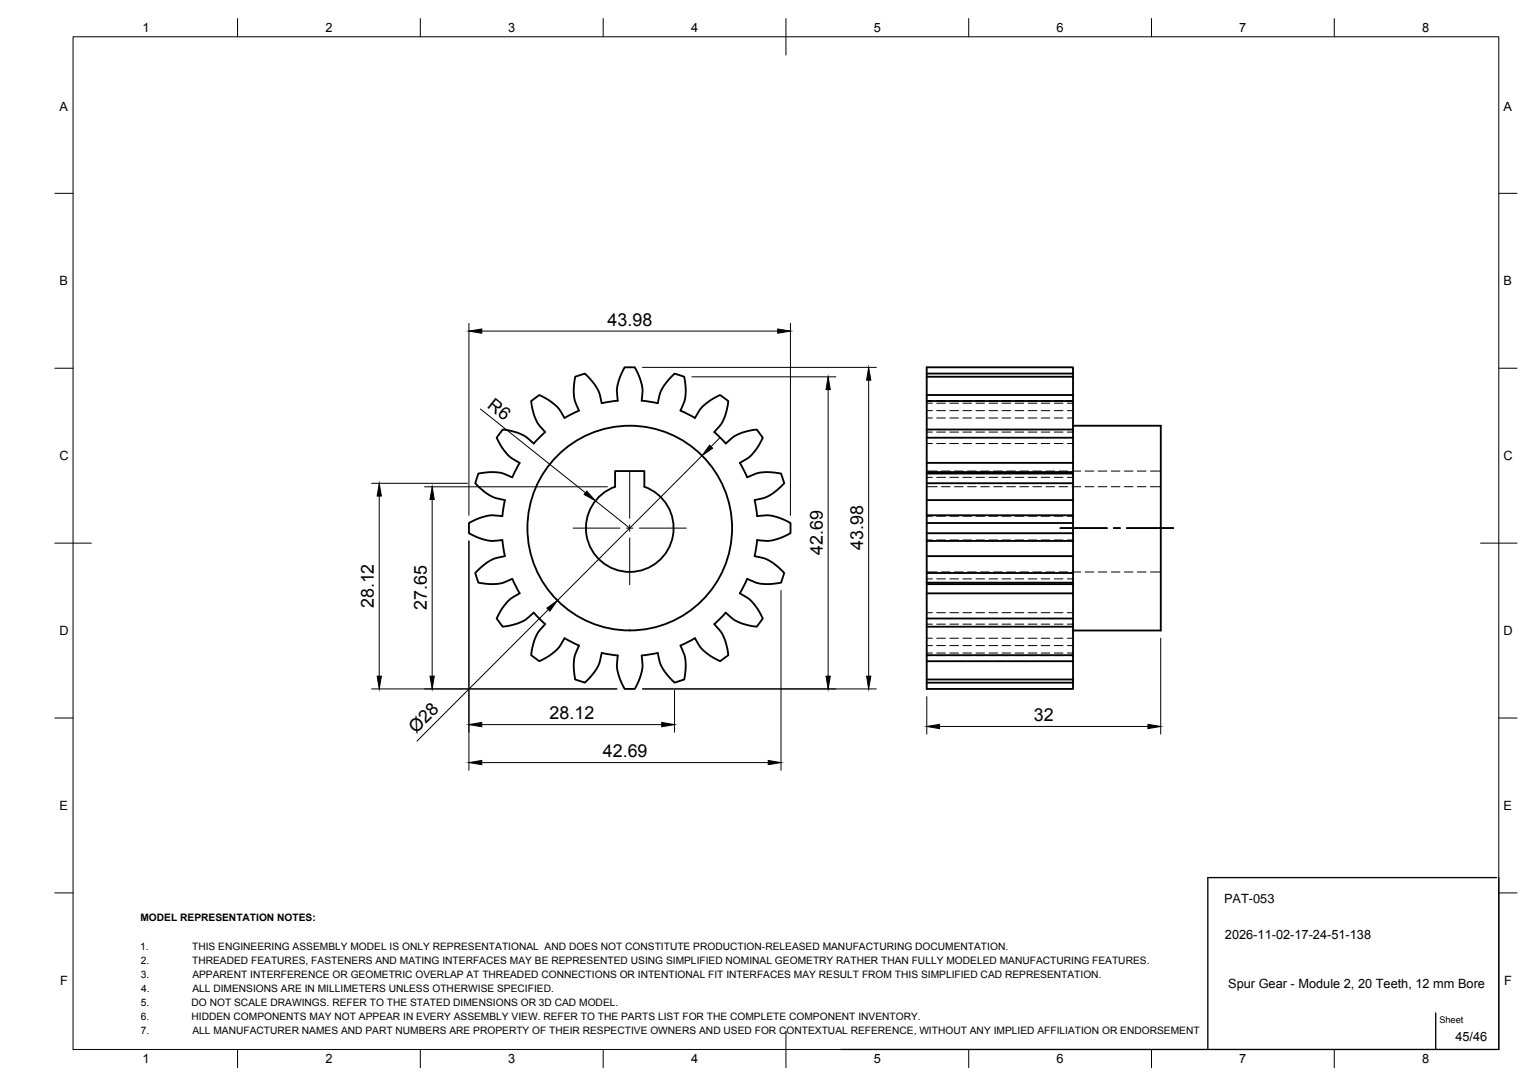
ISO-10303-21;
HEADER;
/* Generated by software containing ST-Developer
 * from STEP Tools, Inc. (www.steptools.com) 
 */

FILE_DESCRIPTION(
/* description */ ('Hand-operated arbor press'),
/* implementation_level */ '2;1');

FILE_NAME(
/* name */ 'Spur Gear - Module 2, 20 Teeth, 12 mm Bore.step',
/* time_stamp */ '2026-10-28T03:25:25-07:00',
/* author */ (''),
/* organization */ (''),
/* preprocessor_version */ 'ST-DEVELOPER v20.2',
/* originating_system */ 'Autodesk Translation Framework v15.17.0.0',
/* authorisation */ '');

FILE_SCHEMA (('AUTOMOTIVE_DESIGN { 1 0 10303 214 3 1 1 }'));
ENDSEC;

DATA;
#10=MECHANICAL_DESIGN_GEOMETRIC_PRESENTATION_REPRESENTATION('',(#630),#32751);
#11=(
BOUNDED_SURFACE()
B_SPLINE_SURFACE(5,1,((#23774,#23775),(#23776,#23777),(#23778,#23779),(#23780,
#23781),(#23782,#23783),(#23784,#23785),(#23786,#23787),(#23788,#23789),
(#23790,#23791),(#23792,#23793),(#23794,#23795),(#23796,#23797),(#23798,
#23799),(#23800,#23801),(#23802,#23803),(#23804,#23805),(#23806,#23807),
(#23808,#23809),(#23810,#23811),(#23812,#23813),(#23814,#23815),(#23816,
#23817),(#23818,#23819),(#23820,#23821),(#23822,#23823),(#23824,#23825),
(#23826,#23827),(#23828,#23829),(#23830,#23831),(#23832,#23833),(#23834,
#23835),(#23836,#23837),(#23838,#23839),(#23840,#23841),(#23842,#23843),
(#23844,#23845),(#23846,#23847),(#23848,#23849),(#23850,#23851),(#23852,
#23853),(#23854,#23855),(#23856,#23857),(#23858,#23859),(#23860,#23861),
(#23862,#23863),(#23864,#23865),(#23866,#23867),(#23868,#23869),(#23870,
#23871),(#23872,#23873),(#23874,#23875),(#23876,#23877),(#23878,#23879),
(#23880,#23881),(#23882,#23883),(#23884,#23885),(#23886,#23887),(#23888,
#23889),(#23890,#23891),(#23892,#23893),(#23894,#23895),(#23896,#23897),
(#23898,#23899),(#23900,#23901),(#23902,#23903),(#23904,#23905),(#23906,
#23907),(#23908,#23909),(#23910,#23911),(#23912,#23913)),.UNSPECIFIED.,
 .F.,.F.,.F.)
B_SPLINE_SURFACE_WITH_KNOTS((6,1,1,1,1,1,1,1,1,1,1,1,1,1,1,1,1,1,1,1,1,
1,1,1,1,1,1,1,1,1,1,1,1,1,1,1,1,1,1,1,1,1,1,1,1,1,1,1,1,1,1,1,1,1,1,1,1,
1,1,1,1,1,1,1,1,6),(2,2),(-1.,-0.984615384615383,-0.969230769230768,-0.953846153846152,
-0.938461538461537,-0.923076923076922,-0.907692307692306,-0.892307692307691,
-0.876923076923076,-0.86153846153846,-0.846153846153845,-0.83076923076923,
-0.815384615384614,-0.799999999999999,-0.784615384615384,-0.769230769230768,
-0.753846153846153,-0.738461538461538,-0.723076923076922,-0.707692307692307,
-0.692307692307692,-0.676923076923076,-0.661538461538461,-0.646153846153846,
-0.63076923076923,-0.615384615384615,-0.6,-0.584615384615384,-0.569230769230769,
-0.553846153846154,-0.538461538461538,-0.523076923076923,-0.507692307692308,
-0.492307692307692,-0.476923076923077,-0.461538461538462,-0.446153846153846,
-0.430769230769231,-0.415384615384615,-0.4,-0.384615384615385,-0.369230769230769,
-0.353846153846154,-0.338461538461538,-0.323076923076923,-0.307692307692308,
-0.292307692307692,-0.276923076923077,-0.261538461538462,-0.246153846153846,
-0.230769230769231,-0.215384615384615,-0.2,-0.184615384615385,-0.169230769230769,
-0.153846153846154,-0.138461538461538,-0.123076923076923,-0.107692307692308,
-0.0923076923076923,-0.0769230769230769,-0.0615384615384615,-0.0461538461538462,
-0.0307692307692308,-0.0153846153846154,0.),(-1.,1.),.UNSPECIFIED.)
GEOMETRIC_REPRESENTATION_ITEM()
RATIONAL_B_SPLINE_SURFACE(((1.,1.),(1.,1.),(1.,1.),(1.,1.),(1.,1.),(1.,
1.),(1.,1.),(1.,1.),(1.,1.),(1.,1.),(1.,1.),(1.,1.),(1.,1.),(1.,1.),(1.,
1.),(1.,1.),(1.,1.),(1.,1.),(1.,1.),(1.,1.),(1.,1.),(1.,1.),(1.,1.),(1.,
1.),(1.,1.),(1.,1.),(1.,1.),(1.,1.),(1.,1.),(1.,1.),(1.,1.),(1.,1.),(1.,
1.),(1.,1.),(1.,1.),(1.,1.),(1.,1.),(1.,1.),(1.,1.),(1.,1.),(1.,1.),(1.,
1.),(1.,1.),(1.,1.),(1.,1.),(1.,1.),(1.,1.),(1.,1.),(1.,1.),(1.,1.),(1.,
1.),(1.,1.),(1.,1.),(1.,1.),(1.,1.),(1.,1.),(1.,1.),(1.,1.),(1.,1.),(1.,
1.),(1.,1.),(1.,1.),(1.,1.),(1.,1.),(1.,1.),(1.,1.),(1.,1.),(1.,1.),(1.,
1.),(1.,1.)))
REPRESENTATION_ITEM('')
SURFACE()
);
#12=(
BOUNDED_SURFACE()
B_SPLINE_SURFACE(5,1,((#23992,#23993),(#23994,#23995),(#23996,#23997),(#23998,
#23999),(#24000,#24001),(#24002,#24003),(#24004,#24005),(#24006,#24007),
(#24008,#24009),(#24010,#24011),(#24012,#24013),(#24014,#24015),(#24016,
#24017),(#24018,#24019),(#24020,#24021),(#24022,#24023),(#24024,#24025),
(#24026,#24027),(#24028,#24029),(#24030,#24031),(#24032,#24033),(#24034,
#24035),(#24036,#24037),(#24038,#24039),(#24040,#24041),(#24042,#24043),
(#24044,#24045),(#24046,#24047),(#24048,#24049),(#24050,#24051),(#24052,
#24053),(#24054,#24055),(#24056,#24057),(#24058,#24059),(#24060,#24061),
(#24062,#24063),(#24064,#24065),(#24066,#24067),(#24068,#24069),(#24070,
#24071),(#24072,#24073),(#24074,#24075),(#24076,#24077),(#24078,#24079),
(#24080,#24081),(#24082,#24083),(#24084,#24085),(#24086,#24087),(#24088,
#24089),(#24090,#24091),(#24092,#24093),(#24094,#24095),(#24096,#24097),
(#24098,#24099),(#24100,#24101),(#24102,#24103),(#24104,#24105),(#24106,
#24107),(#24108,#24109),(#24110,#24111),(#24112,#24113),(#24114,#24115),
(#24116,#24117),(#24118,#24119),(#24120,#24121),(#24122,#24123),(#24124,
#24125),(#24126,#24127),(#24128,#24129),(#24130,#24131)),.UNSPECIFIED.,
 .F.,.F.,.F.)
B_SPLINE_SURFACE_WITH_KNOTS((6,1,1,1,1,1,1,1,1,1,1,1,1,1,1,1,1,1,1,1,1,
1,1,1,1,1,1,1,1,1,1,1,1,1,1,1,1,1,1,1,1,1,1,1,1,1,1,1,1,1,1,1,1,1,1,1,1,
1,1,1,1,1,1,1,1,6),(2,2),(-1.,-0.984615384615383,-0.969230769230768,-0.953846153846152,
-0.938461538461537,-0.923076923076922,-0.907692307692306,-0.892307692307691,
-0.876923076923076,-0.86153846153846,-0.846153846153845,-0.83076923076923,
-0.815384615384614,-0.799999999999999,-0.784615384615384,-0.769230769230768,
-0.753846153846153,-0.738461538461538,-0.723076923076922,-0.707692307692307,
-0.692307692307692,-0.676923076923076,-0.661538461538461,-0.646153846153846,
-0.63076923076923,-0.615384615384615,-0.6,-0.584615384615384,-0.569230769230769,
-0.553846153846154,-0.538461538461538,-0.523076923076923,-0.507692307692308,
-0.492307692307692,-0.476923076923077,-0.461538461538462,-0.446153846153846,
-0.430769230769231,-0.415384615384615,-0.4,-0.384615384615385,-0.369230769230769,
-0.353846153846154,-0.338461538461538,-0.323076923076923,-0.307692307692308,
-0.292307692307692,-0.276923076923077,-0.261538461538462,-0.246153846153846,
-0.230769230769231,-0.215384615384615,-0.2,-0.184615384615385,-0.169230769230769,
-0.153846153846154,-0.138461538461538,-0.123076923076923,-0.107692307692308,
-0.0923076923076923,-0.0769230769230769,-0.0615384615384615,-0.0461538461538462,
-0.0307692307692308,-0.0153846153846154,0.),(-1.,1.),.UNSPECIFIED.)
GEOMETRIC_REPRESENTATION_ITEM()
RATIONAL_B_SPLINE_SURFACE(((1.,1.),(1.,1.),(1.,1.),(1.,1.),(1.,1.),(1.,
1.),(1.,1.),(1.,1.),(1.,1.),(1.,1.),(1.,1.),(1.,1.),(1.,1.),(1.,1.),(1.,
1.),(1.,1.),(1.,1.),(1.,1.),(1.,1.),(1.,1.),(1.,1.),(1.,1.),(1.,1.),(1.,
1.),(1.,1.),(1.,1.),(1.,1.),(1.,1.),(1.,1.),(1.,1.),(1.,1.),(1.,1.),(1.,
1.),(1.,1.),(1.,1.),(1.,1.),(1.,1.),(1.,1.),(1.,1.),(1.,1.),(1.,1.),(1.,
1.),(1.,1.),(1.,1.),(1.,1.),(1.,1.),(1.,1.),(1.,1.),(1.,1.),(1.,1.),(1.,
1.),(1.,1.),(1.,1.),(1.,1.),(1.,1.),(1.,1.),(1.,1.),(1.,1.),(1.,1.),(1.,
1.),(1.,1.),(1.,1.),(1.,1.),(1.,1.),(1.,1.),(1.,1.),(1.,1.),(1.,1.),(1.,
1.),(1.,1.)))
REPRESENTATION_ITEM('')
SURFACE()
);
#13=(
BOUNDED_SURFACE()
B_SPLINE_SURFACE(5,1,((#24208,#24209),(#24210,#24211),(#24212,#24213),(#24214,
#24215),(#24216,#24217),(#24218,#24219),(#24220,#24221),(#24222,#24223),
(#24224,#24225),(#24226,#24227),(#24228,#24229),(#24230,#24231),(#24232,
#24233),(#24234,#24235),(#24236,#24237),(#24238,#24239),(#24240,#24241),
(#24242,#24243),(#24244,#24245),(#24246,#24247),(#24248,#24249),(#24250,
#24251),(#24252,#24253),(#24254,#24255),(#24256,#24257),(#24258,#24259),
(#24260,#24261),(#24262,#24263),(#24264,#24265),(#24266,#24267),(#24268,
#24269),(#24270,#24271),(#24272,#24273),(#24274,#24275),(#24276,#24277),
(#24278,#24279),(#24280,#24281),(#24282,#24283),(#24284,#24285),(#24286,
#24287),(#24288,#24289),(#24290,#24291),(#24292,#24293),(#24294,#24295),
(#24296,#24297),(#24298,#24299),(#24300,#24301),(#24302,#24303),(#24304,
#24305),(#24306,#24307),(#24308,#24309),(#24310,#24311),(#24312,#24313),
(#24314,#24315),(#24316,#24317),(#24318,#24319),(#24320,#24321),(#24322,
#24323),(#24324,#24325),(#24326,#24327),(#24328,#24329),(#24330,#24331),
(#24332,#24333),(#24334,#24335),(#24336,#24337),(#24338,#24339),(#24340,
#24341),(#24342,#24343),(#24344,#24345),(#24346,#24347)),.UNSPECIFIED.,
 .F.,.F.,.F.)
B_SPLINE_SURFACE_WITH_KNOTS((6,1,1,1,1,1,1,1,1,1,1,1,1,1,1,1,1,1,1,1,1,
1,1,1,1,1,1,1,1,1,1,1,1,1,1,1,1,1,1,1,1,1,1,1,1,1,1,1,1,1,1,1,1,1,1,1,1,
1,1,1,1,1,1,1,1,6),(2,2),(-1.,-0.984615384615383,-0.969230769230768,-0.953846153846152,
-0.938461538461537,-0.923076923076922,-0.907692307692306,-0.892307692307691,
-0.876923076923076,-0.86153846153846,-0.846153846153845,-0.83076923076923,
-0.815384615384614,-0.799999999999999,-0.784615384615384,-0.769230769230768,
-0.753846153846153,-0.738461538461538,-0.723076923076922,-0.707692307692307,
-0.692307692307692,-0.676923076923076,-0.661538461538461,-0.646153846153846,
-0.63076923076923,-0.615384615384615,-0.6,-0.584615384615384,-0.569230769230769,
-0.553846153846154,-0.538461538461538,-0.523076923076923,-0.507692307692308,
-0.492307692307692,-0.476923076923077,-0.461538461538462,-0.446153846153846,
-0.430769230769231,-0.415384615384615,-0.4,-0.384615384615385,-0.369230769230769,
-0.353846153846154,-0.338461538461538,-0.323076923076923,-0.307692307692308,
-0.292307692307692,-0.276923076923077,-0.261538461538462,-0.246153846153846,
-0.230769230769231,-0.215384615384615,-0.2,-0.184615384615385,-0.169230769230769,
-0.153846153846154,-0.138461538461538,-0.123076923076923,-0.107692307692308,
-0.0923076923076923,-0.0769230769230769,-0.0615384615384615,-0.0461538461538462,
-0.0307692307692308,-0.0153846153846154,0.),(-1.,1.),.UNSPECIFIED.)
GEOMETRIC_REPRESENTATION_ITEM()
RATIONAL_B_SPLINE_SURFACE(((1.,1.),(1.,1.),(1.,1.),(1.,1.),(1.,1.),(1.,
1.),(1.,1.),(1.,1.),(1.,1.),(1.,1.),(1.,1.),(1.,1.),(1.,1.),(1.,1.),(1.,
1.),(1.,1.),(1.,1.),(1.,1.),(1.,1.),(1.,1.),(1.,1.),(1.,1.),(1.,1.),(1.,
1.),(1.,1.),(1.,1.),(1.,1.),(1.,1.),(1.,1.),(1.,1.),(1.,1.),(1.,1.),(1.,
1.),(1.,1.),(1.,1.),(1.,1.),(1.,1.),(1.,1.),(1.,1.),(1.,1.),(1.,1.),(1.,
1.),(1.,1.),(1.,1.),(1.,1.),(1.,1.),(1.,1.),(1.,1.),(1.,1.),(1.,1.),(1.,
1.),(1.,1.),(1.,1.),(1.,1.),(1.,1.),(1.,1.),(1.,1.),(1.,1.),(1.,1.),(1.,
1.),(1.,1.),(1.,1.),(1.,1.),(1.,1.),(1.,1.),(1.,1.),(1.,1.),(1.,1.),(1.,
1.),(1.,1.)))
REPRESENTATION_ITEM('')
SURFACE()
);
#14=(
BOUNDED_SURFACE()
B_SPLINE_SURFACE(5,1,((#24424,#24425),(#24426,#24427),(#24428,#24429),(#24430,
#24431),(#24432,#24433),(#24434,#24435),(#24436,#24437),(#24438,#24439),
(#24440,#24441),(#24442,#24443),(#24444,#24445),(#24446,#24447),(#24448,
#24449),(#24450,#24451),(#24452,#24453),(#24454,#24455),(#24456,#24457),
(#24458,#24459),(#24460,#24461),(#24462,#24463),(#24464,#24465),(#24466,
#24467),(#24468,#24469),(#24470,#24471),(#24472,#24473),(#24474,#24475),
(#24476,#24477),(#24478,#24479),(#24480,#24481),(#24482,#24483),(#24484,
#24485),(#24486,#24487),(#24488,#24489),(#24490,#24491),(#24492,#24493),
(#24494,#24495),(#24496,#24497),(#24498,#24499),(#24500,#24501),(#24502,
#24503),(#24504,#24505),(#24506,#24507),(#24508,#24509),(#24510,#24511),
(#24512,#24513),(#24514,#24515),(#24516,#24517),(#24518,#24519),(#24520,
#24521),(#24522,#24523),(#24524,#24525),(#24526,#24527),(#24528,#24529),
(#24530,#24531),(#24532,#24533),(#24534,#24535),(#24536,#24537),(#24538,
#24539),(#24540,#24541),(#24542,#24543),(#24544,#24545),(#24546,#24547),
(#24548,#24549),(#24550,#24551),(#24552,#24553),(#24554,#24555),(#24556,
#24557),(#24558,#24559),(#24560,#24561),(#24562,#24563)),.UNSPECIFIED.,
 .F.,.F.,.F.)
B_SPLINE_SURFACE_WITH_KNOTS((6,1,1,1,1,1,1,1,1,1,1,1,1,1,1,1,1,1,1,1,1,
1,1,1,1,1,1,1,1,1,1,1,1,1,1,1,1,1,1,1,1,1,1,1,1,1,1,1,1,1,1,1,1,1,1,1,1,
1,1,1,1,1,1,1,1,6),(2,2),(-1.,-0.984615384615383,-0.969230769230768,-0.953846153846152,
-0.938461538461537,-0.923076923076922,-0.907692307692306,-0.892307692307691,
-0.876923076923076,-0.86153846153846,-0.846153846153845,-0.83076923076923,
-0.815384615384614,-0.799999999999999,-0.784615384615384,-0.769230769230768,
-0.753846153846153,-0.738461538461538,-0.723076923076922,-0.707692307692307,
-0.692307692307692,-0.676923076923076,-0.661538461538461,-0.646153846153846,
-0.63076923076923,-0.615384615384615,-0.6,-0.584615384615384,-0.569230769230769,
-0.553846153846154,-0.538461538461538,-0.523076923076923,-0.507692307692308,
-0.492307692307692,-0.476923076923077,-0.461538461538462,-0.446153846153846,
-0.430769230769231,-0.415384615384615,-0.4,-0.384615384615385,-0.369230769230769,
-0.353846153846154,-0.338461538461538,-0.323076923076923,-0.307692307692308,
-0.292307692307692,-0.276923076923077,-0.261538461538462,-0.246153846153846,
-0.230769230769231,-0.215384615384615,-0.2,-0.184615384615385,-0.169230769230769,
-0.153846153846154,-0.138461538461538,-0.123076923076923,-0.107692307692308,
-0.0923076923076923,-0.0769230769230769,-0.0615384615384615,-0.0461538461538462,
-0.0307692307692308,-0.0153846153846154,0.),(-1.,1.),.UNSPECIFIED.)
GEOMETRIC_REPRESENTATION_ITEM()
RATIONAL_B_SPLINE_SURFACE(((1.,1.),(1.,1.),(1.,1.),(1.,1.),(1.,1.),(1.,
1.),(1.,1.),(1.,1.),(1.,1.),(1.,1.),(1.,1.),(1.,1.),(1.,1.),(1.,1.),(1.,
1.),(1.,1.),(1.,1.),(1.,1.),(1.,1.),(1.,1.),(1.,1.),(1.,1.),(1.,1.),(1.,
1.),(1.,1.),(1.,1.),(1.,1.),(1.,1.),(1.,1.),(1.,1.),(1.,1.),(1.,1.),(1.,
1.),(1.,1.),(1.,1.),(1.,1.),(1.,1.),(1.,1.),(1.,1.),(1.,1.),(1.,1.),(1.,
1.),(1.,1.),(1.,1.),(1.,1.),(1.,1.),(1.,1.),(1.,1.),(1.,1.),(1.,1.),(1.,
1.),(1.,1.),(1.,1.),(1.,1.),(1.,1.),(1.,1.),(1.,1.),(1.,1.),(1.,1.),(1.,
1.),(1.,1.),(1.,1.),(1.,1.),(1.,1.),(1.,1.),(1.,1.),(1.,1.),(1.,1.),(1.,
1.),(1.,1.)))
REPRESENTATION_ITEM('')
SURFACE()
);
#15=(
BOUNDED_SURFACE()
B_SPLINE_SURFACE(5,1,((#24640,#24641),(#24642,#24643),(#24644,#24645),(#24646,
#24647),(#24648,#24649),(#24650,#24651),(#24652,#24653),(#24654,#24655),
(#24656,#24657),(#24658,#24659),(#24660,#24661),(#24662,#24663),(#24664,
#24665),(#24666,#24667),(#24668,#24669),(#24670,#24671),(#24672,#24673),
(#24674,#24675),(#24676,#24677),(#24678,#24679),(#24680,#24681),(#24682,
#24683),(#24684,#24685),(#24686,#24687),(#24688,#24689),(#24690,#24691),
(#24692,#24693),(#24694,#24695),(#24696,#24697),(#24698,#24699),(#24700,
#24701),(#24702,#24703),(#24704,#24705),(#24706,#24707),(#24708,#24709),
(#24710,#24711),(#24712,#24713),(#24714,#24715),(#24716,#24717),(#24718,
#24719),(#24720,#24721),(#24722,#24723),(#24724,#24725),(#24726,#24727),
(#24728,#24729),(#24730,#24731),(#24732,#24733),(#24734,#24735),(#24736,
#24737),(#24738,#24739),(#24740,#24741),(#24742,#24743),(#24744,#24745),
(#24746,#24747),(#24748,#24749),(#24750,#24751),(#24752,#24753),(#24754,
#24755),(#24756,#24757),(#24758,#24759),(#24760,#24761),(#24762,#24763),
(#24764,#24765),(#24766,#24767),(#24768,#24769),(#24770,#24771),(#24772,
#24773),(#24774,#24775),(#24776,#24777),(#24778,#24779)),.UNSPECIFIED.,
 .F.,.F.,.F.)
B_SPLINE_SURFACE_WITH_KNOTS((6,1,1,1,1,1,1,1,1,1,1,1,1,1,1,1,1,1,1,1,1,
1,1,1,1,1,1,1,1,1,1,1,1,1,1,1,1,1,1,1,1,1,1,1,1,1,1,1,1,1,1,1,1,1,1,1,1,
1,1,1,1,1,1,1,1,6),(2,2),(-1.,-0.984615384615383,-0.969230769230768,-0.953846153846152,
-0.938461538461537,-0.923076923076922,-0.907692307692306,-0.892307692307691,
-0.876923076923076,-0.86153846153846,-0.846153846153845,-0.83076923076923,
-0.815384615384614,-0.799999999999999,-0.784615384615384,-0.769230769230768,
-0.753846153846153,-0.738461538461538,-0.723076923076922,-0.707692307692307,
-0.692307692307692,-0.676923076923076,-0.661538461538461,-0.646153846153846,
-0.63076923076923,-0.615384615384615,-0.6,-0.584615384615384,-0.569230769230769,
-0.553846153846154,-0.538461538461538,-0.523076923076923,-0.507692307692308,
-0.492307692307692,-0.476923076923077,-0.461538461538462,-0.446153846153846,
-0.430769230769231,-0.415384615384615,-0.4,-0.384615384615385,-0.369230769230769,
-0.353846153846154,-0.338461538461538,-0.323076923076923,-0.307692307692308,
-0.292307692307692,-0.276923076923077,-0.261538461538462,-0.246153846153846,
-0.230769230769231,-0.215384615384615,-0.2,-0.184615384615385,-0.169230769230769,
-0.153846153846154,-0.138461538461538,-0.123076923076923,-0.107692307692308,
-0.0923076923076923,-0.0769230769230769,-0.0615384615384615,-0.0461538461538462,
-0.0307692307692308,-0.0153846153846154,0.),(-1.,1.),.UNSPECIFIED.)
GEOMETRIC_REPRESENTATION_ITEM()
RATIONAL_B_SPLINE_SURFACE(((1.,1.),(1.,1.),(1.,1.),(1.,1.),(1.,1.),(1.,
1.),(1.,1.),(1.,1.),(1.,1.),(1.,1.),(1.,1.),(1.,1.),(1.,1.),(1.,1.),(1.,
1.),(1.,1.),(1.,1.),(1.,1.),(1.,1.),(1.,1.),(1.,1.),(1.,1.),(1.,1.),(1.,
1.),(1.,1.),(1.,1.),(1.,1.),(1.,1.),(1.,1.),(1.,1.),(1.,1.),(1.,1.),(1.,
1.),(1.,1.),(1.,1.),(1.,1.),(1.,1.),(1.,1.),(1.,1.),(1.,1.),(1.,1.),(1.,
1.),(1.,1.),(1.,1.),(1.,1.),(1.,1.),(1.,1.),(1.,1.),(1.,1.),(1.,1.),(1.,
1.),(1.,1.),(1.,1.),(1.,1.),(1.,1.),(1.,1.),(1.,1.),(1.,1.),(1.,1.),(1.,
1.),(1.,1.),(1.,1.),(1.,1.),(1.,1.),(1.,1.),(1.,1.),(1.,1.),(1.,1.),(1.,
1.),(1.,1.)))
REPRESENTATION_ITEM('')
SURFACE()
);
#16=(
BOUNDED_SURFACE()
B_SPLINE_SURFACE(5,1,((#24856,#24857),(#24858,#24859),(#24860,#24861),(#24862,
#24863),(#24864,#24865),(#24866,#24867),(#24868,#24869),(#24870,#24871),
(#24872,#24873),(#24874,#24875),(#24876,#24877),(#24878,#24879),(#24880,
#24881),(#24882,#24883),(#24884,#24885),(#24886,#24887),(#24888,#24889),
(#24890,#24891),(#24892,#24893),(#24894,#24895),(#24896,#24897),(#24898,
#24899),(#24900,#24901),(#24902,#24903),(#24904,#24905),(#24906,#24907),
(#24908,#24909),(#24910,#24911),(#24912,#24913),(#24914,#24915),(#24916,
#24917),(#24918,#24919),(#24920,#24921),(#24922,#24923),(#24924,#24925),
(#24926,#24927),(#24928,#24929),(#24930,#24931),(#24932,#24933),(#24934,
#24935),(#24936,#24937),(#24938,#24939),(#24940,#24941),(#24942,#24943),
(#24944,#24945),(#24946,#24947),(#24948,#24949),(#24950,#24951),(#24952,
#24953),(#24954,#24955),(#24956,#24957),(#24958,#24959),(#24960,#24961),
(#24962,#24963),(#24964,#24965),(#24966,#24967),(#24968,#24969),(#24970,
#24971),(#24972,#24973),(#24974,#24975),(#24976,#24977),(#24978,#24979),
(#24980,#24981),(#24982,#24983),(#24984,#24985),(#24986,#24987),(#24988,
#24989),(#24990,#24991),(#24992,#24993),(#24994,#24995)),.UNSPECIFIED.,
 .F.,.F.,.F.)
B_SPLINE_SURFACE_WITH_KNOTS((6,1,1,1,1,1,1,1,1,1,1,1,1,1,1,1,1,1,1,1,1,
1,1,1,1,1,1,1,1,1,1,1,1,1,1,1,1,1,1,1,1,1,1,1,1,1,1,1,1,1,1,1,1,1,1,1,1,
1,1,1,1,1,1,1,1,6),(2,2),(-1.,-0.984615384615383,-0.969230769230768,-0.953846153846152,
-0.938461538461537,-0.923076923076922,-0.907692307692306,-0.892307692307691,
-0.876923076923076,-0.86153846153846,-0.846153846153845,-0.83076923076923,
-0.815384615384614,-0.799999999999999,-0.784615384615384,-0.769230769230768,
-0.753846153846153,-0.738461538461538,-0.723076923076922,-0.707692307692307,
-0.692307692307692,-0.676923076923076,-0.661538461538461,-0.646153846153846,
-0.63076923076923,-0.615384615384615,-0.6,-0.584615384615384,-0.569230769230769,
-0.553846153846154,-0.538461538461538,-0.523076923076923,-0.507692307692308,
-0.492307692307692,-0.476923076923077,-0.461538461538462,-0.446153846153846,
-0.430769230769231,-0.415384615384615,-0.4,-0.384615384615385,-0.369230769230769,
-0.353846153846154,-0.338461538461538,-0.323076923076923,-0.307692307692308,
-0.292307692307692,-0.276923076923077,-0.261538461538462,-0.246153846153846,
-0.230769230769231,-0.215384615384615,-0.2,-0.184615384615385,-0.169230769230769,
-0.153846153846154,-0.138461538461538,-0.123076923076923,-0.107692307692308,
-0.0923076923076923,-0.0769230769230769,-0.0615384615384615,-0.0461538461538462,
-0.0307692307692308,-0.0153846153846154,0.),(-1.,1.),.UNSPECIFIED.)
GEOMETRIC_REPRESENTATION_ITEM()
RATIONAL_B_SPLINE_SURFACE(((1.,1.),(1.,1.),(1.,1.),(1.,1.),(1.,1.),(1.,
1.),(1.,1.),(1.,1.),(1.,1.),(1.,1.),(1.,1.),(1.,1.),(1.,1.),(1.,1.),(1.,
1.),(1.,1.),(1.,1.),(1.,1.),(1.,1.),(1.,1.),(1.,1.),(1.,1.),(1.,1.),(1.,
1.),(1.,1.),(1.,1.),(1.,1.),(1.,1.),(1.,1.),(1.,1.),(1.,1.),(1.,1.),(1.,
1.),(1.,1.),(1.,1.),(1.,1.),(1.,1.),(1.,1.),(1.,1.),(1.,1.),(1.,1.),(1.,
1.),(1.,1.),(1.,1.),(1.,1.),(1.,1.),(1.,1.),(1.,1.),(1.,1.),(1.,1.),(1.,
1.),(1.,1.),(1.,1.),(1.,1.),(1.,1.),(1.,1.),(1.,1.),(1.,1.),(1.,1.),(1.,
1.),(1.,1.),(1.,1.),(1.,1.),(1.,1.),(1.,1.),(1.,1.),(1.,1.),(1.,1.),(1.,
1.),(1.,1.)))
REPRESENTATION_ITEM('')
SURFACE()
);
#17=(
BOUNDED_SURFACE()
B_SPLINE_SURFACE(5,1,((#25072,#25073),(#25074,#25075),(#25076,#25077),(#25078,
#25079),(#25080,#25081),(#25082,#25083),(#25084,#25085),(#25086,#25087),
(#25088,#25089),(#25090,#25091),(#25092,#25093),(#25094,#25095),(#25096,
#25097),(#25098,#25099),(#25100,#25101),(#25102,#25103),(#25104,#25105),
(#25106,#25107),(#25108,#25109),(#25110,#25111),(#25112,#25113),(#25114,
#25115),(#25116,#25117),(#25118,#25119),(#25120,#25121),(#25122,#25123),
(#25124,#25125),(#25126,#25127),(#25128,#25129),(#25130,#25131),(#25132,
#25133),(#25134,#25135),(#25136,#25137),(#25138,#25139),(#25140,#25141),
(#25142,#25143),(#25144,#25145),(#25146,#25147),(#25148,#25149),(#25150,
#25151),(#25152,#25153),(#25154,#25155),(#25156,#25157),(#25158,#25159),
(#25160,#25161),(#25162,#25163),(#25164,#25165),(#25166,#25167),(#25168,
#25169),(#25170,#25171),(#25172,#25173),(#25174,#25175),(#25176,#25177),
(#25178,#25179),(#25180,#25181),(#25182,#25183),(#25184,#25185),(#25186,
#25187),(#25188,#25189),(#25190,#25191),(#25192,#25193),(#25194,#25195),
(#25196,#25197),(#25198,#25199),(#25200,#25201),(#25202,#25203),(#25204,
#25205),(#25206,#25207),(#25208,#25209),(#25210,#25211)),.UNSPECIFIED.,
 .F.,.F.,.F.)
B_SPLINE_SURFACE_WITH_KNOTS((6,1,1,1,1,1,1,1,1,1,1,1,1,1,1,1,1,1,1,1,1,
1,1,1,1,1,1,1,1,1,1,1,1,1,1,1,1,1,1,1,1,1,1,1,1,1,1,1,1,1,1,1,1,1,1,1,1,
1,1,1,1,1,1,1,1,6),(2,2),(-1.,-0.984615384615383,-0.969230769230768,-0.953846153846152,
-0.938461538461537,-0.923076923076922,-0.907692307692306,-0.892307692307691,
-0.876923076923076,-0.86153846153846,-0.846153846153845,-0.83076923076923,
-0.815384615384614,-0.799999999999999,-0.784615384615384,-0.769230769230768,
-0.753846153846153,-0.738461538461538,-0.723076923076922,-0.707692307692307,
-0.692307692307692,-0.676923076923076,-0.661538461538461,-0.646153846153846,
-0.63076923076923,-0.615384615384615,-0.6,-0.584615384615384,-0.569230769230769,
-0.553846153846154,-0.538461538461538,-0.523076923076923,-0.507692307692308,
-0.492307692307692,-0.476923076923077,-0.461538461538462,-0.446153846153846,
-0.430769230769231,-0.415384615384615,-0.4,-0.384615384615385,-0.369230769230769,
-0.353846153846154,-0.338461538461538,-0.323076923076923,-0.307692307692308,
-0.292307692307692,-0.276923076923077,-0.261538461538462,-0.246153846153846,
-0.230769230769231,-0.215384615384615,-0.2,-0.184615384615385,-0.169230769230769,
-0.153846153846154,-0.138461538461538,-0.123076923076923,-0.107692307692308,
-0.0923076923076923,-0.0769230769230769,-0.0615384615384615,-0.0461538461538462,
-0.0307692307692308,-0.0153846153846154,0.),(-1.,1.),.UNSPECIFIED.)
GEOMETRIC_REPRESENTATION_ITEM()
RATIONAL_B_SPLINE_SURFACE(((1.,1.),(1.,1.),(1.,1.),(1.,1.),(1.,1.),(1.,
1.),(1.,1.),(1.,1.),(1.,1.),(1.,1.),(1.,1.),(1.,1.),(1.,1.),(1.,1.),(1.,
1.),(1.,1.),(1.,1.),(1.,1.),(1.,1.),(1.,1.),(1.,1.),(1.,1.),(1.,1.),(1.,
1.),(1.,1.),(1.,1.),(1.,1.),(1.,1.),(1.,1.),(1.,1.),(1.,1.),(1.,1.),(1.,
1.),(1.,1.),(1.,1.),(1.,1.),(1.,1.),(1.,1.),(1.,1.),(1.,1.),(1.,1.),(1.,
1.),(1.,1.),(1.,1.),(1.,1.),(1.,1.),(1.,1.),(1.,1.),(1.,1.),(1.,1.),(1.,
1.),(1.,1.),(1.,1.),(1.,1.),(1.,1.),(1.,1.),(1.,1.),(1.,1.),(1.,1.),(1.,
1.),(1.,1.),(1.,1.),(1.,1.),(1.,1.),(1.,1.),(1.,1.),(1.,1.),(1.,1.),(1.,
1.),(1.,1.)))
REPRESENTATION_ITEM('')
SURFACE()
);
#18=(
BOUNDED_SURFACE()
B_SPLINE_SURFACE(5,1,((#25288,#25289),(#25290,#25291),(#25292,#25293),(#25294,
#25295),(#25296,#25297),(#25298,#25299),(#25300,#25301),(#25302,#25303),
(#25304,#25305),(#25306,#25307),(#25308,#25309),(#25310,#25311),(#25312,
#25313),(#25314,#25315),(#25316,#25317),(#25318,#25319),(#25320,#25321),
(#25322,#25323),(#25324,#25325),(#25326,#25327),(#25328,#25329),(#25330,
#25331),(#25332,#25333),(#25334,#25335),(#25336,#25337),(#25338,#25339),
(#25340,#25341),(#25342,#25343),(#25344,#25345),(#25346,#25347),(#25348,
#25349),(#25350,#25351),(#25352,#25353),(#25354,#25355),(#25356,#25357),
(#25358,#25359),(#25360,#25361),(#25362,#25363),(#25364,#25365),(#25366,
#25367),(#25368,#25369),(#25370,#25371),(#25372,#25373),(#25374,#25375),
(#25376,#25377),(#25378,#25379),(#25380,#25381),(#25382,#25383),(#25384,
#25385),(#25386,#25387),(#25388,#25389),(#25390,#25391),(#25392,#25393),
(#25394,#25395),(#25396,#25397),(#25398,#25399),(#25400,#25401),(#25402,
#25403),(#25404,#25405),(#25406,#25407),(#25408,#25409),(#25410,#25411),
(#25412,#25413),(#25414,#25415),(#25416,#25417),(#25418,#25419),(#25420,
#25421),(#25422,#25423),(#25424,#25425),(#25426,#25427)),.UNSPECIFIED.,
 .F.,.F.,.F.)
B_SPLINE_SURFACE_WITH_KNOTS((6,1,1,1,1,1,1,1,1,1,1,1,1,1,1,1,1,1,1,1,1,
1,1,1,1,1,1,1,1,1,1,1,1,1,1,1,1,1,1,1,1,1,1,1,1,1,1,1,1,1,1,1,1,1,1,1,1,
1,1,1,1,1,1,1,1,6),(2,2),(-1.,-0.984615384615383,-0.969230769230768,-0.953846153846152,
-0.938461538461537,-0.923076923076922,-0.907692307692306,-0.892307692307691,
-0.876923076923076,-0.86153846153846,-0.846153846153845,-0.83076923076923,
-0.815384615384614,-0.799999999999999,-0.784615384615384,-0.769230769230768,
-0.753846153846153,-0.738461538461538,-0.723076923076922,-0.707692307692307,
-0.692307692307692,-0.676923076923076,-0.661538461538461,-0.646153846153846,
-0.63076923076923,-0.615384615384615,-0.6,-0.584615384615384,-0.569230769230769,
-0.553846153846154,-0.538461538461538,-0.523076923076923,-0.507692307692308,
-0.492307692307692,-0.476923076923077,-0.461538461538462,-0.446153846153846,
-0.430769230769231,-0.415384615384615,-0.4,-0.384615384615385,-0.369230769230769,
-0.353846153846154,-0.338461538461538,-0.323076923076923,-0.307692307692308,
-0.292307692307692,-0.276923076923077,-0.261538461538462,-0.246153846153846,
-0.230769230769231,-0.215384615384615,-0.2,-0.184615384615385,-0.169230769230769,
-0.153846153846154,-0.138461538461538,-0.123076923076923,-0.107692307692308,
-0.0923076923076923,-0.0769230769230769,-0.0615384615384615,-0.0461538461538462,
-0.0307692307692308,-0.0153846153846154,0.),(-1.,1.),.UNSPECIFIED.)
GEOMETRIC_REPRESENTATION_ITEM()
RATIONAL_B_SPLINE_SURFACE(((1.,1.),(1.,1.),(1.,1.),(1.,1.),(1.,1.),(1.,
1.),(1.,1.),(1.,1.),(1.,1.),(1.,1.),(1.,1.),(1.,1.),(1.,1.),(1.,1.),(1.,
1.),(1.,1.),(1.,1.),(1.,1.),(1.,1.),(1.,1.),(1.,1.),(1.,1.),(1.,1.),(1.,
1.),(1.,1.),(1.,1.),(1.,1.),(1.,1.),(1.,1.),(1.,1.),(1.,1.),(1.,1.),(1.,
1.),(1.,1.),(1.,1.),(1.,1.),(1.,1.),(1.,1.),(1.,1.),(1.,1.),(1.,1.),(1.,
1.),(1.,1.),(1.,1.),(1.,1.),(1.,1.),(1.,1.),(1.,1.),(1.,1.),(1.,1.),(1.,
1.),(1.,1.),(1.,1.),(1.,1.),(1.,1.),(1.,1.),(1.,1.),(1.,1.),(1.,1.),(1.,
1.),(1.,1.),(1.,1.),(1.,1.),(1.,1.),(1.,1.),(1.,1.),(1.,1.),(1.,1.),(1.,
1.),(1.,1.)))
REPRESENTATION_ITEM('')
SURFACE()
);
#19=(
BOUNDED_SURFACE()
B_SPLINE_SURFACE(5,1,((#25504,#25505),(#25506,#25507),(#25508,#25509),(#25510,
#25511),(#25512,#25513),(#25514,#25515),(#25516,#25517),(#25518,#25519),
(#25520,#25521),(#25522,#25523),(#25524,#25525),(#25526,#25527),(#25528,
#25529),(#25530,#25531),(#25532,#25533),(#25534,#25535),(#25536,#25537),
(#25538,#25539),(#25540,#25541),(#25542,#25543),(#25544,#25545),(#25546,
#25547),(#25548,#25549),(#25550,#25551),(#25552,#25553),(#25554,#25555),
(#25556,#25557),(#25558,#25559),(#25560,#25561),(#25562,#25563),(#25564,
#25565),(#25566,#25567),(#25568,#25569),(#25570,#25571),(#25572,#25573),
(#25574,#25575),(#25576,#25577),(#25578,#25579),(#25580,#25581),(#25582,
#25583),(#25584,#25585),(#25586,#25587),(#25588,#25589),(#25590,#25591),
(#25592,#25593),(#25594,#25595),(#25596,#25597),(#25598,#25599),(#25600,
#25601),(#25602,#25603),(#25604,#25605),(#25606,#25607),(#25608,#25609),
(#25610,#25611),(#25612,#25613),(#25614,#25615),(#25616,#25617),(#25618,
#25619),(#25620,#25621),(#25622,#25623),(#25624,#25625),(#25626,#25627),
(#25628,#25629),(#25630,#25631),(#25632,#25633),(#25634,#25635),(#25636,
#25637),(#25638,#25639),(#25640,#25641),(#25642,#25643)),.UNSPECIFIED.,
 .F.,.F.,.F.)
B_SPLINE_SURFACE_WITH_KNOTS((6,1,1,1,1,1,1,1,1,1,1,1,1,1,1,1,1,1,1,1,1,
1,1,1,1,1,1,1,1,1,1,1,1,1,1,1,1,1,1,1,1,1,1,1,1,1,1,1,1,1,1,1,1,1,1,1,1,
1,1,1,1,1,1,1,1,6),(2,2),(-1.,-0.984615384615383,-0.969230769230768,-0.953846153846152,
-0.938461538461537,-0.923076923076922,-0.907692307692306,-0.892307692307691,
-0.876923076923076,-0.86153846153846,-0.846153846153845,-0.83076923076923,
-0.815384615384614,-0.799999999999999,-0.784615384615384,-0.769230769230768,
-0.753846153846153,-0.738461538461538,-0.723076923076922,-0.707692307692307,
-0.692307692307692,-0.676923076923076,-0.661538461538461,-0.646153846153846,
-0.63076923076923,-0.615384615384615,-0.6,-0.584615384615384,-0.569230769230769,
-0.553846153846154,-0.538461538461538,-0.523076923076923,-0.507692307692308,
-0.492307692307692,-0.476923076923077,-0.461538461538462,-0.446153846153846,
-0.430769230769231,-0.415384615384615,-0.4,-0.384615384615385,-0.369230769230769,
-0.353846153846154,-0.338461538461538,-0.323076923076923,-0.307692307692308,
-0.292307692307692,-0.276923076923077,-0.261538461538462,-0.246153846153846,
-0.230769230769231,-0.215384615384615,-0.2,-0.184615384615385,-0.169230769230769,
-0.153846153846154,-0.138461538461538,-0.123076923076923,-0.107692307692308,
-0.0923076923076923,-0.0769230769230769,-0.0615384615384615,-0.0461538461538462,
-0.0307692307692308,-0.0153846153846154,0.),(-1.,1.),.UNSPECIFIED.)
GEOMETRIC_REPRESENTATION_ITEM()
RATIONAL_B_SPLINE_SURFACE(((1.,1.),(1.,1.),(1.,1.),(1.,1.),(1.,1.),(1.,
1.),(1.,1.),(1.,1.),(1.,1.),(1.,1.),(1.,1.),(1.,1.),(1.,1.),(1.,1.),(1.,
1.),(1.,1.),(1.,1.),(1.,1.),(1.,1.),(1.,1.),(1.,1.),(1.,1.),(1.,1.),(1.,
1.),(1.,1.),(1.,1.),(1.,1.),(1.,1.),(1.,1.),(1.,1.),(1.,1.),(1.,1.),(1.,
1.),(1.,1.),(1.,1.),(1.,1.),(1.,1.),(1.,1.),(1.,1.),(1.,1.),(1.,1.),(1.,
1.),(1.,1.),(1.,1.),(1.,1.),(1.,1.),(1.,1.),(1.,1.),(1.,1.),(1.,1.),(1.,
1.),(1.,1.),(1.,1.),(1.,1.),(1.,1.),(1.,1.),(1.,1.),(1.,1.),(1.,1.),(1.,
1.),(1.,1.),(1.,1.),(1.,1.),(1.,1.),(1.,1.),(1.,1.),(1.,1.),(1.,1.),(1.,
1.),(1.,1.)))
REPRESENTATION_ITEM('')
SURFACE()
);
#20=(
BOUNDED_SURFACE()
B_SPLINE_SURFACE(5,1,((#25720,#25721),(#25722,#25723),(#25724,#25725),(#25726,
#25727),(#25728,#25729),(#25730,#25731),(#25732,#25733),(#25734,#25735),
(#25736,#25737),(#25738,#25739),(#25740,#25741),(#25742,#25743),(#25744,
#25745),(#25746,#25747),(#25748,#25749),(#25750,#25751),(#25752,#25753),
(#25754,#25755),(#25756,#25757),(#25758,#25759),(#25760,#25761),(#25762,
#25763),(#25764,#25765),(#25766,#25767),(#25768,#25769),(#25770,#25771),
(#25772,#25773),(#25774,#25775),(#25776,#25777),(#25778,#25779),(#25780,
#25781),(#25782,#25783),(#25784,#25785),(#25786,#25787),(#25788,#25789),
(#25790,#25791),(#25792,#25793),(#25794,#25795),(#25796,#25797),(#25798,
#25799),(#25800,#25801),(#25802,#25803),(#25804,#25805),(#25806,#25807),
(#25808,#25809),(#25810,#25811),(#25812,#25813),(#25814,#25815),(#25816,
#25817),(#25818,#25819),(#25820,#25821),(#25822,#25823),(#25824,#25825),
(#25826,#25827),(#25828,#25829),(#25830,#25831),(#25832,#25833),(#25834,
#25835),(#25836,#25837),(#25838,#25839),(#25840,#25841),(#25842,#25843),
(#25844,#25845),(#25846,#25847),(#25848,#25849),(#25850,#25851),(#25852,
#25853),(#25854,#25855),(#25856,#25857),(#25858,#25859)),.UNSPECIFIED.,
 .F.,.F.,.F.)
B_SPLINE_SURFACE_WITH_KNOTS((6,1,1,1,1,1,1,1,1,1,1,1,1,1,1,1,1,1,1,1,1,
1,1,1,1,1,1,1,1,1,1,1,1,1,1,1,1,1,1,1,1,1,1,1,1,1,1,1,1,1,1,1,1,1,1,1,1,
1,1,1,1,1,1,1,1,6),(2,2),(-1.,-0.984615384615383,-0.969230769230768,-0.953846153846152,
-0.938461538461537,-0.923076923076922,-0.907692307692306,-0.892307692307691,
-0.876923076923076,-0.86153846153846,-0.846153846153845,-0.83076923076923,
-0.815384615384614,-0.799999999999999,-0.784615384615384,-0.769230769230768,
-0.753846153846153,-0.738461538461538,-0.723076923076922,-0.707692307692307,
-0.692307692307692,-0.676923076923076,-0.661538461538461,-0.646153846153846,
-0.63076923076923,-0.615384615384615,-0.6,-0.584615384615384,-0.569230769230769,
-0.553846153846154,-0.538461538461538,-0.523076923076923,-0.507692307692308,
-0.492307692307692,-0.476923076923077,-0.461538461538462,-0.446153846153846,
-0.430769230769231,-0.415384615384615,-0.4,-0.384615384615385,-0.369230769230769,
-0.353846153846154,-0.338461538461538,-0.323076923076923,-0.307692307692308,
-0.292307692307692,-0.276923076923077,-0.261538461538462,-0.246153846153846,
-0.230769230769231,-0.215384615384615,-0.2,-0.184615384615385,-0.169230769230769,
-0.153846153846154,-0.138461538461538,-0.123076923076923,-0.107692307692308,
-0.0923076923076923,-0.0769230769230769,-0.0615384615384615,-0.0461538461538462,
-0.0307692307692308,-0.0153846153846154,0.),(-1.,1.),.UNSPECIFIED.)
GEOMETRIC_REPRESENTATION_ITEM()
RATIONAL_B_SPLINE_SURFACE(((1.,1.),(1.,1.),(1.,1.),(1.,1.),(1.,1.),(1.,
1.),(1.,1.),(1.,1.),(1.,1.),(1.,1.),(1.,1.),(1.,1.),(1.,1.),(1.,1.),(1.,
1.),(1.,1.),(1.,1.),(1.,1.),(1.,1.),(1.,1.),(1.,1.),(1.,1.),(1.,1.),(1.,
1.),(1.,1.),(1.,1.),(1.,1.),(1.,1.),(1.,1.),(1.,1.),(1.,1.),(1.,1.),(1.,
1.),(1.,1.),(1.,1.),(1.,1.),(1.,1.),(1.,1.),(1.,1.),(1.,1.),(1.,1.),(1.,
1.),(1.,1.),(1.,1.),(1.,1.),(1.,1.),(1.,1.),(1.,1.),(1.,1.),(1.,1.),(1.,
1.),(1.,1.),(1.,1.),(1.,1.),(1.,1.),(1.,1.),(1.,1.),(1.,1.),(1.,1.),(1.,
1.),(1.,1.),(1.,1.),(1.,1.),(1.,1.),(1.,1.),(1.,1.),(1.,1.),(1.,1.),(1.,
1.),(1.,1.)))
REPRESENTATION_ITEM('')
SURFACE()
);
#21=(
BOUNDED_SURFACE()
B_SPLINE_SURFACE(5,1,((#25936,#25937),(#25938,#25939),(#25940,#25941),(#25942,
#25943),(#25944,#25945),(#25946,#25947),(#25948,#25949),(#25950,#25951),
(#25952,#25953),(#25954,#25955),(#25956,#25957),(#25958,#25959),(#25960,
#25961),(#25962,#25963),(#25964,#25965),(#25966,#25967),(#25968,#25969),
(#25970,#25971),(#25972,#25973),(#25974,#25975),(#25976,#25977),(#25978,
#25979),(#25980,#25981),(#25982,#25983),(#25984,#25985),(#25986,#25987),
(#25988,#25989),(#25990,#25991),(#25992,#25993),(#25994,#25995),(#25996,
#25997),(#25998,#25999),(#26000,#26001),(#26002,#26003),(#26004,#26005),
(#26006,#26007),(#26008,#26009),(#26010,#26011),(#26012,#26013),(#26014,
#26015),(#26016,#26017),(#26018,#26019),(#26020,#26021),(#26022,#26023),
(#26024,#26025),(#26026,#26027),(#26028,#26029),(#26030,#26031),(#26032,
#26033),(#26034,#26035),(#26036,#26037),(#26038,#26039),(#26040,#26041),
(#26042,#26043),(#26044,#26045),(#26046,#26047),(#26048,#26049),(#26050,
#26051),(#26052,#26053),(#26054,#26055),(#26056,#26057),(#26058,#26059),
(#26060,#26061),(#26062,#26063),(#26064,#26065),(#26066,#26067),(#26068,
#26069),(#26070,#26071),(#26072,#26073),(#26074,#26075)),.UNSPECIFIED.,
 .F.,.F.,.F.)
B_SPLINE_SURFACE_WITH_KNOTS((6,1,1,1,1,1,1,1,1,1,1,1,1,1,1,1,1,1,1,1,1,
1,1,1,1,1,1,1,1,1,1,1,1,1,1,1,1,1,1,1,1,1,1,1,1,1,1,1,1,1,1,1,1,1,1,1,1,
1,1,1,1,1,1,1,1,6),(2,2),(-1.,-0.984615384615383,-0.969230769230768,-0.953846153846152,
-0.938461538461537,-0.923076923076922,-0.907692307692306,-0.892307692307691,
-0.876923076923076,-0.86153846153846,-0.846153846153845,-0.83076923076923,
-0.815384615384614,-0.799999999999999,-0.784615384615384,-0.769230769230768,
-0.753846153846153,-0.738461538461538,-0.723076923076922,-0.707692307692307,
-0.692307692307692,-0.676923076923076,-0.661538461538461,-0.646153846153846,
-0.63076923076923,-0.615384615384615,-0.6,-0.584615384615384,-0.569230769230769,
-0.553846153846154,-0.538461538461538,-0.523076923076923,-0.507692307692308,
-0.492307692307692,-0.476923076923077,-0.461538461538462,-0.446153846153846,
-0.430769230769231,-0.415384615384615,-0.4,-0.384615384615385,-0.369230769230769,
-0.353846153846154,-0.338461538461538,-0.323076923076923,-0.307692307692308,
-0.292307692307692,-0.276923076923077,-0.261538461538462,-0.246153846153846,
-0.230769230769231,-0.215384615384615,-0.2,-0.184615384615385,-0.169230769230769,
-0.153846153846154,-0.138461538461538,-0.123076923076923,-0.107692307692308,
-0.0923076923076923,-0.0769230769230769,-0.0615384615384615,-0.0461538461538462,
-0.0307692307692308,-0.0153846153846154,0.),(-1.,1.),.UNSPECIFIED.)
GEOMETRIC_REPRESENTATION_ITEM()
RATIONAL_B_SPLINE_SURFACE(((1.,1.),(1.,1.),(1.,1.),(1.,1.),(1.,1.),(1.,
1.),(1.,1.),(1.,1.),(1.,1.),(1.,1.),(1.,1.),(1.,1.),(1.,1.),(1.,1.),(1.,
1.),(1.,1.),(1.,1.),(1.,1.),(1.,1.),(1.,1.),(1.,1.),(1.,1.),(1.,1.),(1.,
1.),(1.,1.),(1.,1.),(1.,1.),(1.,1.),(1.,1.),(1.,1.),(1.,1.),(1.,1.),(1.,
1.),(1.,1.),(1.,1.),(1.,1.),(1.,1.),(1.,1.),(1.,1.),(1.,1.),(1.,1.),(1.,
1.),(1.,1.),(1.,1.),(1.,1.),(1.,1.),(1.,1.),(1.,1.),(1.,1.),(1.,1.),(1.,
1.),(1.,1.),(1.,1.),(1.,1.),(1.,1.),(1.,1.),(1.,1.),(1.,1.),(1.,1.),(1.,
1.),(1.,1.),(1.,1.),(1.,1.),(1.,1.),(1.,1.),(1.,1.),(1.,1.),(1.,1.),(1.,
1.),(1.,1.)))
REPRESENTATION_ITEM('')
SURFACE()
);
#22=(
BOUNDED_SURFACE()
B_SPLINE_SURFACE(5,1,((#26152,#26153),(#26154,#26155),(#26156,#26157),(#26158,
#26159),(#26160,#26161),(#26162,#26163),(#26164,#26165),(#26166,#26167),
(#26168,#26169),(#26170,#26171),(#26172,#26173),(#26174,#26175),(#26176,
#26177),(#26178,#26179),(#26180,#26181),(#26182,#26183),(#26184,#26185),
(#26186,#26187),(#26188,#26189),(#26190,#26191),(#26192,#26193),(#26194,
#26195),(#26196,#26197),(#26198,#26199),(#26200,#26201),(#26202,#26203),
(#26204,#26205),(#26206,#26207),(#26208,#26209),(#26210,#26211),(#26212,
#26213),(#26214,#26215),(#26216,#26217),(#26218,#26219),(#26220,#26221),
(#26222,#26223),(#26224,#26225),(#26226,#26227),(#26228,#26229),(#26230,
#26231),(#26232,#26233),(#26234,#26235),(#26236,#26237),(#26238,#26239),
(#26240,#26241),(#26242,#26243),(#26244,#26245),(#26246,#26247),(#26248,
#26249),(#26250,#26251),(#26252,#26253),(#26254,#26255),(#26256,#26257),
(#26258,#26259),(#26260,#26261),(#26262,#26263),(#26264,#26265),(#26266,
#26267),(#26268,#26269),(#26270,#26271),(#26272,#26273),(#26274,#26275),
(#26276,#26277),(#26278,#26279),(#26280,#26281),(#26282,#26283),(#26284,
#26285),(#26286,#26287),(#26288,#26289),(#26290,#26291)),.UNSPECIFIED.,
 .F.,.F.,.F.)
B_SPLINE_SURFACE_WITH_KNOTS((6,1,1,1,1,1,1,1,1,1,1,1,1,1,1,1,1,1,1,1,1,
1,1,1,1,1,1,1,1,1,1,1,1,1,1,1,1,1,1,1,1,1,1,1,1,1,1,1,1,1,1,1,1,1,1,1,1,
1,1,1,1,1,1,1,1,6),(2,2),(-1.,-0.984615384615383,-0.969230769230768,-0.953846153846152,
-0.938461538461537,-0.923076923076922,-0.907692307692306,-0.892307692307691,
-0.876923076923076,-0.86153846153846,-0.846153846153845,-0.83076923076923,
-0.815384615384614,-0.799999999999999,-0.784615384615384,-0.769230769230768,
-0.753846153846153,-0.738461538461538,-0.723076923076922,-0.707692307692307,
-0.692307692307692,-0.676923076923076,-0.661538461538461,-0.646153846153846,
-0.63076923076923,-0.615384615384615,-0.6,-0.584615384615384,-0.569230769230769,
-0.553846153846154,-0.538461538461538,-0.523076923076923,-0.507692307692308,
-0.492307692307692,-0.476923076923077,-0.461538461538462,-0.446153846153846,
-0.430769230769231,-0.415384615384615,-0.4,-0.384615384615385,-0.369230769230769,
-0.353846153846154,-0.338461538461538,-0.323076923076923,-0.307692307692308,
-0.292307692307692,-0.276923076923077,-0.261538461538462,-0.246153846153846,
-0.230769230769231,-0.215384615384615,-0.2,-0.184615384615385,-0.169230769230769,
-0.153846153846154,-0.138461538461538,-0.123076923076923,-0.107692307692308,
-0.0923076923076923,-0.0769230769230769,-0.0615384615384615,-0.0461538461538462,
-0.0307692307692308,-0.0153846153846154,0.),(-1.,1.),.UNSPECIFIED.)
GEOMETRIC_REPRESENTATION_ITEM()
RATIONAL_B_SPLINE_SURFACE(((1.,1.),(1.,1.),(1.,1.),(1.,1.),(1.,1.),(1.,
1.),(1.,1.),(1.,1.),(1.,1.),(1.,1.),(1.,1.),(1.,1.),(1.,1.),(1.,1.),(1.,
1.),(1.,1.),(1.,1.),(1.,1.),(1.,1.),(1.,1.),(1.,1.),(1.,1.),(1.,1.),(1.,
1.),(1.,1.),(1.,1.),(1.,1.),(1.,1.),(1.,1.),(1.,1.),(1.,1.),(1.,1.),(1.,
1.),(1.,1.),(1.,1.),(1.,1.),(1.,1.),(1.,1.),(1.,1.),(1.,1.),(1.,1.),(1.,
1.),(1.,1.),(1.,1.),(1.,1.),(1.,1.),(1.,1.),(1.,1.),(1.,1.),(1.,1.),(1.,
1.),(1.,1.),(1.,1.),(1.,1.),(1.,1.),(1.,1.),(1.,1.),(1.,1.),(1.,1.),(1.,
1.),(1.,1.),(1.,1.),(1.,1.),(1.,1.),(1.,1.),(1.,1.),(1.,1.),(1.,1.),(1.,
1.),(1.,1.)))
REPRESENTATION_ITEM('')
SURFACE()
);
#23=(
BOUNDED_SURFACE()
B_SPLINE_SURFACE(5,1,((#26368,#26369),(#26370,#26371),(#26372,#26373),(#26374,
#26375),(#26376,#26377),(#26378,#26379),(#26380,#26381),(#26382,#26383),
(#26384,#26385),(#26386,#26387),(#26388,#26389),(#26390,#26391),(#26392,
#26393),(#26394,#26395),(#26396,#26397),(#26398,#26399),(#26400,#26401),
(#26402,#26403),(#26404,#26405),(#26406,#26407),(#26408,#26409),(#26410,
#26411),(#26412,#26413),(#26414,#26415),(#26416,#26417),(#26418,#26419),
(#26420,#26421),(#26422,#26423),(#26424,#26425),(#26426,#26427),(#26428,
#26429),(#26430,#26431),(#26432,#26433),(#26434,#26435),(#26436,#26437),
(#26438,#26439),(#26440,#26441),(#26442,#26443),(#26444,#26445),(#26446,
#26447),(#26448,#26449),(#26450,#26451),(#26452,#26453),(#26454,#26455),
(#26456,#26457),(#26458,#26459),(#26460,#26461),(#26462,#26463),(#26464,
#26465),(#26466,#26467),(#26468,#26469),(#26470,#26471),(#26472,#26473),
(#26474,#26475),(#26476,#26477),(#26478,#26479),(#26480,#26481),(#26482,
#26483),(#26484,#26485),(#26486,#26487),(#26488,#26489),(#26490,#26491),
(#26492,#26493),(#26494,#26495),(#26496,#26497),(#26498,#26499),(#26500,
#26501),(#26502,#26503),(#26504,#26505),(#26506,#26507)),.UNSPECIFIED.,
 .F.,.F.,.F.)
B_SPLINE_SURFACE_WITH_KNOTS((6,1,1,1,1,1,1,1,1,1,1,1,1,1,1,1,1,1,1,1,1,
1,1,1,1,1,1,1,1,1,1,1,1,1,1,1,1,1,1,1,1,1,1,1,1,1,1,1,1,1,1,1,1,1,1,1,1,
1,1,1,1,1,1,1,1,6),(2,2),(-1.,-0.984615384615383,-0.969230769230768,-0.953846153846152,
-0.938461538461537,-0.923076923076922,-0.907692307692306,-0.892307692307691,
-0.876923076923076,-0.86153846153846,-0.846153846153845,-0.83076923076923,
-0.815384615384614,-0.799999999999999,-0.784615384615384,-0.769230769230768,
-0.753846153846153,-0.738461538461538,-0.723076923076922,-0.707692307692307,
-0.692307692307692,-0.676923076923076,-0.661538461538461,-0.646153846153846,
-0.63076923076923,-0.615384615384615,-0.6,-0.584615384615384,-0.569230769230769,
-0.553846153846154,-0.538461538461538,-0.523076923076923,-0.507692307692308,
-0.492307692307692,-0.476923076923077,-0.461538461538462,-0.446153846153846,
-0.430769230769231,-0.415384615384615,-0.4,-0.384615384615385,-0.369230769230769,
-0.353846153846154,-0.338461538461538,-0.323076923076923,-0.307692307692308,
-0.292307692307692,-0.276923076923077,-0.261538461538462,-0.246153846153846,
-0.230769230769231,-0.215384615384615,-0.2,-0.184615384615385,-0.169230769230769,
-0.153846153846154,-0.138461538461538,-0.123076923076923,-0.107692307692308,
-0.0923076923076923,-0.0769230769230769,-0.0615384615384615,-0.0461538461538462,
-0.0307692307692308,-0.0153846153846154,0.),(-1.,1.),.UNSPECIFIED.)
GEOMETRIC_REPRESENTATION_ITEM()
RATIONAL_B_SPLINE_SURFACE(((1.,1.),(1.,1.),(1.,1.),(1.,1.),(1.,1.),(1.,
1.),(1.,1.),(1.,1.),(1.,1.),(1.,1.),(1.,1.),(1.,1.),(1.,1.),(1.,1.),(1.,
1.),(1.,1.),(1.,1.),(1.,1.),(1.,1.),(1.,1.),(1.,1.),(1.,1.),(1.,1.),(1.,
1.),(1.,1.),(1.,1.),(1.,1.),(1.,1.),(1.,1.),(1.,1.),(1.,1.),(1.,1.),(1.,
1.),(1.,1.),(1.,1.),(1.,1.),(1.,1.),(1.,1.),(1.,1.),(1.,1.),(1.,1.),(1.,
1.),(1.,1.),(1.,1.),(1.,1.),(1.,1.),(1.,1.),(1.,1.),(1.,1.),(1.,1.),(1.,
1.),(1.,1.),(1.,1.),(1.,1.),(1.,1.),(1.,1.),(1.,1.),(1.,1.),(1.,1.),(1.,
1.),(1.,1.),(1.,1.),(1.,1.),(1.,1.),(1.,1.),(1.,1.),(1.,1.),(1.,1.),(1.,
1.),(1.,1.)))
REPRESENTATION_ITEM('')
SURFACE()
);
#24=(
BOUNDED_SURFACE()
B_SPLINE_SURFACE(5,1,((#26584,#26585),(#26586,#26587),(#26588,#26589),(#26590,
#26591),(#26592,#26593),(#26594,#26595),(#26596,#26597),(#26598,#26599),
(#26600,#26601),(#26602,#26603),(#26604,#26605),(#26606,#26607),(#26608,
#26609),(#26610,#26611),(#26612,#26613),(#26614,#26615),(#26616,#26617),
(#26618,#26619),(#26620,#26621),(#26622,#26623),(#26624,#26625),(#26626,
#26627),(#26628,#26629),(#26630,#26631),(#26632,#26633),(#26634,#26635),
(#26636,#26637),(#26638,#26639),(#26640,#26641),(#26642,#26643),(#26644,
#26645),(#26646,#26647),(#26648,#26649),(#26650,#26651),(#26652,#26653),
(#26654,#26655),(#26656,#26657),(#26658,#26659),(#26660,#26661),(#26662,
#26663),(#26664,#26665),(#26666,#26667),(#26668,#26669),(#26670,#26671),
(#26672,#26673),(#26674,#26675),(#26676,#26677),(#26678,#26679),(#26680,
#26681),(#26682,#26683),(#26684,#26685),(#26686,#26687),(#26688,#26689),
(#26690,#26691),(#26692,#26693),(#26694,#26695),(#26696,#26697),(#26698,
#26699),(#26700,#26701),(#26702,#26703),(#26704,#26705),(#26706,#26707),
(#26708,#26709),(#26710,#26711),(#26712,#26713),(#26714,#26715),(#26716,
#26717),(#26718,#26719),(#26720,#26721),(#26722,#26723)),.UNSPECIFIED.,
 .F.,.F.,.F.)
B_SPLINE_SURFACE_WITH_KNOTS((6,1,1,1,1,1,1,1,1,1,1,1,1,1,1,1,1,1,1,1,1,
1,1,1,1,1,1,1,1,1,1,1,1,1,1,1,1,1,1,1,1,1,1,1,1,1,1,1,1,1,1,1,1,1,1,1,1,
1,1,1,1,1,1,1,1,6),(2,2),(-1.,-0.984615384615383,-0.969230769230768,-0.953846153846152,
-0.938461538461537,-0.923076923076922,-0.907692307692306,-0.892307692307691,
-0.876923076923076,-0.86153846153846,-0.846153846153845,-0.83076923076923,
-0.815384615384614,-0.799999999999999,-0.784615384615384,-0.769230769230768,
-0.753846153846153,-0.738461538461538,-0.723076923076922,-0.707692307692307,
-0.692307692307692,-0.676923076923076,-0.661538461538461,-0.646153846153846,
-0.63076923076923,-0.615384615384615,-0.6,-0.584615384615384,-0.569230769230769,
-0.553846153846154,-0.538461538461538,-0.523076923076923,-0.507692307692308,
-0.492307692307692,-0.476923076923077,-0.461538461538462,-0.446153846153846,
-0.430769230769231,-0.415384615384615,-0.4,-0.384615384615385,-0.369230769230769,
-0.353846153846154,-0.338461538461538,-0.323076923076923,-0.307692307692308,
-0.292307692307692,-0.276923076923077,-0.261538461538462,-0.246153846153846,
-0.230769230769231,-0.215384615384615,-0.2,-0.184615384615385,-0.169230769230769,
-0.153846153846154,-0.138461538461538,-0.123076923076923,-0.107692307692308,
-0.0923076923076923,-0.0769230769230769,-0.0615384615384615,-0.0461538461538462,
-0.0307692307692308,-0.0153846153846154,0.),(-1.,1.),.UNSPECIFIED.)
GEOMETRIC_REPRESENTATION_ITEM()
RATIONAL_B_SPLINE_SURFACE(((1.,1.),(1.,1.),(1.,1.),(1.,1.),(1.,1.),(1.,
1.),(1.,1.),(1.,1.),(1.,1.),(1.,1.),(1.,1.),(1.,1.),(1.,1.),(1.,1.),(1.,
1.),(1.,1.),(1.,1.),(1.,1.),(1.,1.),(1.,1.),(1.,1.),(1.,1.),(1.,1.),(1.,
1.),(1.,1.),(1.,1.),(1.,1.),(1.,1.),(1.,1.),(1.,1.),(1.,1.),(1.,1.),(1.,
1.),(1.,1.),(1.,1.),(1.,1.),(1.,1.),(1.,1.),(1.,1.),(1.,1.),(1.,1.),(1.,
1.),(1.,1.),(1.,1.),(1.,1.),(1.,1.),(1.,1.),(1.,1.),(1.,1.),(1.,1.),(1.,
1.),(1.,1.),(1.,1.),(1.,1.),(1.,1.),(1.,1.),(1.,1.),(1.,1.),(1.,1.),(1.,
1.),(1.,1.),(1.,1.),(1.,1.),(1.,1.),(1.,1.),(1.,1.),(1.,1.),(1.,1.),(1.,
1.),(1.,1.)))
REPRESENTATION_ITEM('')
SURFACE()
);
#25=(
BOUNDED_SURFACE()
B_SPLINE_SURFACE(5,1,((#26800,#26801),(#26802,#26803),(#26804,#26805),(#26806,
#26807),(#26808,#26809),(#26810,#26811),(#26812,#26813),(#26814,#26815),
(#26816,#26817),(#26818,#26819),(#26820,#26821),(#26822,#26823),(#26824,
#26825),(#26826,#26827),(#26828,#26829),(#26830,#26831),(#26832,#26833),
(#26834,#26835),(#26836,#26837),(#26838,#26839),(#26840,#26841),(#26842,
#26843),(#26844,#26845),(#26846,#26847),(#26848,#26849),(#26850,#26851),
(#26852,#26853),(#26854,#26855),(#26856,#26857),(#26858,#26859),(#26860,
#26861),(#26862,#26863),(#26864,#26865),(#26866,#26867),(#26868,#26869),
(#26870,#26871),(#26872,#26873),(#26874,#26875),(#26876,#26877),(#26878,
#26879),(#26880,#26881),(#26882,#26883),(#26884,#26885),(#26886,#26887),
(#26888,#26889),(#26890,#26891),(#26892,#26893),(#26894,#26895),(#26896,
#26897),(#26898,#26899),(#26900,#26901),(#26902,#26903),(#26904,#26905),
(#26906,#26907),(#26908,#26909),(#26910,#26911),(#26912,#26913),(#26914,
#26915),(#26916,#26917),(#26918,#26919),(#26920,#26921),(#26922,#26923),
(#26924,#26925),(#26926,#26927),(#26928,#26929),(#26930,#26931),(#26932,
#26933),(#26934,#26935),(#26936,#26937),(#26938,#26939)),.UNSPECIFIED.,
 .F.,.F.,.F.)
B_SPLINE_SURFACE_WITH_KNOTS((6,1,1,1,1,1,1,1,1,1,1,1,1,1,1,1,1,1,1,1,1,
1,1,1,1,1,1,1,1,1,1,1,1,1,1,1,1,1,1,1,1,1,1,1,1,1,1,1,1,1,1,1,1,1,1,1,1,
1,1,1,1,1,1,1,1,6),(2,2),(-1.,-0.984615384615383,-0.969230769230768,-0.953846153846152,
-0.938461538461537,-0.923076923076922,-0.907692307692306,-0.892307692307691,
-0.876923076923076,-0.86153846153846,-0.846153846153845,-0.83076923076923,
-0.815384615384614,-0.799999999999999,-0.784615384615384,-0.769230769230768,
-0.753846153846153,-0.738461538461538,-0.723076923076922,-0.707692307692307,
-0.692307692307692,-0.676923076923076,-0.661538461538461,-0.646153846153846,
-0.63076923076923,-0.615384615384615,-0.6,-0.584615384615384,-0.569230769230769,
-0.553846153846154,-0.538461538461538,-0.523076923076923,-0.507692307692308,
-0.492307692307692,-0.476923076923077,-0.461538461538462,-0.446153846153846,
-0.430769230769231,-0.415384615384615,-0.4,-0.384615384615385,-0.369230769230769,
-0.353846153846154,-0.338461538461538,-0.323076923076923,-0.307692307692308,
-0.292307692307692,-0.276923076923077,-0.261538461538462,-0.246153846153846,
-0.230769230769231,-0.215384615384615,-0.2,-0.184615384615385,-0.169230769230769,
-0.153846153846154,-0.138461538461538,-0.123076923076923,-0.107692307692308,
-0.0923076923076923,-0.0769230769230769,-0.0615384615384615,-0.0461538461538462,
-0.0307692307692308,-0.0153846153846154,0.),(-1.,1.),.UNSPECIFIED.)
GEOMETRIC_REPRESENTATION_ITEM()
RATIONAL_B_SPLINE_SURFACE(((1.,1.),(1.,1.),(1.,1.),(1.,1.),(1.,1.),(1.,
1.),(1.,1.),(1.,1.),(1.,1.),(1.,1.),(1.,1.),(1.,1.),(1.,1.),(1.,1.),(1.,
1.),(1.,1.),(1.,1.),(1.,1.),(1.,1.),(1.,1.),(1.,1.),(1.,1.),(1.,1.),(1.,
1.),(1.,1.),(1.,1.),(1.,1.),(1.,1.),(1.,1.),(1.,1.),(1.,1.),(1.,1.),(1.,
1.),(1.,1.),(1.,1.),(1.,1.),(1.,1.),(1.,1.),(1.,1.),(1.,1.),(1.,1.),(1.,
1.),(1.,1.),(1.,1.),(1.,1.),(1.,1.),(1.,1.),(1.,1.),(1.,1.),(1.,1.),(1.,
1.),(1.,1.),(1.,1.),(1.,1.),(1.,1.),(1.,1.),(1.,1.),(1.,1.),(1.,1.),(1.,
1.),(1.,1.),(1.,1.),(1.,1.),(1.,1.),(1.,1.),(1.,1.),(1.,1.),(1.,1.),(1.,
1.),(1.,1.)))
REPRESENTATION_ITEM('')
SURFACE()
);
#26=(
BOUNDED_SURFACE()
B_SPLINE_SURFACE(5,1,((#27016,#27017),(#27018,#27019),(#27020,#27021),(#27022,
#27023),(#27024,#27025),(#27026,#27027),(#27028,#27029),(#27030,#27031),
(#27032,#27033),(#27034,#27035),(#27036,#27037),(#27038,#27039),(#27040,
#27041),(#27042,#27043),(#27044,#27045),(#27046,#27047),(#27048,#27049),
(#27050,#27051),(#27052,#27053),(#27054,#27055),(#27056,#27057),(#27058,
#27059),(#27060,#27061),(#27062,#27063),(#27064,#27065),(#27066,#27067),
(#27068,#27069),(#27070,#27071),(#27072,#27073),(#27074,#27075),(#27076,
#27077),(#27078,#27079),(#27080,#27081),(#27082,#27083),(#27084,#27085),
(#27086,#27087),(#27088,#27089),(#27090,#27091),(#27092,#27093),(#27094,
#27095),(#27096,#27097),(#27098,#27099),(#27100,#27101),(#27102,#27103),
(#27104,#27105),(#27106,#27107),(#27108,#27109),(#27110,#27111),(#27112,
#27113),(#27114,#27115),(#27116,#27117),(#27118,#27119),(#27120,#27121),
(#27122,#27123),(#27124,#27125),(#27126,#27127),(#27128,#27129),(#27130,
#27131),(#27132,#27133),(#27134,#27135),(#27136,#27137),(#27138,#27139),
(#27140,#27141),(#27142,#27143),(#27144,#27145),(#27146,#27147),(#27148,
#27149),(#27150,#27151),(#27152,#27153),(#27154,#27155)),.UNSPECIFIED.,
 .F.,.F.,.F.)
B_SPLINE_SURFACE_WITH_KNOTS((6,1,1,1,1,1,1,1,1,1,1,1,1,1,1,1,1,1,1,1,1,
1,1,1,1,1,1,1,1,1,1,1,1,1,1,1,1,1,1,1,1,1,1,1,1,1,1,1,1,1,1,1,1,1,1,1,1,
1,1,1,1,1,1,1,1,6),(2,2),(-1.,-0.984615384615383,-0.969230769230768,-0.953846153846152,
-0.938461538461537,-0.923076923076922,-0.907692307692306,-0.892307692307691,
-0.876923076923076,-0.86153846153846,-0.846153846153845,-0.83076923076923,
-0.815384615384614,-0.799999999999999,-0.784615384615384,-0.769230769230768,
-0.753846153846153,-0.738461538461538,-0.723076923076922,-0.707692307692307,
-0.692307692307692,-0.676923076923076,-0.661538461538461,-0.646153846153846,
-0.63076923076923,-0.615384615384615,-0.6,-0.584615384615384,-0.569230769230769,
-0.553846153846154,-0.538461538461538,-0.523076923076923,-0.507692307692308,
-0.492307692307692,-0.476923076923077,-0.461538461538462,-0.446153846153846,
-0.430769230769231,-0.415384615384615,-0.4,-0.384615384615385,-0.369230769230769,
-0.353846153846154,-0.338461538461538,-0.323076923076923,-0.307692307692308,
-0.292307692307692,-0.276923076923077,-0.261538461538462,-0.246153846153846,
-0.230769230769231,-0.215384615384615,-0.2,-0.184615384615385,-0.169230769230769,
-0.153846153846154,-0.138461538461538,-0.123076923076923,-0.107692307692308,
-0.0923076923076923,-0.0769230769230769,-0.0615384615384615,-0.0461538461538462,
-0.0307692307692308,-0.0153846153846154,0.),(-1.,1.),.UNSPECIFIED.)
GEOMETRIC_REPRESENTATION_ITEM()
RATIONAL_B_SPLINE_SURFACE(((1.,1.),(1.,1.),(1.,1.),(1.,1.),(1.,1.),(1.,
1.),(1.,1.),(1.,1.),(1.,1.),(1.,1.),(1.,1.),(1.,1.),(1.,1.),(1.,1.),(1.,
1.),(1.,1.),(1.,1.),(1.,1.),(1.,1.),(1.,1.),(1.,1.),(1.,1.),(1.,1.),(1.,
1.),(1.,1.),(1.,1.),(1.,1.),(1.,1.),(1.,1.),(1.,1.),(1.,1.),(1.,1.),(1.,
1.),(1.,1.),(1.,1.),(1.,1.),(1.,1.),(1.,1.),(1.,1.),(1.,1.),(1.,1.),(1.,
1.),(1.,1.),(1.,1.),(1.,1.),(1.,1.),(1.,1.),(1.,1.),(1.,1.),(1.,1.),(1.,
1.),(1.,1.),(1.,1.),(1.,1.),(1.,1.),(1.,1.),(1.,1.),(1.,1.),(1.,1.),(1.,
1.),(1.,1.),(1.,1.),(1.,1.),(1.,1.),(1.,1.),(1.,1.),(1.,1.),(1.,1.),(1.,
1.),(1.,1.)))
REPRESENTATION_ITEM('')
SURFACE()
);
#27=(
BOUNDED_SURFACE()
B_SPLINE_SURFACE(5,1,((#27232,#27233),(#27234,#27235),(#27236,#27237),(#27238,
#27239),(#27240,#27241),(#27242,#27243),(#27244,#27245),(#27246,#27247),
(#27248,#27249),(#27250,#27251),(#27252,#27253),(#27254,#27255),(#27256,
#27257),(#27258,#27259),(#27260,#27261),(#27262,#27263),(#27264,#27265),
(#27266,#27267),(#27268,#27269),(#27270,#27271),(#27272,#27273),(#27274,
#27275),(#27276,#27277),(#27278,#27279),(#27280,#27281),(#27282,#27283),
(#27284,#27285),(#27286,#27287),(#27288,#27289),(#27290,#27291),(#27292,
#27293),(#27294,#27295),(#27296,#27297),(#27298,#27299),(#27300,#27301),
(#27302,#27303),(#27304,#27305),(#27306,#27307),(#27308,#27309),(#27310,
#27311),(#27312,#27313),(#27314,#27315),(#27316,#27317),(#27318,#27319),
(#27320,#27321),(#27322,#27323),(#27324,#27325),(#27326,#27327),(#27328,
#27329),(#27330,#27331),(#27332,#27333),(#27334,#27335),(#27336,#27337),
(#27338,#27339),(#27340,#27341),(#27342,#27343),(#27344,#27345),(#27346,
#27347),(#27348,#27349),(#27350,#27351),(#27352,#27353),(#27354,#27355),
(#27356,#27357),(#27358,#27359),(#27360,#27361),(#27362,#27363),(#27364,
#27365),(#27366,#27367),(#27368,#27369),(#27370,#27371)),.UNSPECIFIED.,
 .F.,.F.,.F.)
B_SPLINE_SURFACE_WITH_KNOTS((6,1,1,1,1,1,1,1,1,1,1,1,1,1,1,1,1,1,1,1,1,
1,1,1,1,1,1,1,1,1,1,1,1,1,1,1,1,1,1,1,1,1,1,1,1,1,1,1,1,1,1,1,1,1,1,1,1,
1,1,1,1,1,1,1,1,6),(2,2),(-1.,-0.984615384615383,-0.969230769230768,-0.953846153846152,
-0.938461538461537,-0.923076923076922,-0.907692307692306,-0.892307692307691,
-0.876923076923076,-0.86153846153846,-0.846153846153845,-0.83076923076923,
-0.815384615384614,-0.799999999999999,-0.784615384615384,-0.769230769230768,
-0.753846153846153,-0.738461538461538,-0.723076923076922,-0.707692307692307,
-0.692307692307692,-0.676923076923076,-0.661538461538461,-0.646153846153846,
-0.63076923076923,-0.615384615384615,-0.6,-0.584615384615384,-0.569230769230769,
-0.553846153846154,-0.538461538461538,-0.523076923076923,-0.507692307692308,
-0.492307692307692,-0.476923076923077,-0.461538461538462,-0.446153846153846,
-0.430769230769231,-0.415384615384615,-0.4,-0.384615384615385,-0.369230769230769,
-0.353846153846154,-0.338461538461538,-0.323076923076923,-0.307692307692308,
-0.292307692307692,-0.276923076923077,-0.261538461538462,-0.246153846153846,
-0.230769230769231,-0.215384615384615,-0.2,-0.184615384615385,-0.169230769230769,
-0.153846153846154,-0.138461538461538,-0.123076923076923,-0.107692307692308,
-0.0923076923076923,-0.0769230769230769,-0.0615384615384615,-0.0461538461538462,
-0.0307692307692308,-0.0153846153846154,0.),(-1.,1.),.UNSPECIFIED.)
GEOMETRIC_REPRESENTATION_ITEM()
RATIONAL_B_SPLINE_SURFACE(((1.,1.),(1.,1.),(1.,1.),(1.,1.),(1.,1.),(1.,
1.),(1.,1.),(1.,1.),(1.,1.),(1.,1.),(1.,1.),(1.,1.),(1.,1.),(1.,1.),(1.,
1.),(1.,1.),(1.,1.),(1.,1.),(1.,1.),(1.,1.),(1.,1.),(1.,1.),(1.,1.),(1.,
1.),(1.,1.),(1.,1.),(1.,1.),(1.,1.),(1.,1.),(1.,1.),(1.,1.),(1.,1.),(1.,
1.),(1.,1.),(1.,1.),(1.,1.),(1.,1.),(1.,1.),(1.,1.),(1.,1.),(1.,1.),(1.,
1.),(1.,1.),(1.,1.),(1.,1.),(1.,1.),(1.,1.),(1.,1.),(1.,1.),(1.,1.),(1.,
1.),(1.,1.),(1.,1.),(1.,1.),(1.,1.),(1.,1.),(1.,1.),(1.,1.),(1.,1.),(1.,
1.),(1.,1.),(1.,1.),(1.,1.),(1.,1.),(1.,1.),(1.,1.),(1.,1.),(1.,1.),(1.,
1.),(1.,1.)))
REPRESENTATION_ITEM('')
SURFACE()
);
#28=(
BOUNDED_SURFACE()
B_SPLINE_SURFACE(5,1,((#27448,#27449),(#27450,#27451),(#27452,#27453),(#27454,
#27455),(#27456,#27457),(#27458,#27459),(#27460,#27461),(#27462,#27463),
(#27464,#27465),(#27466,#27467),(#27468,#27469),(#27470,#27471),(#27472,
#27473),(#27474,#27475),(#27476,#27477),(#27478,#27479),(#27480,#27481),
(#27482,#27483),(#27484,#27485),(#27486,#27487),(#27488,#27489),(#27490,
#27491),(#27492,#27493),(#27494,#27495),(#27496,#27497),(#27498,#27499),
(#27500,#27501),(#27502,#27503),(#27504,#27505),(#27506,#27507),(#27508,
#27509),(#27510,#27511),(#27512,#27513),(#27514,#27515),(#27516,#27517),
(#27518,#27519),(#27520,#27521),(#27522,#27523),(#27524,#27525),(#27526,
#27527),(#27528,#27529),(#27530,#27531),(#27532,#27533),(#27534,#27535),
(#27536,#27537),(#27538,#27539),(#27540,#27541),(#27542,#27543),(#27544,
#27545),(#27546,#27547),(#27548,#27549),(#27550,#27551),(#27552,#27553),
(#27554,#27555),(#27556,#27557),(#27558,#27559),(#27560,#27561),(#27562,
#27563),(#27564,#27565),(#27566,#27567),(#27568,#27569),(#27570,#27571),
(#27572,#27573),(#27574,#27575),(#27576,#27577),(#27578,#27579),(#27580,
#27581),(#27582,#27583),(#27584,#27585),(#27586,#27587)),.UNSPECIFIED.,
 .F.,.F.,.F.)
B_SPLINE_SURFACE_WITH_KNOTS((6,1,1,1,1,1,1,1,1,1,1,1,1,1,1,1,1,1,1,1,1,
1,1,1,1,1,1,1,1,1,1,1,1,1,1,1,1,1,1,1,1,1,1,1,1,1,1,1,1,1,1,1,1,1,1,1,1,
1,1,1,1,1,1,1,1,6),(2,2),(-1.,-0.984615384615383,-0.969230769230768,-0.953846153846152,
-0.938461538461537,-0.923076923076922,-0.907692307692306,-0.892307692307691,
-0.876923076923076,-0.86153846153846,-0.846153846153845,-0.83076923076923,
-0.815384615384614,-0.799999999999999,-0.784615384615384,-0.769230769230768,
-0.753846153846153,-0.738461538461538,-0.723076923076922,-0.707692307692307,
-0.692307692307692,-0.676923076923076,-0.661538461538461,-0.646153846153846,
-0.63076923076923,-0.615384615384615,-0.6,-0.584615384615384,-0.569230769230769,
-0.553846153846154,-0.538461538461538,-0.523076923076923,-0.507692307692308,
-0.492307692307692,-0.476923076923077,-0.461538461538462,-0.446153846153846,
-0.430769230769231,-0.415384615384615,-0.4,-0.384615384615385,-0.369230769230769,
-0.353846153846154,-0.338461538461538,-0.323076923076923,-0.307692307692308,
-0.292307692307692,-0.276923076923077,-0.261538461538462,-0.246153846153846,
-0.230769230769231,-0.215384615384615,-0.2,-0.184615384615385,-0.169230769230769,
-0.153846153846154,-0.138461538461538,-0.123076923076923,-0.107692307692308,
-0.0923076923076923,-0.0769230769230769,-0.0615384615384615,-0.0461538461538462,
-0.0307692307692308,-0.0153846153846154,0.),(-1.,1.),.UNSPECIFIED.)
GEOMETRIC_REPRESENTATION_ITEM()
RATIONAL_B_SPLINE_SURFACE(((1.,1.),(1.,1.),(1.,1.),(1.,1.),(1.,1.),(1.,
1.),(1.,1.),(1.,1.),(1.,1.),(1.,1.),(1.,1.),(1.,1.),(1.,1.),(1.,1.),(1.,
1.),(1.,1.),(1.,1.),(1.,1.),(1.,1.),(1.,1.),(1.,1.),(1.,1.),(1.,1.),(1.,
1.),(1.,1.),(1.,1.),(1.,1.),(1.,1.),(1.,1.),(1.,1.),(1.,1.),(1.,1.),(1.,
1.),(1.,1.),(1.,1.),(1.,1.),(1.,1.),(1.,1.),(1.,1.),(1.,1.),(1.,1.),(1.,
1.),(1.,1.),(1.,1.),(1.,1.),(1.,1.),(1.,1.),(1.,1.),(1.,1.),(1.,1.),(1.,
1.),(1.,1.),(1.,1.),(1.,1.),(1.,1.),(1.,1.),(1.,1.),(1.,1.),(1.,1.),(1.,
1.),(1.,1.),(1.,1.),(1.,1.),(1.,1.),(1.,1.),(1.,1.),(1.,1.),(1.,1.),(1.,
1.),(1.,1.)))
REPRESENTATION_ITEM('')
SURFACE()
);
#29=(
BOUNDED_SURFACE()
B_SPLINE_SURFACE(5,1,((#27664,#27665),(#27666,#27667),(#27668,#27669),(#27670,
#27671),(#27672,#27673),(#27674,#27675),(#27676,#27677),(#27678,#27679),
(#27680,#27681),(#27682,#27683),(#27684,#27685),(#27686,#27687),(#27688,
#27689),(#27690,#27691),(#27692,#27693),(#27694,#27695),(#27696,#27697),
(#27698,#27699),(#27700,#27701),(#27702,#27703),(#27704,#27705),(#27706,
#27707),(#27708,#27709),(#27710,#27711),(#27712,#27713),(#27714,#27715),
(#27716,#27717),(#27718,#27719),(#27720,#27721),(#27722,#27723),(#27724,
#27725),(#27726,#27727),(#27728,#27729),(#27730,#27731),(#27732,#27733),
(#27734,#27735),(#27736,#27737),(#27738,#27739),(#27740,#27741),(#27742,
#27743),(#27744,#27745),(#27746,#27747),(#27748,#27749),(#27750,#27751),
(#27752,#27753),(#27754,#27755),(#27756,#27757),(#27758,#27759),(#27760,
#27761),(#27762,#27763),(#27764,#27765),(#27766,#27767),(#27768,#27769),
(#27770,#27771),(#27772,#27773),(#27774,#27775),(#27776,#27777),(#27778,
#27779),(#27780,#27781),(#27782,#27783),(#27784,#27785),(#27786,#27787),
(#27788,#27789),(#27790,#27791),(#27792,#27793),(#27794,#27795),(#27796,
#27797),(#27798,#27799),(#27800,#27801),(#27802,#27803)),.UNSPECIFIED.,
 .F.,.F.,.F.)
B_SPLINE_SURFACE_WITH_KNOTS((6,1,1,1,1,1,1,1,1,1,1,1,1,1,1,1,1,1,1,1,1,
1,1,1,1,1,1,1,1,1,1,1,1,1,1,1,1,1,1,1,1,1,1,1,1,1,1,1,1,1,1,1,1,1,1,1,1,
1,1,1,1,1,1,1,1,6),(2,2),(-1.,-0.984615384615383,-0.969230769230768,-0.953846153846152,
-0.938461538461537,-0.923076923076922,-0.907692307692306,-0.892307692307691,
-0.876923076923076,-0.86153846153846,-0.846153846153845,-0.83076923076923,
-0.815384615384614,-0.799999999999999,-0.784615384615384,-0.769230769230768,
-0.753846153846153,-0.738461538461538,-0.723076923076922,-0.707692307692307,
-0.692307692307692,-0.676923076923076,-0.661538461538461,-0.646153846153846,
-0.63076923076923,-0.615384615384615,-0.6,-0.584615384615384,-0.569230769230769,
-0.553846153846154,-0.538461538461538,-0.523076923076923,-0.507692307692308,
-0.492307692307692,-0.476923076923077,-0.461538461538462,-0.446153846153846,
-0.430769230769231,-0.415384615384615,-0.4,-0.384615384615385,-0.369230769230769,
-0.353846153846154,-0.338461538461538,-0.323076923076923,-0.307692307692308,
-0.292307692307692,-0.276923076923077,-0.261538461538462,-0.246153846153846,
-0.230769230769231,-0.215384615384615,-0.2,-0.184615384615385,-0.169230769230769,
-0.153846153846154,-0.138461538461538,-0.123076923076923,-0.107692307692308,
-0.0923076923076923,-0.0769230769230769,-0.0615384615384615,-0.0461538461538462,
-0.0307692307692308,-0.0153846153846154,0.),(-1.,1.),.UNSPECIFIED.)
GEOMETRIC_REPRESENTATION_ITEM()
RATIONAL_B_SPLINE_SURFACE(((1.,1.),(1.,1.),(1.,1.),(1.,1.),(1.,1.),(1.,
1.),(1.,1.),(1.,1.),(1.,1.),(1.,1.),(1.,1.),(1.,1.),(1.,1.),(1.,1.),(1.,
1.),(1.,1.),(1.,1.),(1.,1.),(1.,1.),(1.,1.),(1.,1.),(1.,1.),(1.,1.),(1.,
1.),(1.,1.),(1.,1.),(1.,1.),(1.,1.),(1.,1.),(1.,1.),(1.,1.),(1.,1.),(1.,
1.),(1.,1.),(1.,1.),(1.,1.),(1.,1.),(1.,1.),(1.,1.),(1.,1.),(1.,1.),(1.,
1.),(1.,1.),(1.,1.),(1.,1.),(1.,1.),(1.,1.),(1.,1.),(1.,1.),(1.,1.),(1.,
1.),(1.,1.),(1.,1.),(1.,1.),(1.,1.),(1.,1.),(1.,1.),(1.,1.),(1.,1.),(1.,
1.),(1.,1.),(1.,1.),(1.,1.),(1.,1.),(1.,1.),(1.,1.),(1.,1.),(1.,1.),(1.,
1.),(1.,1.)))
REPRESENTATION_ITEM('')
SURFACE()
);
#30=(
BOUNDED_SURFACE()
B_SPLINE_SURFACE(5,1,((#27880,#27881),(#27882,#27883),(#27884,#27885),(#27886,
#27887),(#27888,#27889),(#27890,#27891),(#27892,#27893),(#27894,#27895),
(#27896,#27897),(#27898,#27899),(#27900,#27901),(#27902,#27903),(#27904,
#27905),(#27906,#27907),(#27908,#27909),(#27910,#27911),(#27912,#27913),
(#27914,#27915),(#27916,#27917),(#27918,#27919),(#27920,#27921),(#27922,
#27923),(#27924,#27925),(#27926,#27927),(#27928,#27929),(#27930,#27931),
(#27932,#27933),(#27934,#27935),(#27936,#27937),(#27938,#27939),(#27940,
#27941),(#27942,#27943),(#27944,#27945),(#27946,#27947),(#27948,#27949),
(#27950,#27951),(#27952,#27953),(#27954,#27955),(#27956,#27957),(#27958,
#27959),(#27960,#27961),(#27962,#27963),(#27964,#27965),(#27966,#27967),
(#27968,#27969),(#27970,#27971),(#27972,#27973),(#27974,#27975),(#27976,
#27977),(#27978,#27979),(#27980,#27981),(#27982,#27983),(#27984,#27985),
(#27986,#27987),(#27988,#27989),(#27990,#27991),(#27992,#27993),(#27994,
#27995),(#27996,#27997),(#27998,#27999),(#28000,#28001),(#28002,#28003),
(#28004,#28005),(#28006,#28007),(#28008,#28009),(#28010,#28011),(#28012,
#28013),(#28014,#28015),(#28016,#28017),(#28018,#28019)),.UNSPECIFIED.,
 .F.,.F.,.F.)
B_SPLINE_SURFACE_WITH_KNOTS((6,1,1,1,1,1,1,1,1,1,1,1,1,1,1,1,1,1,1,1,1,
1,1,1,1,1,1,1,1,1,1,1,1,1,1,1,1,1,1,1,1,1,1,1,1,1,1,1,1,1,1,1,1,1,1,1,1,
1,1,1,1,1,1,1,1,6),(2,2),(-1.,-0.984615384615383,-0.969230769230768,-0.953846153846152,
-0.938461538461537,-0.923076923076922,-0.907692307692306,-0.892307692307691,
-0.876923076923076,-0.86153846153846,-0.846153846153845,-0.83076923076923,
-0.815384615384614,-0.799999999999999,-0.784615384615384,-0.769230769230768,
-0.753846153846153,-0.738461538461538,-0.723076923076922,-0.707692307692307,
-0.692307692307692,-0.676923076923076,-0.661538461538461,-0.646153846153846,
-0.63076923076923,-0.615384615384615,-0.6,-0.584615384615384,-0.569230769230769,
-0.553846153846154,-0.538461538461538,-0.523076923076923,-0.507692307692308,
-0.492307692307692,-0.476923076923077,-0.461538461538462,-0.446153846153846,
-0.430769230769231,-0.415384615384615,-0.4,-0.384615384615385,-0.369230769230769,
-0.353846153846154,-0.338461538461538,-0.323076923076923,-0.307692307692308,
-0.292307692307692,-0.276923076923077,-0.261538461538462,-0.246153846153846,
-0.230769230769231,-0.215384615384615,-0.2,-0.184615384615385,-0.169230769230769,
-0.153846153846154,-0.138461538461538,-0.123076923076923,-0.107692307692308,
-0.0923076923076923,-0.0769230769230769,-0.0615384615384615,-0.0461538461538462,
-0.0307692307692308,-0.0153846153846154,0.),(-1.,1.),.UNSPECIFIED.)
GEOMETRIC_REPRESENTATION_ITEM()
RATIONAL_B_SPLINE_SURFACE(((1.,1.),(1.,1.),(1.,1.),(1.,1.),(1.,1.),(1.,
1.),(1.,1.),(1.,1.),(1.,1.),(1.,1.),(1.,1.),(1.,1.),(1.,1.),(1.,1.),(1.,
1.),(1.,1.),(1.,1.),(1.,1.),(1.,1.),(1.,1.),(1.,1.),(1.,1.),(1.,1.),(1.,
1.),(1.,1.),(1.,1.),(1.,1.),(1.,1.),(1.,1.),(1.,1.),(1.,1.),(1.,1.),(1.,
1.),(1.,1.),(1.,1.),(1.,1.),(1.,1.),(1.,1.),(1.,1.),(1.,1.),(1.,1.),(1.,
1.),(1.,1.),(1.,1.),(1.,1.),(1.,1.),(1.,1.),(1.,1.),(1.,1.),(1.,1.),(1.,
1.),(1.,1.),(1.,1.),(1.,1.),(1.,1.),(1.,1.),(1.,1.),(1.,1.),(1.,1.),(1.,
1.),(1.,1.),(1.,1.),(1.,1.),(1.,1.),(1.,1.),(1.,1.),(1.,1.),(1.,1.),(1.,
1.),(1.,1.)))
REPRESENTATION_ITEM('')
SURFACE()
);
#31=(
BOUNDED_SURFACE()
B_SPLINE_SURFACE(5,1,((#28096,#28097),(#28098,#28099),(#28100,#28101),(#28102,
#28103),(#28104,#28105),(#28106,#28107),(#28108,#28109),(#28110,#28111),
(#28112,#28113),(#28114,#28115),(#28116,#28117),(#28118,#28119),(#28120,
#28121),(#28122,#28123),(#28124,#28125),(#28126,#28127),(#28128,#28129),
(#28130,#28131),(#28132,#28133),(#28134,#28135),(#28136,#28137),(#28138,
#28139),(#28140,#28141),(#28142,#28143),(#28144,#28145),(#28146,#28147),
(#28148,#28149),(#28150,#28151),(#28152,#28153),(#28154,#28155),(#28156,
#28157),(#28158,#28159),(#28160,#28161),(#28162,#28163),(#28164,#28165),
(#28166,#28167),(#28168,#28169),(#28170,#28171),(#28172,#28173),(#28174,
#28175),(#28176,#28177),(#28178,#28179),(#28180,#28181),(#28182,#28183),
(#28184,#28185),(#28186,#28187),(#28188,#28189),(#28190,#28191),(#28192,
#28193),(#28194,#28195),(#28196,#28197),(#28198,#28199),(#28200,#28201),
(#28202,#28203),(#28204,#28205),(#28206,#28207),(#28208,#28209),(#28210,
#28211),(#28212,#28213),(#28214,#28215),(#28216,#28217),(#28218,#28219),
(#28220,#28221),(#28222,#28223),(#28224,#28225),(#28226,#28227),(#28228,
#28229),(#28230,#28231),(#28232,#28233),(#28234,#28235)),.UNSPECIFIED.,
 .F.,.F.,.F.)
B_SPLINE_SURFACE_WITH_KNOTS((6,1,1,1,1,1,1,1,1,1,1,1,1,1,1,1,1,1,1,1,1,
1,1,1,1,1,1,1,1,1,1,1,1,1,1,1,1,1,1,1,1,1,1,1,1,1,1,1,1,1,1,1,1,1,1,1,1,
1,1,1,1,1,1,1,1,6),(2,2),(-1.,-0.984615384615383,-0.969230769230768,-0.953846153846152,
-0.938461538461537,-0.923076923076922,-0.907692307692306,-0.892307692307691,
-0.876923076923076,-0.86153846153846,-0.846153846153845,-0.83076923076923,
-0.815384615384614,-0.799999999999999,-0.784615384615384,-0.769230769230768,
-0.753846153846153,-0.738461538461538,-0.723076923076922,-0.707692307692307,
-0.692307692307692,-0.676923076923076,-0.661538461538461,-0.646153846153846,
-0.63076923076923,-0.615384615384615,-0.6,-0.584615384615384,-0.569230769230769,
-0.553846153846154,-0.538461538461538,-0.523076923076923,-0.507692307692308,
-0.492307692307692,-0.476923076923077,-0.461538461538462,-0.446153846153846,
-0.430769230769231,-0.415384615384615,-0.4,-0.384615384615385,-0.369230769230769,
-0.353846153846154,-0.338461538461538,-0.323076923076923,-0.307692307692308,
-0.292307692307692,-0.276923076923077,-0.261538461538462,-0.246153846153846,
-0.230769230769231,-0.215384615384615,-0.2,-0.184615384615385,-0.169230769230769,
-0.153846153846154,-0.138461538461538,-0.123076923076923,-0.107692307692308,
-0.0923076923076923,-0.0769230769230769,-0.0615384615384615,-0.0461538461538462,
-0.0307692307692308,-0.0153846153846154,0.),(-1.,1.),.UNSPECIFIED.)
GEOMETRIC_REPRESENTATION_ITEM()
RATIONAL_B_SPLINE_SURFACE(((1.,1.),(1.,1.),(1.,1.),(1.,1.),(1.,1.),(1.,
1.),(1.,1.),(1.,1.),(1.,1.),(1.,1.),(1.,1.),(1.,1.),(1.,1.),(1.,1.),(1.,
1.),(1.,1.),(1.,1.),(1.,1.),(1.,1.),(1.,1.),(1.,1.),(1.,1.),(1.,1.),(1.,
1.),(1.,1.),(1.,1.),(1.,1.),(1.,1.),(1.,1.),(1.,1.),(1.,1.),(1.,1.),(1.,
1.),(1.,1.),(1.,1.),(1.,1.),(1.,1.),(1.,1.),(1.,1.),(1.,1.),(1.,1.),(1.,
1.),(1.,1.),(1.,1.),(1.,1.),(1.,1.),(1.,1.),(1.,1.),(1.,1.),(1.,1.),(1.,
1.),(1.,1.),(1.,1.),(1.,1.),(1.,1.),(1.,1.),(1.,1.),(1.,1.),(1.,1.),(1.,
1.),(1.,1.),(1.,1.),(1.,1.),(1.,1.),(1.,1.),(1.,1.),(1.,1.),(1.,1.),(1.,
1.),(1.,1.)))
REPRESENTATION_ITEM('')
SURFACE()
);
#32=(
BOUNDED_SURFACE()
B_SPLINE_SURFACE(5,1,((#28312,#28313),(#28314,#28315),(#28316,#28317),(#28318,
#28319),(#28320,#28321),(#28322,#28323),(#28324,#28325),(#28326,#28327),
(#28328,#28329),(#28330,#28331),(#28332,#28333),(#28334,#28335),(#28336,
#28337),(#28338,#28339),(#28340,#28341),(#28342,#28343),(#28344,#28345),
(#28346,#28347),(#28348,#28349),(#28350,#28351),(#28352,#28353),(#28354,
#28355),(#28356,#28357),(#28358,#28359),(#28360,#28361),(#28362,#28363),
(#28364,#28365),(#28366,#28367),(#28368,#28369),(#28370,#28371),(#28372,
#28373),(#28374,#28375),(#28376,#28377),(#28378,#28379),(#28380,#28381),
(#28382,#28383),(#28384,#28385),(#28386,#28387),(#28388,#28389),(#28390,
#28391),(#28392,#28393),(#28394,#28395),(#28396,#28397),(#28398,#28399),
(#28400,#28401),(#28402,#28403),(#28404,#28405),(#28406,#28407),(#28408,
#28409),(#28410,#28411),(#28412,#28413),(#28414,#28415),(#28416,#28417),
(#28418,#28419),(#28420,#28421),(#28422,#28423),(#28424,#28425),(#28426,
#28427),(#28428,#28429),(#28430,#28431),(#28432,#28433),(#28434,#28435),
(#28436,#28437),(#28438,#28439),(#28440,#28441),(#28442,#28443),(#28444,
#28445),(#28446,#28447),(#28448,#28449),(#28450,#28451)),.UNSPECIFIED.,
 .F.,.F.,.F.)
B_SPLINE_SURFACE_WITH_KNOTS((6,1,1,1,1,1,1,1,1,1,1,1,1,1,1,1,1,1,1,1,1,
1,1,1,1,1,1,1,1,1,1,1,1,1,1,1,1,1,1,1,1,1,1,1,1,1,1,1,1,1,1,1,1,1,1,1,1,
1,1,1,1,1,1,1,1,6),(2,2),(-1.,-0.984615384615383,-0.969230769230768,-0.953846153846152,
-0.938461538461537,-0.923076923076922,-0.907692307692306,-0.892307692307691,
-0.876923076923076,-0.86153846153846,-0.846153846153845,-0.83076923076923,
-0.815384615384614,-0.799999999999999,-0.784615384615384,-0.769230769230768,
-0.753846153846153,-0.738461538461538,-0.723076923076922,-0.707692307692307,
-0.692307692307692,-0.676923076923076,-0.661538461538461,-0.646153846153846,
-0.63076923076923,-0.615384615384615,-0.6,-0.584615384615384,-0.569230769230769,
-0.553846153846154,-0.538461538461538,-0.523076923076923,-0.507692307692308,
-0.492307692307692,-0.476923076923077,-0.461538461538462,-0.446153846153846,
-0.430769230769231,-0.415384615384615,-0.4,-0.384615384615385,-0.369230769230769,
-0.353846153846154,-0.338461538461538,-0.323076923076923,-0.307692307692308,
-0.292307692307692,-0.276923076923077,-0.261538461538462,-0.246153846153846,
-0.230769230769231,-0.215384615384615,-0.2,-0.184615384615385,-0.169230769230769,
-0.153846153846154,-0.138461538461538,-0.123076923076923,-0.107692307692308,
-0.0923076923076923,-0.0769230769230769,-0.0615384615384615,-0.0461538461538462,
-0.0307692307692308,-0.0153846153846154,0.),(-1.,1.),.UNSPECIFIED.)
GEOMETRIC_REPRESENTATION_ITEM()
RATIONAL_B_SPLINE_SURFACE(((1.,1.),(1.,1.),(1.,1.),(1.,1.),(1.,1.),(1.,
1.),(1.,1.),(1.,1.),(1.,1.),(1.,1.),(1.,1.),(1.,1.),(1.,1.),(1.,1.),(1.,
1.),(1.,1.),(1.,1.),(1.,1.),(1.,1.),(1.,1.),(1.,1.),(1.,1.),(1.,1.),(1.,
1.),(1.,1.),(1.,1.),(1.,1.),(1.,1.),(1.,1.),(1.,1.),(1.,1.),(1.,1.),(1.,
1.),(1.,1.),(1.,1.),(1.,1.),(1.,1.),(1.,1.),(1.,1.),(1.,1.),(1.,1.),(1.,
1.),(1.,1.),(1.,1.),(1.,1.),(1.,1.),(1.,1.),(1.,1.),(1.,1.),(1.,1.),(1.,
1.),(1.,1.),(1.,1.),(1.,1.),(1.,1.),(1.,1.),(1.,1.),(1.,1.),(1.,1.),(1.,
1.),(1.,1.),(1.,1.),(1.,1.),(1.,1.),(1.,1.),(1.,1.),(1.,1.),(1.,1.),(1.,
1.),(1.,1.)))
REPRESENTATION_ITEM('')
SURFACE()
);
#33=(
BOUNDED_SURFACE()
B_SPLINE_SURFACE(5,1,((#28528,#28529),(#28530,#28531),(#28532,#28533),(#28534,
#28535),(#28536,#28537),(#28538,#28539),(#28540,#28541),(#28542,#28543),
(#28544,#28545),(#28546,#28547),(#28548,#28549),(#28550,#28551),(#28552,
#28553),(#28554,#28555),(#28556,#28557),(#28558,#28559),(#28560,#28561),
(#28562,#28563),(#28564,#28565),(#28566,#28567),(#28568,#28569),(#28570,
#28571),(#28572,#28573),(#28574,#28575),(#28576,#28577),(#28578,#28579),
(#28580,#28581),(#28582,#28583),(#28584,#28585),(#28586,#28587),(#28588,
#28589),(#28590,#28591),(#28592,#28593),(#28594,#28595),(#28596,#28597),
(#28598,#28599),(#28600,#28601),(#28602,#28603),(#28604,#28605),(#28606,
#28607),(#28608,#28609),(#28610,#28611),(#28612,#28613),(#28614,#28615),
(#28616,#28617),(#28618,#28619),(#28620,#28621),(#28622,#28623),(#28624,
#28625),(#28626,#28627),(#28628,#28629),(#28630,#28631),(#28632,#28633),
(#28634,#28635),(#28636,#28637),(#28638,#28639),(#28640,#28641),(#28642,
#28643),(#28644,#28645),(#28646,#28647),(#28648,#28649),(#28650,#28651),
(#28652,#28653),(#28654,#28655),(#28656,#28657),(#28658,#28659),(#28660,
#28661),(#28662,#28663),(#28664,#28665),(#28666,#28667)),.UNSPECIFIED.,
 .F.,.F.,.F.)
B_SPLINE_SURFACE_WITH_KNOTS((6,1,1,1,1,1,1,1,1,1,1,1,1,1,1,1,1,1,1,1,1,
1,1,1,1,1,1,1,1,1,1,1,1,1,1,1,1,1,1,1,1,1,1,1,1,1,1,1,1,1,1,1,1,1,1,1,1,
1,1,1,1,1,1,1,1,6),(2,2),(-1.,-0.984615384615383,-0.969230769230768,-0.953846153846152,
-0.938461538461537,-0.923076923076922,-0.907692307692306,-0.892307692307691,
-0.876923076923076,-0.86153846153846,-0.846153846153845,-0.83076923076923,
-0.815384615384614,-0.799999999999999,-0.784615384615384,-0.769230769230768,
-0.753846153846153,-0.738461538461538,-0.723076923076922,-0.707692307692307,
-0.692307692307692,-0.676923076923076,-0.661538461538461,-0.646153846153846,
-0.63076923076923,-0.615384615384615,-0.6,-0.584615384615384,-0.569230769230769,
-0.553846153846154,-0.538461538461538,-0.523076923076923,-0.507692307692308,
-0.492307692307692,-0.476923076923077,-0.461538461538462,-0.446153846153846,
-0.430769230769231,-0.415384615384615,-0.4,-0.384615384615385,-0.369230769230769,
-0.353846153846154,-0.338461538461538,-0.323076923076923,-0.307692307692308,
-0.292307692307692,-0.276923076923077,-0.261538461538462,-0.246153846153846,
-0.230769230769231,-0.215384615384615,-0.2,-0.184615384615385,-0.169230769230769,
-0.153846153846154,-0.138461538461538,-0.123076923076923,-0.107692307692308,
-0.0923076923076923,-0.0769230769230769,-0.0615384615384615,-0.0461538461538462,
-0.0307692307692308,-0.0153846153846154,0.),(-1.,1.),.UNSPECIFIED.)
GEOMETRIC_REPRESENTATION_ITEM()
RATIONAL_B_SPLINE_SURFACE(((1.,1.),(1.,1.),(1.,1.),(1.,1.),(1.,1.),(1.,
1.),(1.,1.),(1.,1.),(1.,1.),(1.,1.),(1.,1.),(1.,1.),(1.,1.),(1.,1.),(1.,
1.),(1.,1.),(1.,1.),(1.,1.),(1.,1.),(1.,1.),(1.,1.),(1.,1.),(1.,1.),(1.,
1.),(1.,1.),(1.,1.),(1.,1.),(1.,1.),(1.,1.),(1.,1.),(1.,1.),(1.,1.),(1.,
1.),(1.,1.),(1.,1.),(1.,1.),(1.,1.),(1.,1.),(1.,1.),(1.,1.),(1.,1.),(1.,
1.),(1.,1.),(1.,1.),(1.,1.),(1.,1.),(1.,1.),(1.,1.),(1.,1.),(1.,1.),(1.,
1.),(1.,1.),(1.,1.),(1.,1.),(1.,1.),(1.,1.),(1.,1.),(1.,1.),(1.,1.),(1.,
1.),(1.,1.),(1.,1.),(1.,1.),(1.,1.),(1.,1.),(1.,1.),(1.,1.),(1.,1.),(1.,
1.),(1.,1.)))
REPRESENTATION_ITEM('')
SURFACE()
);
#34=(
BOUNDED_SURFACE()
B_SPLINE_SURFACE(5,1,((#28744,#28745),(#28746,#28747),(#28748,#28749),(#28750,
#28751),(#28752,#28753),(#28754,#28755),(#28756,#28757),(#28758,#28759),
(#28760,#28761),(#28762,#28763),(#28764,#28765),(#28766,#28767),(#28768,
#28769),(#28770,#28771),(#28772,#28773),(#28774,#28775),(#28776,#28777),
(#28778,#28779),(#28780,#28781),(#28782,#28783),(#28784,#28785),(#28786,
#28787),(#28788,#28789),(#28790,#28791),(#28792,#28793),(#28794,#28795),
(#28796,#28797),(#28798,#28799),(#28800,#28801),(#28802,#28803),(#28804,
#28805),(#28806,#28807),(#28808,#28809),(#28810,#28811),(#28812,#28813),
(#28814,#28815),(#28816,#28817),(#28818,#28819),(#28820,#28821),(#28822,
#28823),(#28824,#28825),(#28826,#28827),(#28828,#28829),(#28830,#28831),
(#28832,#28833),(#28834,#28835),(#28836,#28837),(#28838,#28839),(#28840,
#28841),(#28842,#28843),(#28844,#28845),(#28846,#28847),(#28848,#28849),
(#28850,#28851),(#28852,#28853),(#28854,#28855),(#28856,#28857),(#28858,
#28859),(#28860,#28861),(#28862,#28863),(#28864,#28865),(#28866,#28867),
(#28868,#28869),(#28870,#28871),(#28872,#28873),(#28874,#28875),(#28876,
#28877),(#28878,#28879),(#28880,#28881),(#28882,#28883)),.UNSPECIFIED.,
 .F.,.F.,.F.)
B_SPLINE_SURFACE_WITH_KNOTS((6,1,1,1,1,1,1,1,1,1,1,1,1,1,1,1,1,1,1,1,1,
1,1,1,1,1,1,1,1,1,1,1,1,1,1,1,1,1,1,1,1,1,1,1,1,1,1,1,1,1,1,1,1,1,1,1,1,
1,1,1,1,1,1,1,1,6),(2,2),(-1.,-0.984615384615383,-0.969230769230768,-0.953846153846152,
-0.938461538461537,-0.923076923076922,-0.907692307692306,-0.892307692307691,
-0.876923076923076,-0.86153846153846,-0.846153846153845,-0.83076923076923,
-0.815384615384614,-0.799999999999999,-0.784615384615384,-0.769230769230768,
-0.753846153846153,-0.738461538461538,-0.723076923076922,-0.707692307692307,
-0.692307692307692,-0.676923076923076,-0.661538461538461,-0.646153846153846,
-0.63076923076923,-0.615384615384615,-0.6,-0.584615384615384,-0.569230769230769,
-0.553846153846154,-0.538461538461538,-0.523076923076923,-0.507692307692308,
-0.492307692307692,-0.476923076923077,-0.461538461538462,-0.446153846153846,
-0.430769230769231,-0.415384615384615,-0.4,-0.384615384615385,-0.369230769230769,
-0.353846153846154,-0.338461538461538,-0.323076923076923,-0.307692307692308,
-0.292307692307692,-0.276923076923077,-0.261538461538462,-0.246153846153846,
-0.230769230769231,-0.215384615384615,-0.2,-0.184615384615385,-0.169230769230769,
-0.153846153846154,-0.138461538461538,-0.123076923076923,-0.107692307692308,
-0.0923076923076923,-0.0769230769230769,-0.0615384615384615,-0.0461538461538462,
-0.0307692307692308,-0.0153846153846154,0.),(-1.,1.),.UNSPECIFIED.)
GEOMETRIC_REPRESENTATION_ITEM()
RATIONAL_B_SPLINE_SURFACE(((1.,1.),(1.,1.),(1.,1.),(1.,1.),(1.,1.),(1.,
1.),(1.,1.),(1.,1.),(1.,1.),(1.,1.),(1.,1.),(1.,1.),(1.,1.),(1.,1.),(1.,
1.),(1.,1.),(1.,1.),(1.,1.),(1.,1.),(1.,1.),(1.,1.),(1.,1.),(1.,1.),(1.,
1.),(1.,1.),(1.,1.),(1.,1.),(1.,1.),(1.,1.),(1.,1.),(1.,1.),(1.,1.),(1.,
1.),(1.,1.),(1.,1.),(1.,1.),(1.,1.),(1.,1.),(1.,1.),(1.,1.),(1.,1.),(1.,
1.),(1.,1.),(1.,1.),(1.,1.),(1.,1.),(1.,1.),(1.,1.),(1.,1.),(1.,1.),(1.,
1.),(1.,1.),(1.,1.),(1.,1.),(1.,1.),(1.,1.),(1.,1.),(1.,1.),(1.,1.),(1.,
1.),(1.,1.),(1.,1.),(1.,1.),(1.,1.),(1.,1.),(1.,1.),(1.,1.),(1.,1.),(1.,
1.),(1.,1.)))
REPRESENTATION_ITEM('')
SURFACE()
);
#35=(
BOUNDED_SURFACE()
B_SPLINE_SURFACE(5,1,((#28960,#28961),(#28962,#28963),(#28964,#28965),(#28966,
#28967),(#28968,#28969),(#28970,#28971),(#28972,#28973),(#28974,#28975),
(#28976,#28977),(#28978,#28979),(#28980,#28981),(#28982,#28983),(#28984,
#28985),(#28986,#28987),(#28988,#28989),(#28990,#28991),(#28992,#28993),
(#28994,#28995),(#28996,#28997),(#28998,#28999),(#29000,#29001),(#29002,
#29003),(#29004,#29005),(#29006,#29007),(#29008,#29009),(#29010,#29011),
(#29012,#29013),(#29014,#29015),(#29016,#29017),(#29018,#29019),(#29020,
#29021),(#29022,#29023),(#29024,#29025),(#29026,#29027),(#29028,#29029),
(#29030,#29031),(#29032,#29033),(#29034,#29035),(#29036,#29037),(#29038,
#29039),(#29040,#29041),(#29042,#29043),(#29044,#29045),(#29046,#29047),
(#29048,#29049),(#29050,#29051),(#29052,#29053),(#29054,#29055),(#29056,
#29057),(#29058,#29059),(#29060,#29061),(#29062,#29063),(#29064,#29065),
(#29066,#29067),(#29068,#29069),(#29070,#29071),(#29072,#29073),(#29074,
#29075),(#29076,#29077),(#29078,#29079),(#29080,#29081),(#29082,#29083),
(#29084,#29085),(#29086,#29087),(#29088,#29089),(#29090,#29091),(#29092,
#29093),(#29094,#29095),(#29096,#29097),(#29098,#29099)),.UNSPECIFIED.,
 .F.,.F.,.F.)
B_SPLINE_SURFACE_WITH_KNOTS((6,1,1,1,1,1,1,1,1,1,1,1,1,1,1,1,1,1,1,1,1,
1,1,1,1,1,1,1,1,1,1,1,1,1,1,1,1,1,1,1,1,1,1,1,1,1,1,1,1,1,1,1,1,1,1,1,1,
1,1,1,1,1,1,1,1,6),(2,2),(-1.,-0.984615384615383,-0.969230769230768,-0.953846153846152,
-0.938461538461537,-0.923076923076922,-0.907692307692306,-0.892307692307691,
-0.876923076923076,-0.86153846153846,-0.846153846153845,-0.83076923076923,
-0.815384615384614,-0.799999999999999,-0.784615384615384,-0.769230769230768,
-0.753846153846153,-0.738461538461538,-0.723076923076922,-0.707692307692307,
-0.692307692307692,-0.676923076923076,-0.661538461538461,-0.646153846153846,
-0.63076923076923,-0.615384615384615,-0.6,-0.584615384615384,-0.569230769230769,
-0.553846153846154,-0.538461538461538,-0.523076923076923,-0.507692307692308,
-0.492307692307692,-0.476923076923077,-0.461538461538462,-0.446153846153846,
-0.430769230769231,-0.415384615384615,-0.4,-0.384615384615385,-0.369230769230769,
-0.353846153846154,-0.338461538461538,-0.323076923076923,-0.307692307692308,
-0.292307692307692,-0.276923076923077,-0.261538461538462,-0.246153846153846,
-0.230769230769231,-0.215384615384615,-0.2,-0.184615384615385,-0.169230769230769,
-0.153846153846154,-0.138461538461538,-0.123076923076923,-0.107692307692308,
-0.0923076923076923,-0.0769230769230769,-0.0615384615384615,-0.0461538461538462,
-0.0307692307692308,-0.0153846153846154,0.),(-1.,1.),.UNSPECIFIED.)
GEOMETRIC_REPRESENTATION_ITEM()
RATIONAL_B_SPLINE_SURFACE(((1.,1.),(1.,1.),(1.,1.),(1.,1.),(1.,1.),(1.,
1.),(1.,1.),(1.,1.),(1.,1.),(1.,1.),(1.,1.),(1.,1.),(1.,1.),(1.,1.),(1.,
1.),(1.,1.),(1.,1.),(1.,1.),(1.,1.),(1.,1.),(1.,1.),(1.,1.),(1.,1.),(1.,
1.),(1.,1.),(1.,1.),(1.,1.),(1.,1.),(1.,1.),(1.,1.),(1.,1.),(1.,1.),(1.,
1.),(1.,1.),(1.,1.),(1.,1.),(1.,1.),(1.,1.),(1.,1.),(1.,1.),(1.,1.),(1.,
1.),(1.,1.),(1.,1.),(1.,1.),(1.,1.),(1.,1.),(1.,1.),(1.,1.),(1.,1.),(1.,
1.),(1.,1.),(1.,1.),(1.,1.),(1.,1.),(1.,1.),(1.,1.),(1.,1.),(1.,1.),(1.,
1.),(1.,1.),(1.,1.),(1.,1.),(1.,1.),(1.,1.),(1.,1.),(1.,1.),(1.,1.),(1.,
1.),(1.,1.)))
REPRESENTATION_ITEM('')
SURFACE()
);
#36=(
BOUNDED_SURFACE()
B_SPLINE_SURFACE(5,1,((#29176,#29177),(#29178,#29179),(#29180,#29181),(#29182,
#29183),(#29184,#29185),(#29186,#29187),(#29188,#29189),(#29190,#29191),
(#29192,#29193),(#29194,#29195),(#29196,#29197),(#29198,#29199),(#29200,
#29201),(#29202,#29203),(#29204,#29205),(#29206,#29207),(#29208,#29209),
(#29210,#29211),(#29212,#29213),(#29214,#29215),(#29216,#29217),(#29218,
#29219),(#29220,#29221),(#29222,#29223),(#29224,#29225),(#29226,#29227),
(#29228,#29229),(#29230,#29231),(#29232,#29233),(#29234,#29235),(#29236,
#29237),(#29238,#29239),(#29240,#29241),(#29242,#29243),(#29244,#29245),
(#29246,#29247),(#29248,#29249),(#29250,#29251),(#29252,#29253),(#29254,
#29255),(#29256,#29257),(#29258,#29259),(#29260,#29261),(#29262,#29263),
(#29264,#29265),(#29266,#29267),(#29268,#29269),(#29270,#29271),(#29272,
#29273),(#29274,#29275),(#29276,#29277),(#29278,#29279),(#29280,#29281),
(#29282,#29283),(#29284,#29285),(#29286,#29287),(#29288,#29289),(#29290,
#29291),(#29292,#29293),(#29294,#29295),(#29296,#29297),(#29298,#29299),
(#29300,#29301),(#29302,#29303),(#29304,#29305),(#29306,#29307),(#29308,
#29309),(#29310,#29311),(#29312,#29313),(#29314,#29315)),.UNSPECIFIED.,
 .F.,.F.,.F.)
B_SPLINE_SURFACE_WITH_KNOTS((6,1,1,1,1,1,1,1,1,1,1,1,1,1,1,1,1,1,1,1,1,
1,1,1,1,1,1,1,1,1,1,1,1,1,1,1,1,1,1,1,1,1,1,1,1,1,1,1,1,1,1,1,1,1,1,1,1,
1,1,1,1,1,1,1,1,6),(2,2),(-1.,-0.984615384615383,-0.969230769230768,-0.953846153846152,
-0.938461538461537,-0.923076923076922,-0.907692307692306,-0.892307692307691,
-0.876923076923076,-0.86153846153846,-0.846153846153845,-0.83076923076923,
-0.815384615384614,-0.799999999999999,-0.784615384615384,-0.769230769230768,
-0.753846153846153,-0.738461538461538,-0.723076923076922,-0.707692307692307,
-0.692307692307692,-0.676923076923076,-0.661538461538461,-0.646153846153846,
-0.63076923076923,-0.615384615384615,-0.6,-0.584615384615384,-0.569230769230769,
-0.553846153846154,-0.538461538461538,-0.523076923076923,-0.507692307692308,
-0.492307692307692,-0.476923076923077,-0.461538461538462,-0.446153846153846,
-0.430769230769231,-0.415384615384615,-0.4,-0.384615384615385,-0.369230769230769,
-0.353846153846154,-0.338461538461538,-0.323076923076923,-0.307692307692308,
-0.292307692307692,-0.276923076923077,-0.261538461538462,-0.246153846153846,
-0.230769230769231,-0.215384615384615,-0.2,-0.184615384615385,-0.169230769230769,
-0.153846153846154,-0.138461538461538,-0.123076923076923,-0.107692307692308,
-0.0923076923076923,-0.0769230769230769,-0.0615384615384615,-0.0461538461538462,
-0.0307692307692308,-0.0153846153846154,0.),(-1.,1.),.UNSPECIFIED.)
GEOMETRIC_REPRESENTATION_ITEM()
RATIONAL_B_SPLINE_SURFACE(((1.,1.),(1.,1.),(1.,1.),(1.,1.),(1.,1.),(1.,
1.),(1.,1.),(1.,1.),(1.,1.),(1.,1.),(1.,1.),(1.,1.),(1.,1.),(1.,1.),(1.,
1.),(1.,1.),(1.,1.),(1.,1.),(1.,1.),(1.,1.),(1.,1.),(1.,1.),(1.,1.),(1.,
1.),(1.,1.),(1.,1.),(1.,1.),(1.,1.),(1.,1.),(1.,1.),(1.,1.),(1.,1.),(1.,
1.),(1.,1.),(1.,1.),(1.,1.),(1.,1.),(1.,1.),(1.,1.),(1.,1.),(1.,1.),(1.,
1.),(1.,1.),(1.,1.),(1.,1.),(1.,1.),(1.,1.),(1.,1.),(1.,1.),(1.,1.),(1.,
1.),(1.,1.),(1.,1.),(1.,1.),(1.,1.),(1.,1.),(1.,1.),(1.,1.),(1.,1.),(1.,
1.),(1.,1.),(1.,1.),(1.,1.),(1.,1.),(1.,1.),(1.,1.),(1.,1.),(1.,1.),(1.,
1.),(1.,1.)))
REPRESENTATION_ITEM('')
SURFACE()
);
#37=(
BOUNDED_SURFACE()
B_SPLINE_SURFACE(5,1,((#29392,#29393),(#29394,#29395),(#29396,#29397),(#29398,
#29399),(#29400,#29401),(#29402,#29403),(#29404,#29405),(#29406,#29407),
(#29408,#29409),(#29410,#29411),(#29412,#29413),(#29414,#29415),(#29416,
#29417),(#29418,#29419),(#29420,#29421),(#29422,#29423),(#29424,#29425),
(#29426,#29427),(#29428,#29429),(#29430,#29431),(#29432,#29433),(#29434,
#29435),(#29436,#29437),(#29438,#29439),(#29440,#29441),(#29442,#29443),
(#29444,#29445),(#29446,#29447),(#29448,#29449),(#29450,#29451),(#29452,
#29453),(#29454,#29455),(#29456,#29457),(#29458,#29459),(#29460,#29461),
(#29462,#29463),(#29464,#29465),(#29466,#29467),(#29468,#29469),(#29470,
#29471),(#29472,#29473),(#29474,#29475),(#29476,#29477),(#29478,#29479),
(#29480,#29481),(#29482,#29483),(#29484,#29485),(#29486,#29487),(#29488,
#29489),(#29490,#29491),(#29492,#29493),(#29494,#29495),(#29496,#29497),
(#29498,#29499),(#29500,#29501),(#29502,#29503),(#29504,#29505),(#29506,
#29507),(#29508,#29509),(#29510,#29511),(#29512,#29513),(#29514,#29515),
(#29516,#29517),(#29518,#29519),(#29520,#29521),(#29522,#29523),(#29524,
#29525),(#29526,#29527),(#29528,#29529),(#29530,#29531)),.UNSPECIFIED.,
 .F.,.F.,.F.)
B_SPLINE_SURFACE_WITH_KNOTS((6,1,1,1,1,1,1,1,1,1,1,1,1,1,1,1,1,1,1,1,1,
1,1,1,1,1,1,1,1,1,1,1,1,1,1,1,1,1,1,1,1,1,1,1,1,1,1,1,1,1,1,1,1,1,1,1,1,
1,1,1,1,1,1,1,1,6),(2,2),(-1.,-0.984615384615383,-0.969230769230768,-0.953846153846152,
-0.938461538461537,-0.923076923076922,-0.907692307692306,-0.892307692307691,
-0.876923076923076,-0.86153846153846,-0.846153846153845,-0.83076923076923,
-0.815384615384614,-0.799999999999999,-0.784615384615384,-0.769230769230768,
-0.753846153846153,-0.738461538461538,-0.723076923076922,-0.707692307692307,
-0.692307692307692,-0.676923076923076,-0.661538461538461,-0.646153846153846,
-0.63076923076923,-0.615384615384615,-0.6,-0.584615384615384,-0.569230769230769,
-0.553846153846154,-0.538461538461538,-0.523076923076923,-0.507692307692308,
-0.492307692307692,-0.476923076923077,-0.461538461538462,-0.446153846153846,
-0.430769230769231,-0.415384615384615,-0.4,-0.384615384615385,-0.369230769230769,
-0.353846153846154,-0.338461538461538,-0.323076923076923,-0.307692307692308,
-0.292307692307692,-0.276923076923077,-0.261538461538462,-0.246153846153846,
-0.230769230769231,-0.215384615384615,-0.2,-0.184615384615385,-0.169230769230769,
-0.153846153846154,-0.138461538461538,-0.123076923076923,-0.107692307692308,
-0.0923076923076923,-0.0769230769230769,-0.0615384615384615,-0.0461538461538462,
-0.0307692307692308,-0.0153846153846154,0.),(-1.,1.),.UNSPECIFIED.)
GEOMETRIC_REPRESENTATION_ITEM()
RATIONAL_B_SPLINE_SURFACE(((1.,1.),(1.,1.),(1.,1.),(1.,1.),(1.,1.),(1.,
1.),(1.,1.),(1.,1.),(1.,1.),(1.,1.),(1.,1.),(1.,1.),(1.,1.),(1.,1.),(1.,
1.),(1.,1.),(1.,1.),(1.,1.),(1.,1.),(1.,1.),(1.,1.),(1.,1.),(1.,1.),(1.,
1.),(1.,1.),(1.,1.),(1.,1.),(1.,1.),(1.,1.),(1.,1.),(1.,1.),(1.,1.),(1.,
1.),(1.,1.),(1.,1.),(1.,1.),(1.,1.),(1.,1.),(1.,1.),(1.,1.),(1.,1.),(1.,
1.),(1.,1.),(1.,1.),(1.,1.),(1.,1.),(1.,1.),(1.,1.),(1.,1.),(1.,1.),(1.,
1.),(1.,1.),(1.,1.),(1.,1.),(1.,1.),(1.,1.),(1.,1.),(1.,1.),(1.,1.),(1.,
1.),(1.,1.),(1.,1.),(1.,1.),(1.,1.),(1.,1.),(1.,1.),(1.,1.),(1.,1.),(1.,
1.),(1.,1.)))
REPRESENTATION_ITEM('')
SURFACE()
);
#38=(
BOUNDED_SURFACE()
B_SPLINE_SURFACE(5,1,((#29608,#29609),(#29610,#29611),(#29612,#29613),(#29614,
#29615),(#29616,#29617),(#29618,#29619),(#29620,#29621),(#29622,#29623),
(#29624,#29625),(#29626,#29627),(#29628,#29629),(#29630,#29631),(#29632,
#29633),(#29634,#29635),(#29636,#29637),(#29638,#29639),(#29640,#29641),
(#29642,#29643),(#29644,#29645),(#29646,#29647),(#29648,#29649),(#29650,
#29651),(#29652,#29653),(#29654,#29655),(#29656,#29657),(#29658,#29659),
(#29660,#29661),(#29662,#29663),(#29664,#29665),(#29666,#29667),(#29668,
#29669),(#29670,#29671),(#29672,#29673),(#29674,#29675),(#29676,#29677),
(#29678,#29679),(#29680,#29681),(#29682,#29683),(#29684,#29685),(#29686,
#29687),(#29688,#29689),(#29690,#29691),(#29692,#29693),(#29694,#29695),
(#29696,#29697),(#29698,#29699),(#29700,#29701),(#29702,#29703),(#29704,
#29705),(#29706,#29707),(#29708,#29709),(#29710,#29711),(#29712,#29713),
(#29714,#29715),(#29716,#29717),(#29718,#29719),(#29720,#29721),(#29722,
#29723),(#29724,#29725),(#29726,#29727),(#29728,#29729),(#29730,#29731),
(#29732,#29733),(#29734,#29735),(#29736,#29737),(#29738,#29739),(#29740,
#29741),(#29742,#29743),(#29744,#29745),(#29746,#29747)),.UNSPECIFIED.,
 .F.,.F.,.F.)
B_SPLINE_SURFACE_WITH_KNOTS((6,1,1,1,1,1,1,1,1,1,1,1,1,1,1,1,1,1,1,1,1,
1,1,1,1,1,1,1,1,1,1,1,1,1,1,1,1,1,1,1,1,1,1,1,1,1,1,1,1,1,1,1,1,1,1,1,1,
1,1,1,1,1,1,1,1,6),(2,2),(-1.,-0.984615384615383,-0.969230769230768,-0.953846153846152,
-0.938461538461537,-0.923076923076922,-0.907692307692306,-0.892307692307691,
-0.876923076923076,-0.86153846153846,-0.846153846153845,-0.83076923076923,
-0.815384615384614,-0.799999999999999,-0.784615384615384,-0.769230769230768,
-0.753846153846153,-0.738461538461538,-0.723076923076922,-0.707692307692307,
-0.692307692307692,-0.676923076923076,-0.661538461538461,-0.646153846153846,
-0.63076923076923,-0.615384615384615,-0.6,-0.584615384615384,-0.569230769230769,
-0.553846153846154,-0.538461538461538,-0.523076923076923,-0.507692307692308,
-0.492307692307692,-0.476923076923077,-0.461538461538462,-0.446153846153846,
-0.430769230769231,-0.415384615384615,-0.4,-0.384615384615385,-0.369230769230769,
-0.353846153846154,-0.338461538461538,-0.323076923076923,-0.307692307692308,
-0.292307692307692,-0.276923076923077,-0.261538461538462,-0.246153846153846,
-0.230769230769231,-0.215384615384615,-0.2,-0.184615384615385,-0.169230769230769,
-0.153846153846154,-0.138461538461538,-0.123076923076923,-0.107692307692308,
-0.0923076923076923,-0.0769230769230769,-0.0615384615384615,-0.0461538461538462,
-0.0307692307692308,-0.0153846153846154,0.),(-1.,1.),.UNSPECIFIED.)
GEOMETRIC_REPRESENTATION_ITEM()
RATIONAL_B_SPLINE_SURFACE(((1.,1.),(1.,1.),(1.,1.),(1.,1.),(1.,1.),(1.,
1.),(1.,1.),(1.,1.),(1.,1.),(1.,1.),(1.,1.),(1.,1.),(1.,1.),(1.,1.),(1.,
1.),(1.,1.),(1.,1.),(1.,1.),(1.,1.),(1.,1.),(1.,1.),(1.,1.),(1.,1.),(1.,
1.),(1.,1.),(1.,1.),(1.,1.),(1.,1.),(1.,1.),(1.,1.),(1.,1.),(1.,1.),(1.,
1.),(1.,1.),(1.,1.),(1.,1.),(1.,1.),(1.,1.),(1.,1.),(1.,1.),(1.,1.),(1.,
1.),(1.,1.),(1.,1.),(1.,1.),(1.,1.),(1.,1.),(1.,1.),(1.,1.),(1.,1.),(1.,
1.),(1.,1.),(1.,1.),(1.,1.),(1.,1.),(1.,1.),(1.,1.),(1.,1.),(1.,1.),(1.,
1.),(1.,1.),(1.,1.),(1.,1.),(1.,1.),(1.,1.),(1.,1.),(1.,1.),(1.,1.),(1.,
1.),(1.,1.)))
REPRESENTATION_ITEM('')
SURFACE()
);
#39=(
BOUNDED_SURFACE()
B_SPLINE_SURFACE(5,1,((#29824,#29825),(#29826,#29827),(#29828,#29829),(#29830,
#29831),(#29832,#29833),(#29834,#29835),(#29836,#29837),(#29838,#29839),
(#29840,#29841),(#29842,#29843),(#29844,#29845),(#29846,#29847),(#29848,
#29849),(#29850,#29851),(#29852,#29853),(#29854,#29855),(#29856,#29857),
(#29858,#29859),(#29860,#29861),(#29862,#29863),(#29864,#29865),(#29866,
#29867),(#29868,#29869),(#29870,#29871),(#29872,#29873),(#29874,#29875),
(#29876,#29877),(#29878,#29879),(#29880,#29881),(#29882,#29883),(#29884,
#29885),(#29886,#29887),(#29888,#29889),(#29890,#29891),(#29892,#29893),
(#29894,#29895),(#29896,#29897),(#29898,#29899),(#29900,#29901),(#29902,
#29903),(#29904,#29905),(#29906,#29907),(#29908,#29909),(#29910,#29911),
(#29912,#29913),(#29914,#29915),(#29916,#29917),(#29918,#29919),(#29920,
#29921),(#29922,#29923),(#29924,#29925),(#29926,#29927),(#29928,#29929),
(#29930,#29931),(#29932,#29933),(#29934,#29935),(#29936,#29937),(#29938,
#29939),(#29940,#29941),(#29942,#29943),(#29944,#29945),(#29946,#29947),
(#29948,#29949),(#29950,#29951),(#29952,#29953),(#29954,#29955),(#29956,
#29957),(#29958,#29959),(#29960,#29961),(#29962,#29963)),.UNSPECIFIED.,
 .F.,.F.,.F.)
B_SPLINE_SURFACE_WITH_KNOTS((6,1,1,1,1,1,1,1,1,1,1,1,1,1,1,1,1,1,1,1,1,
1,1,1,1,1,1,1,1,1,1,1,1,1,1,1,1,1,1,1,1,1,1,1,1,1,1,1,1,1,1,1,1,1,1,1,1,
1,1,1,1,1,1,1,1,6),(2,2),(-1.,-0.984615384615383,-0.969230769230768,-0.953846153846152,
-0.938461538461537,-0.923076923076922,-0.907692307692306,-0.892307692307691,
-0.876923076923076,-0.86153846153846,-0.846153846153845,-0.83076923076923,
-0.815384615384614,-0.799999999999999,-0.784615384615384,-0.769230769230768,
-0.753846153846153,-0.738461538461538,-0.723076923076922,-0.707692307692307,
-0.692307692307692,-0.676923076923076,-0.661538461538461,-0.646153846153846,
-0.63076923076923,-0.615384615384615,-0.6,-0.584615384615384,-0.569230769230769,
-0.553846153846154,-0.538461538461538,-0.523076923076923,-0.507692307692308,
-0.492307692307692,-0.476923076923077,-0.461538461538462,-0.446153846153846,
-0.430769230769231,-0.415384615384615,-0.4,-0.384615384615385,-0.369230769230769,
-0.353846153846154,-0.338461538461538,-0.323076923076923,-0.307692307692308,
-0.292307692307692,-0.276923076923077,-0.261538461538462,-0.246153846153846,
-0.230769230769231,-0.215384615384615,-0.2,-0.184615384615385,-0.169230769230769,
-0.153846153846154,-0.138461538461538,-0.123076923076923,-0.107692307692308,
-0.0923076923076923,-0.0769230769230769,-0.0615384615384615,-0.0461538461538462,
-0.0307692307692308,-0.0153846153846154,0.),(-1.,1.),.UNSPECIFIED.)
GEOMETRIC_REPRESENTATION_ITEM()
RATIONAL_B_SPLINE_SURFACE(((1.,1.),(1.,1.),(1.,1.),(1.,1.),(1.,1.),(1.,
1.),(1.,1.),(1.,1.),(1.,1.),(1.,1.),(1.,1.),(1.,1.),(1.,1.),(1.,1.),(1.,
1.),(1.,1.),(1.,1.),(1.,1.),(1.,1.),(1.,1.),(1.,1.),(1.,1.),(1.,1.),(1.,
1.),(1.,1.),(1.,1.),(1.,1.),(1.,1.),(1.,1.),(1.,1.),(1.,1.),(1.,1.),(1.,
1.),(1.,1.),(1.,1.),(1.,1.),(1.,1.),(1.,1.),(1.,1.),(1.,1.),(1.,1.),(1.,
1.),(1.,1.),(1.,1.),(1.,1.),(1.,1.),(1.,1.),(1.,1.),(1.,1.),(1.,1.),(1.,
1.),(1.,1.),(1.,1.),(1.,1.),(1.,1.),(1.,1.),(1.,1.),(1.,1.),(1.,1.),(1.,
1.),(1.,1.),(1.,1.),(1.,1.),(1.,1.),(1.,1.),(1.,1.),(1.,1.),(1.,1.),(1.,
1.),(1.,1.)))
REPRESENTATION_ITEM('')
SURFACE()
);
#40=(
BOUNDED_SURFACE()
B_SPLINE_SURFACE(5,1,((#30040,#30041),(#30042,#30043),(#30044,#30045),(#30046,
#30047),(#30048,#30049),(#30050,#30051),(#30052,#30053),(#30054,#30055),
(#30056,#30057),(#30058,#30059),(#30060,#30061),(#30062,#30063),(#30064,
#30065),(#30066,#30067),(#30068,#30069),(#30070,#30071),(#30072,#30073),
(#30074,#30075),(#30076,#30077),(#30078,#30079),(#30080,#30081),(#30082,
#30083),(#30084,#30085),(#30086,#30087),(#30088,#30089),(#30090,#30091),
(#30092,#30093),(#30094,#30095),(#30096,#30097),(#30098,#30099),(#30100,
#30101),(#30102,#30103),(#30104,#30105),(#30106,#30107),(#30108,#30109),
(#30110,#30111),(#30112,#30113),(#30114,#30115),(#30116,#30117),(#30118,
#30119),(#30120,#30121),(#30122,#30123),(#30124,#30125),(#30126,#30127),
(#30128,#30129),(#30130,#30131),(#30132,#30133),(#30134,#30135),(#30136,
#30137),(#30138,#30139),(#30140,#30141),(#30142,#30143),(#30144,#30145),
(#30146,#30147),(#30148,#30149),(#30150,#30151),(#30152,#30153),(#30154,
#30155),(#30156,#30157),(#30158,#30159),(#30160,#30161),(#30162,#30163),
(#30164,#30165),(#30166,#30167),(#30168,#30169),(#30170,#30171),(#30172,
#30173),(#30174,#30175),(#30176,#30177),(#30178,#30179)),.UNSPECIFIED.,
 .F.,.F.,.F.)
B_SPLINE_SURFACE_WITH_KNOTS((6,1,1,1,1,1,1,1,1,1,1,1,1,1,1,1,1,1,1,1,1,
1,1,1,1,1,1,1,1,1,1,1,1,1,1,1,1,1,1,1,1,1,1,1,1,1,1,1,1,1,1,1,1,1,1,1,1,
1,1,1,1,1,1,1,1,6),(2,2),(-1.,-0.984615384615383,-0.969230769230768,-0.953846153846152,
-0.938461538461537,-0.923076923076922,-0.907692307692306,-0.892307692307691,
-0.876923076923076,-0.86153846153846,-0.846153846153845,-0.83076923076923,
-0.815384615384614,-0.799999999999999,-0.784615384615384,-0.769230769230768,
-0.753846153846153,-0.738461538461538,-0.723076923076922,-0.707692307692307,
-0.692307692307692,-0.676923076923076,-0.661538461538461,-0.646153846153846,
-0.63076923076923,-0.615384615384615,-0.6,-0.584615384615384,-0.569230769230769,
-0.553846153846154,-0.538461538461538,-0.523076923076923,-0.507692307692308,
-0.492307692307692,-0.476923076923077,-0.461538461538462,-0.446153846153846,
-0.430769230769231,-0.415384615384615,-0.4,-0.384615384615385,-0.369230769230769,
-0.353846153846154,-0.338461538461538,-0.323076923076923,-0.307692307692308,
-0.292307692307692,-0.276923076923077,-0.261538461538462,-0.246153846153846,
-0.230769230769231,-0.215384615384615,-0.2,-0.184615384615385,-0.169230769230769,
-0.153846153846154,-0.138461538461538,-0.123076923076923,-0.107692307692308,
-0.0923076923076923,-0.0769230769230769,-0.0615384615384615,-0.0461538461538462,
-0.0307692307692308,-0.0153846153846154,0.),(-1.,1.),.UNSPECIFIED.)
GEOMETRIC_REPRESENTATION_ITEM()
RATIONAL_B_SPLINE_SURFACE(((1.,1.),(1.,1.),(1.,1.),(1.,1.),(1.,1.),(1.,
1.),(1.,1.),(1.,1.),(1.,1.),(1.,1.),(1.,1.),(1.,1.),(1.,1.),(1.,1.),(1.,
1.),(1.,1.),(1.,1.),(1.,1.),(1.,1.),(1.,1.),(1.,1.),(1.,1.),(1.,1.),(1.,
1.),(1.,1.),(1.,1.),(1.,1.),(1.,1.),(1.,1.),(1.,1.),(1.,1.),(1.,1.),(1.,
1.),(1.,1.),(1.,1.),(1.,1.),(1.,1.),(1.,1.),(1.,1.),(1.,1.),(1.,1.),(1.,
1.),(1.,1.),(1.,1.),(1.,1.),(1.,1.),(1.,1.),(1.,1.),(1.,1.),(1.,1.),(1.,
1.),(1.,1.),(1.,1.),(1.,1.),(1.,1.),(1.,1.),(1.,1.),(1.,1.),(1.,1.),(1.,
1.),(1.,1.),(1.,1.),(1.,1.),(1.,1.),(1.,1.),(1.,1.),(1.,1.),(1.,1.),(1.,
1.),(1.,1.)))
REPRESENTATION_ITEM('')
SURFACE()
);
#41=(
BOUNDED_SURFACE()
B_SPLINE_SURFACE(5,1,((#30256,#30257),(#30258,#30259),(#30260,#30261),(#30262,
#30263),(#30264,#30265),(#30266,#30267),(#30268,#30269),(#30270,#30271),
(#30272,#30273),(#30274,#30275),(#30276,#30277),(#30278,#30279),(#30280,
#30281),(#30282,#30283),(#30284,#30285),(#30286,#30287),(#30288,#30289),
(#30290,#30291),(#30292,#30293),(#30294,#30295),(#30296,#30297),(#30298,
#30299),(#30300,#30301),(#30302,#30303),(#30304,#30305),(#30306,#30307),
(#30308,#30309),(#30310,#30311),(#30312,#30313),(#30314,#30315),(#30316,
#30317),(#30318,#30319),(#30320,#30321),(#30322,#30323),(#30324,#30325),
(#30326,#30327),(#30328,#30329),(#30330,#30331),(#30332,#30333),(#30334,
#30335),(#30336,#30337),(#30338,#30339),(#30340,#30341),(#30342,#30343),
(#30344,#30345),(#30346,#30347),(#30348,#30349),(#30350,#30351),(#30352,
#30353),(#30354,#30355),(#30356,#30357),(#30358,#30359),(#30360,#30361),
(#30362,#30363),(#30364,#30365),(#30366,#30367),(#30368,#30369),(#30370,
#30371),(#30372,#30373),(#30374,#30375),(#30376,#30377),(#30378,#30379),
(#30380,#30381),(#30382,#30383),(#30384,#30385),(#30386,#30387),(#30388,
#30389),(#30390,#30391),(#30392,#30393),(#30394,#30395)),.UNSPECIFIED.,
 .F.,.F.,.F.)
B_SPLINE_SURFACE_WITH_KNOTS((6,1,1,1,1,1,1,1,1,1,1,1,1,1,1,1,1,1,1,1,1,
1,1,1,1,1,1,1,1,1,1,1,1,1,1,1,1,1,1,1,1,1,1,1,1,1,1,1,1,1,1,1,1,1,1,1,1,
1,1,1,1,1,1,1,1,6),(2,2),(-1.,-0.984615384615383,-0.969230769230768,-0.953846153846152,
-0.938461538461537,-0.923076923076922,-0.907692307692306,-0.892307692307691,
-0.876923076923076,-0.86153846153846,-0.846153846153845,-0.83076923076923,
-0.815384615384614,-0.799999999999999,-0.784615384615384,-0.769230769230768,
-0.753846153846153,-0.738461538461538,-0.723076923076922,-0.707692307692307,
-0.692307692307692,-0.676923076923076,-0.661538461538461,-0.646153846153846,
-0.63076923076923,-0.615384615384615,-0.6,-0.584615384615384,-0.569230769230769,
-0.553846153846154,-0.538461538461538,-0.523076923076923,-0.507692307692308,
-0.492307692307692,-0.476923076923077,-0.461538461538462,-0.446153846153846,
-0.430769230769231,-0.415384615384615,-0.4,-0.384615384615385,-0.369230769230769,
-0.353846153846154,-0.338461538461538,-0.323076923076923,-0.307692307692308,
-0.292307692307692,-0.276923076923077,-0.261538461538462,-0.246153846153846,
-0.230769230769231,-0.215384615384615,-0.2,-0.184615384615385,-0.169230769230769,
-0.153846153846154,-0.138461538461538,-0.123076923076923,-0.107692307692308,
-0.0923076923076923,-0.0769230769230769,-0.0615384615384615,-0.0461538461538462,
-0.0307692307692308,-0.0153846153846154,0.),(-1.,1.),.UNSPECIFIED.)
GEOMETRIC_REPRESENTATION_ITEM()
RATIONAL_B_SPLINE_SURFACE(((1.,1.),(1.,1.),(1.,1.),(1.,1.),(1.,1.),(1.,
1.),(1.,1.),(1.,1.),(1.,1.),(1.,1.),(1.,1.),(1.,1.),(1.,1.),(1.,1.),(1.,
1.),(1.,1.),(1.,1.),(1.,1.),(1.,1.),(1.,1.),(1.,1.),(1.,1.),(1.,1.),(1.,
1.),(1.,1.),(1.,1.),(1.,1.),(1.,1.),(1.,1.),(1.,1.),(1.,1.),(1.,1.),(1.,
1.),(1.,1.),(1.,1.),(1.,1.),(1.,1.),(1.,1.),(1.,1.),(1.,1.),(1.,1.),(1.,
1.),(1.,1.),(1.,1.),(1.,1.),(1.,1.),(1.,1.),(1.,1.),(1.,1.),(1.,1.),(1.,
1.),(1.,1.),(1.,1.),(1.,1.),(1.,1.),(1.,1.),(1.,1.),(1.,1.),(1.,1.),(1.,
1.),(1.,1.),(1.,1.),(1.,1.),(1.,1.),(1.,1.),(1.,1.),(1.,1.),(1.,1.),(1.,
1.),(1.,1.)))
REPRESENTATION_ITEM('')
SURFACE()
);
#42=(
BOUNDED_SURFACE()
B_SPLINE_SURFACE(5,1,((#30472,#30473),(#30474,#30475),(#30476,#30477),(#30478,
#30479),(#30480,#30481),(#30482,#30483),(#30484,#30485),(#30486,#30487),
(#30488,#30489),(#30490,#30491),(#30492,#30493),(#30494,#30495),(#30496,
#30497),(#30498,#30499),(#30500,#30501),(#30502,#30503),(#30504,#30505),
(#30506,#30507),(#30508,#30509),(#30510,#30511),(#30512,#30513),(#30514,
#30515),(#30516,#30517),(#30518,#30519),(#30520,#30521),(#30522,#30523),
(#30524,#30525),(#30526,#30527),(#30528,#30529),(#30530,#30531),(#30532,
#30533),(#30534,#30535),(#30536,#30537),(#30538,#30539),(#30540,#30541),
(#30542,#30543),(#30544,#30545),(#30546,#30547),(#30548,#30549),(#30550,
#30551),(#30552,#30553),(#30554,#30555),(#30556,#30557),(#30558,#30559),
(#30560,#30561),(#30562,#30563),(#30564,#30565),(#30566,#30567),(#30568,
#30569),(#30570,#30571),(#30572,#30573),(#30574,#30575),(#30576,#30577),
(#30578,#30579),(#30580,#30581),(#30582,#30583),(#30584,#30585),(#30586,
#30587),(#30588,#30589),(#30590,#30591),(#30592,#30593),(#30594,#30595),
(#30596,#30597),(#30598,#30599),(#30600,#30601),(#30602,#30603),(#30604,
#30605),(#30606,#30607),(#30608,#30609),(#30610,#30611)),.UNSPECIFIED.,
 .F.,.F.,.F.)
B_SPLINE_SURFACE_WITH_KNOTS((6,1,1,1,1,1,1,1,1,1,1,1,1,1,1,1,1,1,1,1,1,
1,1,1,1,1,1,1,1,1,1,1,1,1,1,1,1,1,1,1,1,1,1,1,1,1,1,1,1,1,1,1,1,1,1,1,1,
1,1,1,1,1,1,1,1,6),(2,2),(-1.,-0.984615384615383,-0.969230769230768,-0.953846153846152,
-0.938461538461537,-0.923076923076922,-0.907692307692306,-0.892307692307691,
-0.876923076923076,-0.86153846153846,-0.846153846153845,-0.83076923076923,
-0.815384615384614,-0.799999999999999,-0.784615384615384,-0.769230769230768,
-0.753846153846153,-0.738461538461538,-0.723076923076922,-0.707692307692307,
-0.692307692307692,-0.676923076923076,-0.661538461538461,-0.646153846153846,
-0.63076923076923,-0.615384615384615,-0.6,-0.584615384615384,-0.569230769230769,
-0.553846153846154,-0.538461538461538,-0.523076923076923,-0.507692307692308,
-0.492307692307692,-0.476923076923077,-0.461538461538462,-0.446153846153846,
-0.430769230769231,-0.415384615384615,-0.4,-0.384615384615385,-0.369230769230769,
-0.353846153846154,-0.338461538461538,-0.323076923076923,-0.307692307692308,
-0.292307692307692,-0.276923076923077,-0.261538461538462,-0.246153846153846,
-0.230769230769231,-0.215384615384615,-0.2,-0.184615384615385,-0.169230769230769,
-0.153846153846154,-0.138461538461538,-0.123076923076923,-0.107692307692308,
-0.0923076923076923,-0.0769230769230769,-0.0615384615384615,-0.0461538461538462,
-0.0307692307692308,-0.0153846153846154,0.),(-1.,1.),.UNSPECIFIED.)
GEOMETRIC_REPRESENTATION_ITEM()
RATIONAL_B_SPLINE_SURFACE(((1.,1.),(1.,1.),(1.,1.),(1.,1.),(1.,1.),(1.,
1.),(1.,1.),(1.,1.),(1.,1.),(1.,1.),(1.,1.),(1.,1.),(1.,1.),(1.,1.),(1.,
1.),(1.,1.),(1.,1.),(1.,1.),(1.,1.),(1.,1.),(1.,1.),(1.,1.),(1.,1.),(1.,
1.),(1.,1.),(1.,1.),(1.,1.),(1.,1.),(1.,1.),(1.,1.),(1.,1.),(1.,1.),(1.,
1.),(1.,1.),(1.,1.),(1.,1.),(1.,1.),(1.,1.),(1.,1.),(1.,1.),(1.,1.),(1.,
1.),(1.,1.),(1.,1.),(1.,1.),(1.,1.),(1.,1.),(1.,1.),(1.,1.),(1.,1.),(1.,
1.),(1.,1.),(1.,1.),(1.,1.),(1.,1.),(1.,1.),(1.,1.),(1.,1.),(1.,1.),(1.,
1.),(1.,1.),(1.,1.),(1.,1.),(1.,1.),(1.,1.),(1.,1.),(1.,1.),(1.,1.),(1.,
1.),(1.,1.)))
REPRESENTATION_ITEM('')
SURFACE()
);
#43=(
BOUNDED_SURFACE()
B_SPLINE_SURFACE(5,1,((#30688,#30689),(#30690,#30691),(#30692,#30693),(#30694,
#30695),(#30696,#30697),(#30698,#30699),(#30700,#30701),(#30702,#30703),
(#30704,#30705),(#30706,#30707),(#30708,#30709),(#30710,#30711),(#30712,
#30713),(#30714,#30715),(#30716,#30717),(#30718,#30719),(#30720,#30721),
(#30722,#30723),(#30724,#30725),(#30726,#30727),(#30728,#30729),(#30730,
#30731),(#30732,#30733),(#30734,#30735),(#30736,#30737),(#30738,#30739),
(#30740,#30741),(#30742,#30743),(#30744,#30745),(#30746,#30747),(#30748,
#30749),(#30750,#30751),(#30752,#30753),(#30754,#30755),(#30756,#30757),
(#30758,#30759),(#30760,#30761),(#30762,#30763),(#30764,#30765),(#30766,
#30767),(#30768,#30769),(#30770,#30771),(#30772,#30773),(#30774,#30775),
(#30776,#30777),(#30778,#30779),(#30780,#30781),(#30782,#30783),(#30784,
#30785),(#30786,#30787),(#30788,#30789),(#30790,#30791),(#30792,#30793),
(#30794,#30795),(#30796,#30797),(#30798,#30799),(#30800,#30801),(#30802,
#30803),(#30804,#30805),(#30806,#30807),(#30808,#30809),(#30810,#30811),
(#30812,#30813),(#30814,#30815),(#30816,#30817),(#30818,#30819),(#30820,
#30821),(#30822,#30823),(#30824,#30825),(#30826,#30827)),.UNSPECIFIED.,
 .F.,.F.,.F.)
B_SPLINE_SURFACE_WITH_KNOTS((6,1,1,1,1,1,1,1,1,1,1,1,1,1,1,1,1,1,1,1,1,
1,1,1,1,1,1,1,1,1,1,1,1,1,1,1,1,1,1,1,1,1,1,1,1,1,1,1,1,1,1,1,1,1,1,1,1,
1,1,1,1,1,1,1,1,6),(2,2),(-1.,-0.984615384615383,-0.969230769230768,-0.953846153846152,
-0.938461538461537,-0.923076923076922,-0.907692307692306,-0.892307692307691,
-0.876923076923076,-0.86153846153846,-0.846153846153845,-0.83076923076923,
-0.815384615384614,-0.799999999999999,-0.784615384615384,-0.769230769230768,
-0.753846153846153,-0.738461538461538,-0.723076923076922,-0.707692307692307,
-0.692307692307692,-0.676923076923076,-0.661538461538461,-0.646153846153846,
-0.63076923076923,-0.615384615384615,-0.6,-0.584615384615384,-0.569230769230769,
-0.553846153846154,-0.538461538461538,-0.523076923076923,-0.507692307692308,
-0.492307692307692,-0.476923076923077,-0.461538461538462,-0.446153846153846,
-0.430769230769231,-0.415384615384615,-0.4,-0.384615384615385,-0.369230769230769,
-0.353846153846154,-0.338461538461538,-0.323076923076923,-0.307692307692308,
-0.292307692307692,-0.276923076923077,-0.261538461538462,-0.246153846153846,
-0.230769230769231,-0.215384615384615,-0.2,-0.184615384615385,-0.169230769230769,
-0.153846153846154,-0.138461538461538,-0.123076923076923,-0.107692307692308,
-0.0923076923076923,-0.0769230769230769,-0.0615384615384615,-0.0461538461538462,
-0.0307692307692308,-0.0153846153846154,0.),(-1.,1.),.UNSPECIFIED.)
GEOMETRIC_REPRESENTATION_ITEM()
RATIONAL_B_SPLINE_SURFACE(((1.,1.),(1.,1.),(1.,1.),(1.,1.),(1.,1.),(1.,
1.),(1.,1.),(1.,1.),(1.,1.),(1.,1.),(1.,1.),(1.,1.),(1.,1.),(1.,1.),(1.,
1.),(1.,1.),(1.,1.),(1.,1.),(1.,1.),(1.,1.),(1.,1.),(1.,1.),(1.,1.),(1.,
1.),(1.,1.),(1.,1.),(1.,1.),(1.,1.),(1.,1.),(1.,1.),(1.,1.),(1.,1.),(1.,
1.),(1.,1.),(1.,1.),(1.,1.),(1.,1.),(1.,1.),(1.,1.),(1.,1.),(1.,1.),(1.,
1.),(1.,1.),(1.,1.),(1.,1.),(1.,1.),(1.,1.),(1.,1.),(1.,1.),(1.,1.),(1.,
1.),(1.,1.),(1.,1.),(1.,1.),(1.,1.),(1.,1.),(1.,1.),(1.,1.),(1.,1.),(1.,
1.),(1.,1.),(1.,1.),(1.,1.),(1.,1.),(1.,1.),(1.,1.),(1.,1.),(1.,1.),(1.,
1.),(1.,1.)))
REPRESENTATION_ITEM('')
SURFACE()
);
#44=(
BOUNDED_SURFACE()
B_SPLINE_SURFACE(5,1,((#30904,#30905),(#30906,#30907),(#30908,#30909),(#30910,
#30911),(#30912,#30913),(#30914,#30915),(#30916,#30917),(#30918,#30919),
(#30920,#30921),(#30922,#30923),(#30924,#30925),(#30926,#30927),(#30928,
#30929),(#30930,#30931),(#30932,#30933),(#30934,#30935),(#30936,#30937),
(#30938,#30939),(#30940,#30941),(#30942,#30943),(#30944,#30945),(#30946,
#30947),(#30948,#30949),(#30950,#30951),(#30952,#30953),(#30954,#30955),
(#30956,#30957),(#30958,#30959),(#30960,#30961),(#30962,#30963),(#30964,
#30965),(#30966,#30967),(#30968,#30969),(#30970,#30971),(#30972,#30973),
(#30974,#30975),(#30976,#30977),(#30978,#30979),(#30980,#30981),(#30982,
#30983),(#30984,#30985),(#30986,#30987),(#30988,#30989),(#30990,#30991),
(#30992,#30993),(#30994,#30995),(#30996,#30997),(#30998,#30999),(#31000,
#31001),(#31002,#31003),(#31004,#31005),(#31006,#31007),(#31008,#31009),
(#31010,#31011),(#31012,#31013),(#31014,#31015),(#31016,#31017),(#31018,
#31019),(#31020,#31021),(#31022,#31023),(#31024,#31025),(#31026,#31027),
(#31028,#31029),(#31030,#31031),(#31032,#31033),(#31034,#31035),(#31036,
#31037),(#31038,#31039),(#31040,#31041),(#31042,#31043)),.UNSPECIFIED.,
 .F.,.F.,.F.)
B_SPLINE_SURFACE_WITH_KNOTS((6,1,1,1,1,1,1,1,1,1,1,1,1,1,1,1,1,1,1,1,1,
1,1,1,1,1,1,1,1,1,1,1,1,1,1,1,1,1,1,1,1,1,1,1,1,1,1,1,1,1,1,1,1,1,1,1,1,
1,1,1,1,1,1,1,1,6),(2,2),(-1.,-0.984615384615383,-0.969230769230768,-0.953846153846152,
-0.938461538461537,-0.923076923076922,-0.907692307692306,-0.892307692307691,
-0.876923076923076,-0.86153846153846,-0.846153846153845,-0.83076923076923,
-0.815384615384614,-0.799999999999999,-0.784615384615384,-0.769230769230768,
-0.753846153846153,-0.738461538461538,-0.723076923076922,-0.707692307692307,
-0.692307692307692,-0.676923076923076,-0.661538461538461,-0.646153846153846,
-0.63076923076923,-0.615384615384615,-0.6,-0.584615384615384,-0.569230769230769,
-0.553846153846154,-0.538461538461538,-0.523076923076923,-0.507692307692308,
-0.492307692307692,-0.476923076923077,-0.461538461538462,-0.446153846153846,
-0.430769230769231,-0.415384615384615,-0.4,-0.384615384615385,-0.369230769230769,
-0.353846153846154,-0.338461538461538,-0.323076923076923,-0.307692307692308,
-0.292307692307692,-0.276923076923077,-0.261538461538462,-0.246153846153846,
-0.230769230769231,-0.215384615384615,-0.2,-0.184615384615385,-0.169230769230769,
-0.153846153846154,-0.138461538461538,-0.123076923076923,-0.107692307692308,
-0.0923076923076923,-0.0769230769230769,-0.0615384615384615,-0.0461538461538462,
-0.0307692307692308,-0.0153846153846154,0.),(-1.,1.),.UNSPECIFIED.)
GEOMETRIC_REPRESENTATION_ITEM()
RATIONAL_B_SPLINE_SURFACE(((1.,1.),(1.,1.),(1.,1.),(1.,1.),(1.,1.),(1.,
1.),(1.,1.),(1.,1.),(1.,1.),(1.,1.),(1.,1.),(1.,1.),(1.,1.),(1.,1.),(1.,
1.),(1.,1.),(1.,1.),(1.,1.),(1.,1.),(1.,1.),(1.,1.),(1.,1.),(1.,1.),(1.,
1.),(1.,1.),(1.,1.),(1.,1.),(1.,1.),(1.,1.),(1.,1.),(1.,1.),(1.,1.),(1.,
1.),(1.,1.),(1.,1.),(1.,1.),(1.,1.),(1.,1.),(1.,1.),(1.,1.),(1.,1.),(1.,
1.),(1.,1.),(1.,1.),(1.,1.),(1.,1.),(1.,1.),(1.,1.),(1.,1.),(1.,1.),(1.,
1.),(1.,1.),(1.,1.),(1.,1.),(1.,1.),(1.,1.),(1.,1.),(1.,1.),(1.,1.),(1.,
1.),(1.,1.),(1.,1.),(1.,1.),(1.,1.),(1.,1.),(1.,1.),(1.,1.),(1.,1.),(1.,
1.),(1.,1.)))
REPRESENTATION_ITEM('')
SURFACE()
);
#45=(
BOUNDED_SURFACE()
B_SPLINE_SURFACE(5,1,((#31120,#31121),(#31122,#31123),(#31124,#31125),(#31126,
#31127),(#31128,#31129),(#31130,#31131),(#31132,#31133),(#31134,#31135),
(#31136,#31137),(#31138,#31139),(#31140,#31141),(#31142,#31143),(#31144,
#31145),(#31146,#31147),(#31148,#31149),(#31150,#31151),(#31152,#31153),
(#31154,#31155),(#31156,#31157),(#31158,#31159),(#31160,#31161),(#31162,
#31163),(#31164,#31165),(#31166,#31167),(#31168,#31169),(#31170,#31171),
(#31172,#31173),(#31174,#31175),(#31176,#31177),(#31178,#31179),(#31180,
#31181),(#31182,#31183),(#31184,#31185),(#31186,#31187),(#31188,#31189),
(#31190,#31191),(#31192,#31193),(#31194,#31195),(#31196,#31197),(#31198,
#31199),(#31200,#31201),(#31202,#31203),(#31204,#31205),(#31206,#31207),
(#31208,#31209),(#31210,#31211),(#31212,#31213),(#31214,#31215),(#31216,
#31217),(#31218,#31219),(#31220,#31221),(#31222,#31223),(#31224,#31225),
(#31226,#31227),(#31228,#31229),(#31230,#31231),(#31232,#31233),(#31234,
#31235),(#31236,#31237),(#31238,#31239),(#31240,#31241),(#31242,#31243),
(#31244,#31245),(#31246,#31247),(#31248,#31249),(#31250,#31251),(#31252,
#31253),(#31254,#31255),(#31256,#31257),(#31258,#31259)),.UNSPECIFIED.,
 .F.,.F.,.F.)
B_SPLINE_SURFACE_WITH_KNOTS((6,1,1,1,1,1,1,1,1,1,1,1,1,1,1,1,1,1,1,1,1,
1,1,1,1,1,1,1,1,1,1,1,1,1,1,1,1,1,1,1,1,1,1,1,1,1,1,1,1,1,1,1,1,1,1,1,1,
1,1,1,1,1,1,1,1,6),(2,2),(-1.,-0.984615384615383,-0.969230769230768,-0.953846153846152,
-0.938461538461537,-0.923076923076922,-0.907692307692306,-0.892307692307691,
-0.876923076923076,-0.86153846153846,-0.846153846153845,-0.83076923076923,
-0.815384615384614,-0.799999999999999,-0.784615384615384,-0.769230769230768,
-0.753846153846153,-0.738461538461538,-0.723076923076922,-0.707692307692307,
-0.692307692307692,-0.676923076923076,-0.661538461538461,-0.646153846153846,
-0.63076923076923,-0.615384615384615,-0.6,-0.584615384615384,-0.569230769230769,
-0.553846153846154,-0.538461538461538,-0.523076923076923,-0.507692307692308,
-0.492307692307692,-0.476923076923077,-0.461538461538462,-0.446153846153846,
-0.430769230769231,-0.415384615384615,-0.4,-0.384615384615385,-0.369230769230769,
-0.353846153846154,-0.338461538461538,-0.323076923076923,-0.307692307692308,
-0.292307692307692,-0.276923076923077,-0.261538461538462,-0.246153846153846,
-0.230769230769231,-0.215384615384615,-0.2,-0.184615384615385,-0.169230769230769,
-0.153846153846154,-0.138461538461538,-0.123076923076923,-0.107692307692308,
-0.0923076923076923,-0.0769230769230769,-0.0615384615384615,-0.0461538461538462,
-0.0307692307692308,-0.0153846153846154,0.),(-1.,1.),.UNSPECIFIED.)
GEOMETRIC_REPRESENTATION_ITEM()
RATIONAL_B_SPLINE_SURFACE(((1.,1.),(1.,1.),(1.,1.),(1.,1.),(1.,1.),(1.,
1.),(1.,1.),(1.,1.),(1.,1.),(1.,1.),(1.,1.),(1.,1.),(1.,1.),(1.,1.),(1.,
1.),(1.,1.),(1.,1.),(1.,1.),(1.,1.),(1.,1.),(1.,1.),(1.,1.),(1.,1.),(1.,
1.),(1.,1.),(1.,1.),(1.,1.),(1.,1.),(1.,1.),(1.,1.),(1.,1.),(1.,1.),(1.,
1.),(1.,1.),(1.,1.),(1.,1.),(1.,1.),(1.,1.),(1.,1.),(1.,1.),(1.,1.),(1.,
1.),(1.,1.),(1.,1.),(1.,1.),(1.,1.),(1.,1.),(1.,1.),(1.,1.),(1.,1.),(1.,
1.),(1.,1.),(1.,1.),(1.,1.),(1.,1.),(1.,1.),(1.,1.),(1.,1.),(1.,1.),(1.,
1.),(1.,1.),(1.,1.),(1.,1.),(1.,1.),(1.,1.),(1.,1.),(1.,1.),(1.,1.),(1.,
1.),(1.,1.)))
REPRESENTATION_ITEM('')
SURFACE()
);
#46=(
BOUNDED_SURFACE()
B_SPLINE_SURFACE(5,1,((#31336,#31337),(#31338,#31339),(#31340,#31341),(#31342,
#31343),(#31344,#31345),(#31346,#31347),(#31348,#31349),(#31350,#31351),
(#31352,#31353),(#31354,#31355),(#31356,#31357),(#31358,#31359),(#31360,
#31361),(#31362,#31363),(#31364,#31365),(#31366,#31367),(#31368,#31369),
(#31370,#31371),(#31372,#31373),(#31374,#31375),(#31376,#31377),(#31378,
#31379),(#31380,#31381),(#31382,#31383),(#31384,#31385),(#31386,#31387),
(#31388,#31389),(#31390,#31391),(#31392,#31393),(#31394,#31395),(#31396,
#31397),(#31398,#31399),(#31400,#31401),(#31402,#31403),(#31404,#31405),
(#31406,#31407),(#31408,#31409),(#31410,#31411),(#31412,#31413),(#31414,
#31415),(#31416,#31417),(#31418,#31419),(#31420,#31421),(#31422,#31423),
(#31424,#31425),(#31426,#31427),(#31428,#31429),(#31430,#31431),(#31432,
#31433),(#31434,#31435),(#31436,#31437),(#31438,#31439),(#31440,#31441),
(#31442,#31443),(#31444,#31445),(#31446,#31447),(#31448,#31449),(#31450,
#31451),(#31452,#31453),(#31454,#31455),(#31456,#31457),(#31458,#31459),
(#31460,#31461),(#31462,#31463),(#31464,#31465),(#31466,#31467),(#31468,
#31469),(#31470,#31471),(#31472,#31473),(#31474,#31475)),.UNSPECIFIED.,
 .F.,.F.,.F.)
B_SPLINE_SURFACE_WITH_KNOTS((6,1,1,1,1,1,1,1,1,1,1,1,1,1,1,1,1,1,1,1,1,
1,1,1,1,1,1,1,1,1,1,1,1,1,1,1,1,1,1,1,1,1,1,1,1,1,1,1,1,1,1,1,1,1,1,1,1,
1,1,1,1,1,1,1,1,6),(2,2),(-1.,-0.984615384615383,-0.969230769230768,-0.953846153846152,
-0.938461538461537,-0.923076923076922,-0.907692307692306,-0.892307692307691,
-0.876923076923076,-0.86153846153846,-0.846153846153845,-0.83076923076923,
-0.815384615384614,-0.799999999999999,-0.784615384615384,-0.769230769230768,
-0.753846153846153,-0.738461538461538,-0.723076923076922,-0.707692307692307,
-0.692307692307692,-0.676923076923076,-0.661538461538461,-0.646153846153846,
-0.63076923076923,-0.615384615384615,-0.6,-0.584615384615384,-0.569230769230769,
-0.553846153846154,-0.538461538461538,-0.523076923076923,-0.507692307692308,
-0.492307692307692,-0.476923076923077,-0.461538461538462,-0.446153846153846,
-0.430769230769231,-0.415384615384615,-0.4,-0.384615384615385,-0.369230769230769,
-0.353846153846154,-0.338461538461538,-0.323076923076923,-0.307692307692308,
-0.292307692307692,-0.276923076923077,-0.261538461538462,-0.246153846153846,
-0.230769230769231,-0.215384615384615,-0.2,-0.184615384615385,-0.169230769230769,
-0.153846153846154,-0.138461538461538,-0.123076923076923,-0.107692307692308,
-0.0923076923076923,-0.0769230769230769,-0.0615384615384615,-0.0461538461538462,
-0.0307692307692308,-0.0153846153846154,0.),(-1.,1.),.UNSPECIFIED.)
GEOMETRIC_REPRESENTATION_ITEM()
RATIONAL_B_SPLINE_SURFACE(((1.,1.),(1.,1.),(1.,1.),(1.,1.),(1.,1.),(1.,
1.),(1.,1.),(1.,1.),(1.,1.),(1.,1.),(1.,1.),(1.,1.),(1.,1.),(1.,1.),(1.,
1.),(1.,1.),(1.,1.),(1.,1.),(1.,1.),(1.,1.),(1.,1.),(1.,1.),(1.,1.),(1.,
1.),(1.,1.),(1.,1.),(1.,1.),(1.,1.),(1.,1.),(1.,1.),(1.,1.),(1.,1.),(1.,
1.),(1.,1.),(1.,1.),(1.,1.),(1.,1.),(1.,1.),(1.,1.),(1.,1.),(1.,1.),(1.,
1.),(1.,1.),(1.,1.),(1.,1.),(1.,1.),(1.,1.),(1.,1.),(1.,1.),(1.,1.),(1.,
1.),(1.,1.),(1.,1.),(1.,1.),(1.,1.),(1.,1.),(1.,1.),(1.,1.),(1.,1.),(1.,
1.),(1.,1.),(1.,1.),(1.,1.),(1.,1.),(1.,1.),(1.,1.),(1.,1.),(1.,1.),(1.,
1.),(1.,1.)))
REPRESENTATION_ITEM('')
SURFACE()
);
#47=(
BOUNDED_SURFACE()
B_SPLINE_SURFACE(5,1,((#31552,#31553),(#31554,#31555),(#31556,#31557),(#31558,
#31559),(#31560,#31561),(#31562,#31563),(#31564,#31565),(#31566,#31567),
(#31568,#31569),(#31570,#31571),(#31572,#31573),(#31574,#31575),(#31576,
#31577),(#31578,#31579),(#31580,#31581),(#31582,#31583),(#31584,#31585),
(#31586,#31587),(#31588,#31589),(#31590,#31591),(#31592,#31593),(#31594,
#31595),(#31596,#31597),(#31598,#31599),(#31600,#31601),(#31602,#31603),
(#31604,#31605),(#31606,#31607),(#31608,#31609),(#31610,#31611),(#31612,
#31613),(#31614,#31615),(#31616,#31617),(#31618,#31619),(#31620,#31621),
(#31622,#31623),(#31624,#31625),(#31626,#31627),(#31628,#31629),(#31630,
#31631),(#31632,#31633),(#31634,#31635),(#31636,#31637),(#31638,#31639),
(#31640,#31641),(#31642,#31643),(#31644,#31645),(#31646,#31647),(#31648,
#31649),(#31650,#31651),(#31652,#31653),(#31654,#31655),(#31656,#31657),
(#31658,#31659),(#31660,#31661),(#31662,#31663),(#31664,#31665),(#31666,
#31667),(#31668,#31669),(#31670,#31671),(#31672,#31673),(#31674,#31675),
(#31676,#31677),(#31678,#31679),(#31680,#31681),(#31682,#31683),(#31684,
#31685),(#31686,#31687),(#31688,#31689),(#31690,#31691)),.UNSPECIFIED.,
 .F.,.F.,.F.)
B_SPLINE_SURFACE_WITH_KNOTS((6,1,1,1,1,1,1,1,1,1,1,1,1,1,1,1,1,1,1,1,1,
1,1,1,1,1,1,1,1,1,1,1,1,1,1,1,1,1,1,1,1,1,1,1,1,1,1,1,1,1,1,1,1,1,1,1,1,
1,1,1,1,1,1,1,1,6),(2,2),(-1.,-0.984615384615383,-0.969230769230768,-0.953846153846152,
-0.938461538461537,-0.923076923076922,-0.907692307692306,-0.892307692307691,
-0.876923076923076,-0.86153846153846,-0.846153846153845,-0.83076923076923,
-0.815384615384614,-0.799999999999999,-0.784615384615384,-0.769230769230768,
-0.753846153846153,-0.738461538461538,-0.723076923076922,-0.707692307692307,
-0.692307692307692,-0.676923076923076,-0.661538461538461,-0.646153846153846,
-0.63076923076923,-0.615384615384615,-0.6,-0.584615384615384,-0.569230769230769,
-0.553846153846154,-0.538461538461538,-0.523076923076923,-0.507692307692308,
-0.492307692307692,-0.476923076923077,-0.461538461538462,-0.446153846153846,
-0.430769230769231,-0.415384615384615,-0.4,-0.384615384615385,-0.369230769230769,
-0.353846153846154,-0.338461538461538,-0.323076923076923,-0.307692307692308,
-0.292307692307692,-0.276923076923077,-0.261538461538462,-0.246153846153846,
-0.230769230769231,-0.215384615384615,-0.2,-0.184615384615385,-0.169230769230769,
-0.153846153846154,-0.138461538461538,-0.123076923076923,-0.107692307692308,
-0.0923076923076923,-0.0769230769230769,-0.0615384615384615,-0.0461538461538462,
-0.0307692307692308,-0.0153846153846154,0.),(-1.,1.),.UNSPECIFIED.)
GEOMETRIC_REPRESENTATION_ITEM()
RATIONAL_B_SPLINE_SURFACE(((1.,1.),(1.,1.),(1.,1.),(1.,1.),(1.,1.),(1.,
1.),(1.,1.),(1.,1.),(1.,1.),(1.,1.),(1.,1.),(1.,1.),(1.,1.),(1.,1.),(1.,
1.),(1.,1.),(1.,1.),(1.,1.),(1.,1.),(1.,1.),(1.,1.),(1.,1.),(1.,1.),(1.,
1.),(1.,1.),(1.,1.),(1.,1.),(1.,1.),(1.,1.),(1.,1.),(1.,1.),(1.,1.),(1.,
1.),(1.,1.),(1.,1.),(1.,1.),(1.,1.),(1.,1.),(1.,1.),(1.,1.),(1.,1.),(1.,
1.),(1.,1.),(1.,1.),(1.,1.),(1.,1.),(1.,1.),(1.,1.),(1.,1.),(1.,1.),(1.,
1.),(1.,1.),(1.,1.),(1.,1.),(1.,1.),(1.,1.),(1.,1.),(1.,1.),(1.,1.),(1.,
1.),(1.,1.),(1.,1.),(1.,1.),(1.,1.),(1.,1.),(1.,1.),(1.,1.),(1.,1.),(1.,
1.),(1.,1.)))
REPRESENTATION_ITEM('')
SURFACE()
);
#48=(
BOUNDED_SURFACE()
B_SPLINE_SURFACE(5,1,((#31768,#31769),(#31770,#31771),(#31772,#31773),(#31774,
#31775),(#31776,#31777),(#31778,#31779),(#31780,#31781),(#31782,#31783),
(#31784,#31785),(#31786,#31787),(#31788,#31789),(#31790,#31791),(#31792,
#31793),(#31794,#31795),(#31796,#31797),(#31798,#31799),(#31800,#31801),
(#31802,#31803),(#31804,#31805),(#31806,#31807),(#31808,#31809),(#31810,
#31811),(#31812,#31813),(#31814,#31815),(#31816,#31817),(#31818,#31819),
(#31820,#31821),(#31822,#31823),(#31824,#31825),(#31826,#31827),(#31828,
#31829),(#31830,#31831),(#31832,#31833),(#31834,#31835),(#31836,#31837),
(#31838,#31839),(#31840,#31841),(#31842,#31843),(#31844,#31845),(#31846,
#31847),(#31848,#31849),(#31850,#31851),(#31852,#31853),(#31854,#31855),
(#31856,#31857),(#31858,#31859),(#31860,#31861),(#31862,#31863),(#31864,
#31865),(#31866,#31867),(#31868,#31869),(#31870,#31871),(#31872,#31873),
(#31874,#31875),(#31876,#31877),(#31878,#31879),(#31880,#31881),(#31882,
#31883),(#31884,#31885),(#31886,#31887),(#31888,#31889),(#31890,#31891),
(#31892,#31893),(#31894,#31895),(#31896,#31897),(#31898,#31899),(#31900,
#31901),(#31902,#31903),(#31904,#31905),(#31906,#31907)),.UNSPECIFIED.,
 .F.,.F.,.F.)
B_SPLINE_SURFACE_WITH_KNOTS((6,1,1,1,1,1,1,1,1,1,1,1,1,1,1,1,1,1,1,1,1,
1,1,1,1,1,1,1,1,1,1,1,1,1,1,1,1,1,1,1,1,1,1,1,1,1,1,1,1,1,1,1,1,1,1,1,1,
1,1,1,1,1,1,1,1,6),(2,2),(-1.,-0.984615384615383,-0.969230769230768,-0.953846153846152,
-0.938461538461537,-0.923076923076922,-0.907692307692306,-0.892307692307691,
-0.876923076923076,-0.86153846153846,-0.846153846153845,-0.83076923076923,
-0.815384615384614,-0.799999999999999,-0.784615384615384,-0.769230769230768,
-0.753846153846153,-0.738461538461538,-0.723076923076922,-0.707692307692307,
-0.692307692307692,-0.676923076923076,-0.661538461538461,-0.646153846153846,
-0.63076923076923,-0.615384615384615,-0.6,-0.584615384615384,-0.569230769230769,
-0.553846153846154,-0.538461538461538,-0.523076923076923,-0.507692307692308,
-0.492307692307692,-0.476923076923077,-0.461538461538462,-0.446153846153846,
-0.430769230769231,-0.415384615384615,-0.4,-0.384615384615385,-0.369230769230769,
-0.353846153846154,-0.338461538461538,-0.323076923076923,-0.307692307692308,
-0.292307692307692,-0.276923076923077,-0.261538461538462,-0.246153846153846,
-0.230769230769231,-0.215384615384615,-0.2,-0.184615384615385,-0.169230769230769,
-0.153846153846154,-0.138461538461538,-0.123076923076923,-0.107692307692308,
-0.0923076923076923,-0.0769230769230769,-0.0615384615384615,-0.0461538461538462,
-0.0307692307692308,-0.0153846153846154,0.),(-1.,1.),.UNSPECIFIED.)
GEOMETRIC_REPRESENTATION_ITEM()
RATIONAL_B_SPLINE_SURFACE(((1.,1.),(1.,1.),(1.,1.),(1.,1.),(1.,1.),(1.,
1.),(1.,1.),(1.,1.),(1.,1.),(1.,1.),(1.,1.),(1.,1.),(1.,1.),(1.,1.),(1.,
1.),(1.,1.),(1.,1.),(1.,1.),(1.,1.),(1.,1.),(1.,1.),(1.,1.),(1.,1.),(1.,
1.),(1.,1.),(1.,1.),(1.,1.),(1.,1.),(1.,1.),(1.,1.),(1.,1.),(1.,1.),(1.,
1.),(1.,1.),(1.,1.),(1.,1.),(1.,1.),(1.,1.),(1.,1.),(1.,1.),(1.,1.),(1.,
1.),(1.,1.),(1.,1.),(1.,1.),(1.,1.),(1.,1.),(1.,1.),(1.,1.),(1.,1.),(1.,
1.),(1.,1.),(1.,1.),(1.,1.),(1.,1.),(1.,1.),(1.,1.),(1.,1.),(1.,1.),(1.,
1.),(1.,1.),(1.,1.),(1.,1.),(1.,1.),(1.,1.),(1.,1.),(1.,1.),(1.,1.),(1.,
1.),(1.,1.)))
REPRESENTATION_ITEM('')
SURFACE()
);
#49=(
BOUNDED_SURFACE()
B_SPLINE_SURFACE(5,1,((#31984,#31985),(#31986,#31987),(#31988,#31989),(#31990,
#31991),(#31992,#31993),(#31994,#31995),(#31996,#31997),(#31998,#31999),
(#32000,#32001),(#32002,#32003),(#32004,#32005),(#32006,#32007),(#32008,
#32009),(#32010,#32011),(#32012,#32013),(#32014,#32015),(#32016,#32017),
(#32018,#32019),(#32020,#32021),(#32022,#32023),(#32024,#32025),(#32026,
#32027),(#32028,#32029),(#32030,#32031),(#32032,#32033),(#32034,#32035),
(#32036,#32037),(#32038,#32039),(#32040,#32041),(#32042,#32043),(#32044,
#32045),(#32046,#32047),(#32048,#32049),(#32050,#32051),(#32052,#32053),
(#32054,#32055),(#32056,#32057),(#32058,#32059),(#32060,#32061),(#32062,
#32063),(#32064,#32065),(#32066,#32067),(#32068,#32069),(#32070,#32071),
(#32072,#32073),(#32074,#32075),(#32076,#32077),(#32078,#32079),(#32080,
#32081),(#32082,#32083),(#32084,#32085),(#32086,#32087),(#32088,#32089),
(#32090,#32091),(#32092,#32093),(#32094,#32095),(#32096,#32097),(#32098,
#32099),(#32100,#32101),(#32102,#32103),(#32104,#32105),(#32106,#32107),
(#32108,#32109),(#32110,#32111),(#32112,#32113),(#32114,#32115),(#32116,
#32117),(#32118,#32119),(#32120,#32121),(#32122,#32123)),.UNSPECIFIED.,
 .F.,.F.,.F.)
B_SPLINE_SURFACE_WITH_KNOTS((6,1,1,1,1,1,1,1,1,1,1,1,1,1,1,1,1,1,1,1,1,
1,1,1,1,1,1,1,1,1,1,1,1,1,1,1,1,1,1,1,1,1,1,1,1,1,1,1,1,1,1,1,1,1,1,1,1,
1,1,1,1,1,1,1,1,6),(2,2),(-1.,-0.984615384615383,-0.969230769230768,-0.953846153846152,
-0.938461538461537,-0.923076923076922,-0.907692307692306,-0.892307692307691,
-0.876923076923076,-0.86153846153846,-0.846153846153845,-0.83076923076923,
-0.815384615384614,-0.799999999999999,-0.784615384615384,-0.769230769230768,
-0.753846153846153,-0.738461538461538,-0.723076923076922,-0.707692307692307,
-0.692307692307692,-0.676923076923076,-0.661538461538461,-0.646153846153846,
-0.63076923076923,-0.615384615384615,-0.6,-0.584615384615384,-0.569230769230769,
-0.553846153846154,-0.538461538461538,-0.523076923076923,-0.507692307692308,
-0.492307692307692,-0.476923076923077,-0.461538461538462,-0.446153846153846,
-0.430769230769231,-0.415384615384615,-0.4,-0.384615384615385,-0.369230769230769,
-0.353846153846154,-0.338461538461538,-0.323076923076923,-0.307692307692308,
-0.292307692307692,-0.276923076923077,-0.261538461538462,-0.246153846153846,
-0.230769230769231,-0.215384615384615,-0.2,-0.184615384615385,-0.169230769230769,
-0.153846153846154,-0.138461538461538,-0.123076923076923,-0.107692307692308,
-0.0923076923076923,-0.0769230769230769,-0.0615384615384615,-0.0461538461538462,
-0.0307692307692308,-0.0153846153846154,0.),(-1.,1.),.UNSPECIFIED.)
GEOMETRIC_REPRESENTATION_ITEM()
RATIONAL_B_SPLINE_SURFACE(((1.,1.),(1.,1.),(1.,1.),(1.,1.),(1.,1.),(1.,
1.),(1.,1.),(1.,1.),(1.,1.),(1.,1.),(1.,1.),(1.,1.),(1.,1.),(1.,1.),(1.,
1.),(1.,1.),(1.,1.),(1.,1.),(1.,1.),(1.,1.),(1.,1.),(1.,1.),(1.,1.),(1.,
1.),(1.,1.),(1.,1.),(1.,1.),(1.,1.),(1.,1.),(1.,1.),(1.,1.),(1.,1.),(1.,
1.),(1.,1.),(1.,1.),(1.,1.),(1.,1.),(1.,1.),(1.,1.),(1.,1.),(1.,1.),(1.,
1.),(1.,1.),(1.,1.),(1.,1.),(1.,1.),(1.,1.),(1.,1.),(1.,1.),(1.,1.),(1.,
1.),(1.,1.),(1.,1.),(1.,1.),(1.,1.),(1.,1.),(1.,1.),(1.,1.),(1.,1.),(1.,
1.),(1.,1.),(1.,1.),(1.,1.),(1.,1.),(1.,1.),(1.,1.),(1.,1.),(1.,1.),(1.,
1.),(1.,1.)))
REPRESENTATION_ITEM('')
SURFACE()
);
#50=(
BOUNDED_SURFACE()
B_SPLINE_SURFACE(5,1,((#32200,#32201),(#32202,#32203),(#32204,#32205),(#32206,
#32207),(#32208,#32209),(#32210,#32211),(#32212,#32213),(#32214,#32215),
(#32216,#32217),(#32218,#32219),(#32220,#32221),(#32222,#32223),(#32224,
#32225),(#32226,#32227),(#32228,#32229),(#32230,#32231),(#32232,#32233),
(#32234,#32235),(#32236,#32237),(#32238,#32239),(#32240,#32241),(#32242,
#32243),(#32244,#32245),(#32246,#32247),(#32248,#32249),(#32250,#32251),
(#32252,#32253),(#32254,#32255),(#32256,#32257),(#32258,#32259),(#32260,
#32261),(#32262,#32263),(#32264,#32265),(#32266,#32267),(#32268,#32269),
(#32270,#32271),(#32272,#32273),(#32274,#32275),(#32276,#32277),(#32278,
#32279),(#32280,#32281),(#32282,#32283),(#32284,#32285),(#32286,#32287),
(#32288,#32289),(#32290,#32291),(#32292,#32293),(#32294,#32295),(#32296,
#32297),(#32298,#32299),(#32300,#32301),(#32302,#32303),(#32304,#32305),
(#32306,#32307),(#32308,#32309),(#32310,#32311),(#32312,#32313),(#32314,
#32315),(#32316,#32317),(#32318,#32319),(#32320,#32321),(#32322,#32323),
(#32324,#32325),(#32326,#32327),(#32328,#32329),(#32330,#32331),(#32332,
#32333),(#32334,#32335),(#32336,#32337),(#32338,#32339)),.UNSPECIFIED.,
 .F.,.F.,.F.)
B_SPLINE_SURFACE_WITH_KNOTS((6,1,1,1,1,1,1,1,1,1,1,1,1,1,1,1,1,1,1,1,1,
1,1,1,1,1,1,1,1,1,1,1,1,1,1,1,1,1,1,1,1,1,1,1,1,1,1,1,1,1,1,1,1,1,1,1,1,
1,1,1,1,1,1,1,1,6),(2,2),(-1.,-0.984615384615383,-0.969230769230768,-0.953846153846152,
-0.938461538461537,-0.923076923076922,-0.907692307692306,-0.892307692307691,
-0.876923076923076,-0.86153846153846,-0.846153846153845,-0.83076923076923,
-0.815384615384614,-0.799999999999999,-0.784615384615384,-0.769230769230768,
-0.753846153846153,-0.738461538461538,-0.723076923076922,-0.707692307692307,
-0.692307692307692,-0.676923076923076,-0.661538461538461,-0.646153846153846,
-0.63076923076923,-0.615384615384615,-0.6,-0.584615384615384,-0.569230769230769,
-0.553846153846154,-0.538461538461538,-0.523076923076923,-0.507692307692308,
-0.492307692307692,-0.476923076923077,-0.461538461538462,-0.446153846153846,
-0.430769230769231,-0.415384615384615,-0.4,-0.384615384615385,-0.369230769230769,
-0.353846153846154,-0.338461538461538,-0.323076923076923,-0.307692307692308,
-0.292307692307692,-0.276923076923077,-0.261538461538462,-0.246153846153846,
-0.230769230769231,-0.215384615384615,-0.2,-0.184615384615385,-0.169230769230769,
-0.153846153846154,-0.138461538461538,-0.123076923076923,-0.107692307692308,
-0.0923076923076923,-0.0769230769230769,-0.0615384615384615,-0.0461538461538462,
-0.0307692307692308,-0.0153846153846154,0.),(-1.,1.),.UNSPECIFIED.)
GEOMETRIC_REPRESENTATION_ITEM()
RATIONAL_B_SPLINE_SURFACE(((1.,1.),(1.,1.),(1.,1.),(1.,1.),(1.,1.),(1.,
1.),(1.,1.),(1.,1.),(1.,1.),(1.,1.),(1.,1.),(1.,1.),(1.,1.),(1.,1.),(1.,
1.),(1.,1.),(1.,1.),(1.,1.),(1.,1.),(1.,1.),(1.,1.),(1.,1.),(1.,1.),(1.,
1.),(1.,1.),(1.,1.),(1.,1.),(1.,1.),(1.,1.),(1.,1.),(1.,1.),(1.,1.),(1.,
1.),(1.,1.),(1.,1.),(1.,1.),(1.,1.),(1.,1.),(1.,1.),(1.,1.),(1.,1.),(1.,
1.),(1.,1.),(1.,1.),(1.,1.),(1.,1.),(1.,1.),(1.,1.),(1.,1.),(1.,1.),(1.,
1.),(1.,1.),(1.,1.),(1.,1.),(1.,1.),(1.,1.),(1.,1.),(1.,1.),(1.,1.),(1.,
1.),(1.,1.),(1.,1.),(1.,1.),(1.,1.),(1.,1.),(1.,1.),(1.,1.),(1.,1.),(1.,
1.),(1.,1.)))
REPRESENTATION_ITEM('')
SURFACE()
);
#51=(
BOUNDED_CURVE()
B_SPLINE_CURVE(5,(#20848,#20849,#20850,#20851,#20852,#20853,#20854,#20855,
#20856,#20857,#20858,#20859,#20860,#20861,#20862,#20863,#20864,#20865,#20866,
#20867,#20868,#20869,#20870,#20871,#20872,#20873,#20874,#20875,#20876,#20877,
#20878,#20879,#20880,#20881,#20882,#20883,#20884,#20885,#20886,#20887,#20888,
#20889,#20890,#20891,#20892,#20893,#20894,#20895,#20896,#20897,#20898,#20899,
#20900,#20901,#20902,#20903,#20904,#20905,#20906,#20907,#20908,#20909,#20910,
#20911,#20912,#20913,#20914,#20915,#20916,#20917),.UNSPECIFIED.,.F.,.F.)
B_SPLINE_CURVE_WITH_KNOTS((6,1,1,1,1,1,1,1,1,1,1,1,1,1,1,1,1,1,1,1,1,1,
1,1,1,1,1,1,1,1,1,1,1,1,1,1,1,1,1,1,1,1,1,1,1,1,1,1,1,1,1,1,1,1,1,1,1,1,
1,1,1,1,1,1,1,6),(0.,0.0153846153846154,0.0307692307692308,0.0461538461538462,
0.0615384615384615,0.0769230769230769,0.0923076923076923,0.107692307692308,
0.123076923076923,0.138461538461538,0.153846153846154,0.169230769230769,
0.184615384615385,0.2,0.215384615384615,0.230769230769231,0.246153846153846,
0.261538461538462,0.276923076923077,0.292307692307692,0.307692307692308,
0.323076923076923,0.338461538461538,0.353846153846154,0.369230769230769,
0.384615384615385,0.4,0.415384615384615,0.430769230769231,0.446153846153846,
0.461538461538462,0.476923076923077,0.492307692307692,0.507692307692308,
0.523076923076923,0.538461538461538,0.553846153846154,0.569230769230769,
0.584615384615384,0.6,0.615384615384615,0.63076923076923,0.646153846153846,
0.661538461538461,0.676923076923076,0.692307692307692,0.707692307692307,
0.723076923076922,0.738461538461538,0.753846153846153,0.769230769230768,
0.784615384615384,0.799999999999999,0.815384615384614,0.83076923076923,
0.846153846153845,0.86153846153846,0.876923076923076,0.892307692307691,
0.907692307692306,0.923076923076922,0.938461538461537,0.953846153846152,
0.969230769230768,0.984615384615383,1.),.UNSPECIFIED.)
CURVE()
GEOMETRIC_REPRESENTATION_ITEM()
RATIONAL_B_SPLINE_CURVE((1.,1.,1.,1.,1.,1.,1.,1.,1.,1.,1.,1.,1.,1.,1.,1.,
1.,1.,1.,1.,1.,1.,1.,1.,1.,1.,1.,1.,1.,1.,1.,1.,1.,1.,1.,1.,1.,1.,1.,1.,
1.,1.,1.,1.,1.,1.,1.,1.,1.,1.,1.,1.,1.,1.,1.,1.,1.,1.,1.,1.,1.,1.,1.,1.,
1.,1.,1.,1.,1.,1.))
REPRESENTATION_ITEM('')
);
#52=(
BOUNDED_CURVE()
B_SPLINE_CURVE(5,(#20921,#20922,#20923,#20924,#20925,#20926,#20927,#20928,
#20929,#20930,#20931,#20932,#20933,#20934,#20935,#20936,#20937,#20938,#20939,
#20940,#20941,#20942,#20943,#20944,#20945,#20946,#20947,#20948,#20949,#20950,
#20951,#20952,#20953,#20954,#20955,#20956,#20957,#20958,#20959,#20960,#20961,
#20962,#20963,#20964,#20965,#20966,#20967,#20968,#20969,#20970,#20971,#20972,
#20973,#20974,#20975,#20976,#20977,#20978,#20979,#20980,#20981,#20982,#20983,
#20984,#20985,#20986,#20987,#20988,#20989,#20990),.UNSPECIFIED.,.F.,.F.)
B_SPLINE_CURVE_WITH_KNOTS((6,1,1,1,1,1,1,1,1,1,1,1,1,1,1,1,1,1,1,1,1,1,
1,1,1,1,1,1,1,1,1,1,1,1,1,1,1,1,1,1,1,1,1,1,1,1,1,1,1,1,1,1,1,1,1,1,1,1,
1,1,1,1,1,1,1,6),(0.,0.0153846153846154,0.0307692307692308,0.0461538461538462,
0.0615384615384615,0.0769230769230769,0.0923076923076923,0.107692307692308,
0.123076923076923,0.138461538461538,0.153846153846154,0.169230769230769,
0.184615384615385,0.2,0.215384615384615,0.230769230769231,0.246153846153846,
0.261538461538462,0.276923076923077,0.292307692307692,0.307692307692308,
0.323076923076923,0.338461538461538,0.353846153846154,0.369230769230769,
0.384615384615385,0.4,0.415384615384615,0.430769230769231,0.446153846153846,
0.461538461538462,0.476923076923077,0.492307692307692,0.507692307692308,
0.523076923076923,0.538461538461538,0.553846153846154,0.569230769230769,
0.584615384615384,0.6,0.615384615384615,0.63076923076923,0.646153846153846,
0.661538461538461,0.676923076923076,0.692307692307692,0.707692307692307,
0.723076923076922,0.738461538461538,0.753846153846153,0.769230769230768,
0.784615384615384,0.799999999999999,0.815384615384614,0.83076923076923,
0.846153846153845,0.86153846153846,0.876923076923076,0.892307692307691,
0.907692307692306,0.923076923076922,0.938461538461537,0.953846153846152,
0.969230769230768,0.984615384615383,1.),.UNSPECIFIED.)
CURVE()
GEOMETRIC_REPRESENTATION_ITEM()
RATIONAL_B_SPLINE_CURVE((1.,1.,1.,1.,1.,1.,1.,1.,1.,1.,1.,1.,1.,1.,1.,1.,
1.,1.,1.,1.,1.,1.,1.,1.,1.,1.,1.,1.,1.,1.,1.,1.,1.,1.,1.,1.,1.,1.,1.,1.,
1.,1.,1.,1.,1.,1.,1.,1.,1.,1.,1.,1.,1.,1.,1.,1.,1.,1.,1.,1.,1.,1.,1.,1.,
1.,1.,1.,1.,1.,1.))
REPRESENTATION_ITEM('')
);
#53=(
BOUNDED_CURVE()
B_SPLINE_CURVE(5,(#20994,#20995,#20996,#20997,#20998,#20999,#21000,#21001,
#21002,#21003,#21004,#21005,#21006,#21007,#21008,#21009,#21010,#21011,#21012,
#21013,#21014,#21015,#21016,#21017,#21018,#21019,#21020,#21021,#21022,#21023,
#21024,#21025,#21026,#21027,#21028,#21029,#21030,#21031,#21032,#21033,#21034,
#21035,#21036,#21037,#21038,#21039,#21040,#21041,#21042,#21043,#21044,#21045,
#21046,#21047,#21048,#21049,#21050,#21051,#21052,#21053,#21054,#21055,#21056,
#21057,#21058,#21059,#21060,#21061,#21062,#21063),.UNSPECIFIED.,.F.,.F.)
B_SPLINE_CURVE_WITH_KNOTS((6,1,1,1,1,1,1,1,1,1,1,1,1,1,1,1,1,1,1,1,1,1,
1,1,1,1,1,1,1,1,1,1,1,1,1,1,1,1,1,1,1,1,1,1,1,1,1,1,1,1,1,1,1,1,1,1,1,1,
1,1,1,1,1,1,1,6),(0.,0.0153846153846154,0.0307692307692308,0.0461538461538462,
0.0615384615384615,0.0769230769230769,0.0923076923076923,0.107692307692308,
0.123076923076923,0.138461538461538,0.153846153846154,0.169230769230769,
0.184615384615385,0.2,0.215384615384615,0.230769230769231,0.246153846153846,
0.261538461538462,0.276923076923077,0.292307692307692,0.307692307692308,
0.323076923076923,0.338461538461538,0.353846153846154,0.369230769230769,
0.384615384615385,0.4,0.415384615384615,0.430769230769231,0.446153846153846,
0.461538461538462,0.476923076923077,0.492307692307692,0.507692307692308,
0.523076923076923,0.538461538461538,0.553846153846154,0.569230769230769,
0.584615384615384,0.6,0.615384615384615,0.63076923076923,0.646153846153846,
0.661538461538461,0.676923076923076,0.692307692307692,0.707692307692307,
0.723076923076922,0.738461538461538,0.753846153846153,0.769230769230768,
0.784615384615384,0.799999999999999,0.815384615384614,0.83076923076923,
0.846153846153845,0.86153846153846,0.876923076923076,0.892307692307691,
0.907692307692306,0.923076923076922,0.938461538461537,0.953846153846152,
0.969230769230768,0.984615384615383,1.),.UNSPECIFIED.)
CURVE()
GEOMETRIC_REPRESENTATION_ITEM()
RATIONAL_B_SPLINE_CURVE((1.,1.,1.,1.,1.,1.,1.,1.,1.,1.,1.,1.,1.,1.,1.,1.,
1.,1.,1.,1.,1.,1.,1.,1.,1.,1.,1.,1.,1.,1.,1.,1.,1.,1.,1.,1.,1.,1.,1.,1.,
1.,1.,1.,1.,1.,1.,1.,1.,1.,1.,1.,1.,1.,1.,1.,1.,1.,1.,1.,1.,1.,1.,1.,1.,
1.,1.,1.,1.,1.,1.))
REPRESENTATION_ITEM('')
);
#54=(
BOUNDED_CURVE()
B_SPLINE_CURVE(5,(#21067,#21068,#21069,#21070,#21071,#21072,#21073,#21074,
#21075,#21076,#21077,#21078,#21079,#21080,#21081,#21082,#21083,#21084,#21085,
#21086,#21087,#21088,#21089,#21090,#21091,#21092,#21093,#21094,#21095,#21096,
#21097,#21098,#21099,#21100,#21101,#21102,#21103,#21104,#21105,#21106,#21107,
#21108,#21109,#21110,#21111,#21112,#21113,#21114,#21115,#21116,#21117,#21118,
#21119,#21120,#21121,#21122,#21123,#21124,#21125,#21126,#21127,#21128,#21129,
#21130,#21131,#21132,#21133,#21134,#21135,#21136),.UNSPECIFIED.,.F.,.F.)
B_SPLINE_CURVE_WITH_KNOTS((6,1,1,1,1,1,1,1,1,1,1,1,1,1,1,1,1,1,1,1,1,1,
1,1,1,1,1,1,1,1,1,1,1,1,1,1,1,1,1,1,1,1,1,1,1,1,1,1,1,1,1,1,1,1,1,1,1,1,
1,1,1,1,1,1,1,6),(0.,0.0153846153846154,0.0307692307692308,0.0461538461538462,
0.0615384615384615,0.0769230769230769,0.0923076923076923,0.107692307692308,
0.123076923076923,0.138461538461538,0.153846153846154,0.169230769230769,
0.184615384615385,0.2,0.215384615384615,0.230769230769231,0.246153846153846,
0.261538461538462,0.276923076923077,0.292307692307692,0.307692307692308,
0.323076923076923,0.338461538461538,0.353846153846154,0.369230769230769,
0.384615384615385,0.4,0.415384615384615,0.430769230769231,0.446153846153846,
0.461538461538462,0.476923076923077,0.492307692307692,0.507692307692308,
0.523076923076923,0.538461538461538,0.553846153846154,0.569230769230769,
0.584615384615384,0.6,0.615384615384615,0.63076923076923,0.646153846153846,
0.661538461538461,0.676923076923076,0.692307692307692,0.707692307692307,
0.723076923076922,0.738461538461538,0.753846153846153,0.769230769230768,
0.784615384615384,0.799999999999999,0.815384615384614,0.83076923076923,
0.846153846153845,0.86153846153846,0.876923076923076,0.892307692307691,
0.907692307692306,0.923076923076922,0.938461538461537,0.953846153846152,
0.969230769230768,0.984615384615383,1.),.UNSPECIFIED.)
CURVE()
GEOMETRIC_REPRESENTATION_ITEM()
RATIONAL_B_SPLINE_CURVE((1.,1.,1.,1.,1.,1.,1.,1.,1.,1.,1.,1.,1.,1.,1.,1.,
1.,1.,1.,1.,1.,1.,1.,1.,1.,1.,1.,1.,1.,1.,1.,1.,1.,1.,1.,1.,1.,1.,1.,1.,
1.,1.,1.,1.,1.,1.,1.,1.,1.,1.,1.,1.,1.,1.,1.,1.,1.,1.,1.,1.,1.,1.,1.,1.,
1.,1.,1.,1.,1.,1.))
REPRESENTATION_ITEM('')
);
#55=(
BOUNDED_CURVE()
B_SPLINE_CURVE(5,(#21140,#21141,#21142,#21143,#21144,#21145,#21146,#21147,
#21148,#21149,#21150,#21151,#21152,#21153,#21154,#21155,#21156,#21157,#21158,
#21159,#21160,#21161,#21162,#21163,#21164,#21165,#21166,#21167,#21168,#21169,
#21170,#21171,#21172,#21173,#21174,#21175,#21176,#21177,#21178,#21179,#21180,
#21181,#21182,#21183,#21184,#21185,#21186,#21187,#21188,#21189,#21190,#21191,
#21192,#21193,#21194,#21195,#21196,#21197,#21198,#21199,#21200,#21201,#21202,
#21203,#21204,#21205,#21206,#21207,#21208,#21209),.UNSPECIFIED.,.F.,.F.)
B_SPLINE_CURVE_WITH_KNOTS((6,1,1,1,1,1,1,1,1,1,1,1,1,1,1,1,1,1,1,1,1,1,
1,1,1,1,1,1,1,1,1,1,1,1,1,1,1,1,1,1,1,1,1,1,1,1,1,1,1,1,1,1,1,1,1,1,1,1,
1,1,1,1,1,1,1,6),(0.,0.0153846153846154,0.0307692307692308,0.0461538461538462,
0.0615384615384615,0.0769230769230769,0.0923076923076923,0.107692307692308,
0.123076923076923,0.138461538461538,0.153846153846154,0.169230769230769,
0.184615384615385,0.2,0.215384615384615,0.230769230769231,0.246153846153846,
0.261538461538462,0.276923076923077,0.292307692307692,0.307692307692308,
0.323076923076923,0.338461538461538,0.353846153846154,0.369230769230769,
0.384615384615385,0.4,0.415384615384615,0.430769230769231,0.446153846153846,
0.461538461538462,0.476923076923077,0.492307692307692,0.507692307692308,
0.523076923076923,0.538461538461538,0.553846153846154,0.569230769230769,
0.584615384615384,0.6,0.615384615384615,0.63076923076923,0.646153846153846,
0.661538461538461,0.676923076923076,0.692307692307692,0.707692307692307,
0.723076923076922,0.738461538461538,0.753846153846153,0.769230769230768,
0.784615384615384,0.799999999999999,0.815384615384614,0.83076923076923,
0.846153846153845,0.86153846153846,0.876923076923076,0.892307692307691,
0.907692307692306,0.923076923076922,0.938461538461537,0.953846153846152,
0.969230769230768,0.984615384615383,1.),.UNSPECIFIED.)
CURVE()
GEOMETRIC_REPRESENTATION_ITEM()
RATIONAL_B_SPLINE_CURVE((1.,1.,1.,1.,1.,1.,1.,1.,1.,1.,1.,1.,1.,1.,1.,1.,
1.,1.,1.,1.,1.,1.,1.,1.,1.,1.,1.,1.,1.,1.,1.,1.,1.,1.,1.,1.,1.,1.,1.,1.,
1.,1.,1.,1.,1.,1.,1.,1.,1.,1.,1.,1.,1.,1.,1.,1.,1.,1.,1.,1.,1.,1.,1.,1.,
1.,1.,1.,1.,1.,1.))
REPRESENTATION_ITEM('')
);
#56=(
BOUNDED_CURVE()
B_SPLINE_CURVE(5,(#21213,#21214,#21215,#21216,#21217,#21218,#21219,#21220,
#21221,#21222,#21223,#21224,#21225,#21226,#21227,#21228,#21229,#21230,#21231,
#21232,#21233,#21234,#21235,#21236,#21237,#21238,#21239,#21240,#21241,#21242,
#21243,#21244,#21245,#21246,#21247,#21248,#21249,#21250,#21251,#21252,#21253,
#21254,#21255,#21256,#21257,#21258,#21259,#21260,#21261,#21262,#21263,#21264,
#21265,#21266,#21267,#21268,#21269,#21270,#21271,#21272,#21273,#21274,#21275,
#21276,#21277,#21278,#21279,#21280,#21281,#21282),.UNSPECIFIED.,.F.,.F.)
B_SPLINE_CURVE_WITH_KNOTS((6,1,1,1,1,1,1,1,1,1,1,1,1,1,1,1,1,1,1,1,1,1,
1,1,1,1,1,1,1,1,1,1,1,1,1,1,1,1,1,1,1,1,1,1,1,1,1,1,1,1,1,1,1,1,1,1,1,1,
1,1,1,1,1,1,1,6),(0.,0.0153846153846154,0.0307692307692308,0.0461538461538462,
0.0615384615384615,0.0769230769230769,0.0923076923076923,0.107692307692308,
0.123076923076923,0.138461538461538,0.153846153846154,0.169230769230769,
0.184615384615385,0.2,0.215384615384615,0.230769230769231,0.246153846153846,
0.261538461538462,0.276923076923077,0.292307692307692,0.307692307692308,
0.323076923076923,0.338461538461538,0.353846153846154,0.369230769230769,
0.384615384615385,0.4,0.415384615384615,0.430769230769231,0.446153846153846,
0.461538461538462,0.476923076923077,0.492307692307692,0.507692307692308,
0.523076923076923,0.538461538461538,0.553846153846154,0.569230769230769,
0.584615384615384,0.6,0.615384615384615,0.63076923076923,0.646153846153846,
0.661538461538461,0.676923076923076,0.692307692307692,0.707692307692307,
0.723076923076922,0.738461538461538,0.753846153846153,0.769230769230768,
0.784615384615384,0.799999999999999,0.815384615384614,0.83076923076923,
0.846153846153845,0.86153846153846,0.876923076923076,0.892307692307691,
0.907692307692306,0.923076923076922,0.938461538461537,0.953846153846152,
0.969230769230768,0.984615384615383,1.),.UNSPECIFIED.)
CURVE()
GEOMETRIC_REPRESENTATION_ITEM()
RATIONAL_B_SPLINE_CURVE((1.,1.,1.,1.,1.,1.,1.,1.,1.,1.,1.,1.,1.,1.,1.,1.,
1.,1.,1.,1.,1.,1.,1.,1.,1.,1.,1.,1.,1.,1.,1.,1.,1.,1.,1.,1.,1.,1.,1.,1.,
1.,1.,1.,1.,1.,1.,1.,1.,1.,1.,1.,1.,1.,1.,1.,1.,1.,1.,1.,1.,1.,1.,1.,1.,
1.,1.,1.,1.,1.,1.))
REPRESENTATION_ITEM('')
);
#57=(
BOUNDED_CURVE()
B_SPLINE_CURVE(5,(#21286,#21287,#21288,#21289,#21290,#21291,#21292,#21293,
#21294,#21295,#21296,#21297,#21298,#21299,#21300,#21301,#21302,#21303,#21304,
#21305,#21306,#21307,#21308,#21309,#21310,#21311,#21312,#21313,#21314,#21315,
#21316,#21317,#21318,#21319,#21320,#21321,#21322,#21323,#21324,#21325,#21326,
#21327,#21328,#21329,#21330,#21331,#21332,#21333,#21334,#21335,#21336,#21337,
#21338,#21339,#21340,#21341,#21342,#21343,#21344,#21345,#21346,#21347,#21348,
#21349,#21350,#21351,#21352,#21353,#21354,#21355),.UNSPECIFIED.,.F.,.F.)
B_SPLINE_CURVE_WITH_KNOTS((6,1,1,1,1,1,1,1,1,1,1,1,1,1,1,1,1,1,1,1,1,1,
1,1,1,1,1,1,1,1,1,1,1,1,1,1,1,1,1,1,1,1,1,1,1,1,1,1,1,1,1,1,1,1,1,1,1,1,
1,1,1,1,1,1,1,6),(0.,0.0153846153846154,0.0307692307692308,0.0461538461538462,
0.0615384615384615,0.0769230769230769,0.0923076923076923,0.107692307692308,
0.123076923076923,0.138461538461538,0.153846153846154,0.169230769230769,
0.184615384615385,0.2,0.215384615384615,0.230769230769231,0.246153846153846,
0.261538461538462,0.276923076923077,0.292307692307692,0.307692307692308,
0.323076923076923,0.338461538461538,0.353846153846154,0.369230769230769,
0.384615384615385,0.4,0.415384615384615,0.430769230769231,0.446153846153846,
0.461538461538462,0.476923076923077,0.492307692307692,0.507692307692308,
0.523076923076923,0.538461538461538,0.553846153846154,0.569230769230769,
0.584615384615384,0.6,0.615384615384615,0.63076923076923,0.646153846153846,
0.661538461538461,0.676923076923076,0.692307692307692,0.707692307692307,
0.723076923076922,0.738461538461538,0.753846153846153,0.769230769230768,
0.784615384615384,0.799999999999999,0.815384615384614,0.83076923076923,
0.846153846153845,0.86153846153846,0.876923076923076,0.892307692307691,
0.907692307692306,0.923076923076922,0.938461538461537,0.953846153846152,
0.969230769230768,0.984615384615383,1.),.UNSPECIFIED.)
CURVE()
GEOMETRIC_REPRESENTATION_ITEM()
RATIONAL_B_SPLINE_CURVE((1.,1.,1.,1.,1.,1.,1.,1.,1.,1.,1.,1.,1.,1.,1.,1.,
1.,1.,1.,1.,1.,1.,1.,1.,1.,1.,1.,1.,1.,1.,1.,1.,1.,1.,1.,1.,1.,1.,1.,1.,
1.,1.,1.,1.,1.,1.,1.,1.,1.,1.,1.,1.,1.,1.,1.,1.,1.,1.,1.,1.,1.,1.,1.,1.,
1.,1.,1.,1.,1.,1.))
REPRESENTATION_ITEM('')
);
#58=(
BOUNDED_CURVE()
B_SPLINE_CURVE(5,(#21359,#21360,#21361,#21362,#21363,#21364,#21365,#21366,
#21367,#21368,#21369,#21370,#21371,#21372,#21373,#21374,#21375,#21376,#21377,
#21378,#21379,#21380,#21381,#21382,#21383,#21384,#21385,#21386,#21387,#21388,
#21389,#21390,#21391,#21392,#21393,#21394,#21395,#21396,#21397,#21398,#21399,
#21400,#21401,#21402,#21403,#21404,#21405,#21406,#21407,#21408,#21409,#21410,
#21411,#21412,#21413,#21414,#21415,#21416,#21417,#21418,#21419,#21420,#21421,
#21422,#21423,#21424,#21425,#21426,#21427,#21428),.UNSPECIFIED.,.F.,.F.)
B_SPLINE_CURVE_WITH_KNOTS((6,1,1,1,1,1,1,1,1,1,1,1,1,1,1,1,1,1,1,1,1,1,
1,1,1,1,1,1,1,1,1,1,1,1,1,1,1,1,1,1,1,1,1,1,1,1,1,1,1,1,1,1,1,1,1,1,1,1,
1,1,1,1,1,1,1,6),(0.,0.0153846153846154,0.0307692307692308,0.0461538461538462,
0.0615384615384615,0.0769230769230769,0.0923076923076923,0.107692307692308,
0.123076923076923,0.138461538461538,0.153846153846154,0.169230769230769,
0.184615384615385,0.2,0.215384615384615,0.230769230769231,0.246153846153846,
0.261538461538462,0.276923076923077,0.292307692307692,0.307692307692308,
0.323076923076923,0.338461538461538,0.353846153846154,0.369230769230769,
0.384615384615385,0.4,0.415384615384615,0.430769230769231,0.446153846153846,
0.461538461538462,0.476923076923077,0.492307692307692,0.507692307692308,
0.523076923076923,0.538461538461538,0.553846153846154,0.569230769230769,
0.584615384615384,0.6,0.615384615384615,0.63076923076923,0.646153846153846,
0.661538461538461,0.676923076923076,0.692307692307692,0.707692307692307,
0.723076923076922,0.738461538461538,0.753846153846153,0.769230769230768,
0.784615384615384,0.799999999999999,0.815384615384614,0.83076923076923,
0.846153846153845,0.86153846153846,0.876923076923076,0.892307692307691,
0.907692307692306,0.923076923076922,0.938461538461537,0.953846153846152,
0.969230769230768,0.984615384615383,1.),.UNSPECIFIED.)
CURVE()
GEOMETRIC_REPRESENTATION_ITEM()
RATIONAL_B_SPLINE_CURVE((1.,1.,1.,1.,1.,1.,1.,1.,1.,1.,1.,1.,1.,1.,1.,1.,
1.,1.,1.,1.,1.,1.,1.,1.,1.,1.,1.,1.,1.,1.,1.,1.,1.,1.,1.,1.,1.,1.,1.,1.,
1.,1.,1.,1.,1.,1.,1.,1.,1.,1.,1.,1.,1.,1.,1.,1.,1.,1.,1.,1.,1.,1.,1.,1.,
1.,1.,1.,1.,1.,1.))
REPRESENTATION_ITEM('')
);
#59=(
BOUNDED_CURVE()
B_SPLINE_CURVE(5,(#21432,#21433,#21434,#21435,#21436,#21437,#21438,#21439,
#21440,#21441,#21442,#21443,#21444,#21445,#21446,#21447,#21448,#21449,#21450,
#21451,#21452,#21453,#21454,#21455,#21456,#21457,#21458,#21459,#21460,#21461,
#21462,#21463,#21464,#21465,#21466,#21467,#21468,#21469,#21470,#21471,#21472,
#21473,#21474,#21475,#21476,#21477,#21478,#21479,#21480,#21481,#21482,#21483,
#21484,#21485,#21486,#21487,#21488,#21489,#21490,#21491,#21492,#21493,#21494,
#21495,#21496,#21497,#21498,#21499,#21500,#21501),.UNSPECIFIED.,.F.,.F.)
B_SPLINE_CURVE_WITH_KNOTS((6,1,1,1,1,1,1,1,1,1,1,1,1,1,1,1,1,1,1,1,1,1,
1,1,1,1,1,1,1,1,1,1,1,1,1,1,1,1,1,1,1,1,1,1,1,1,1,1,1,1,1,1,1,1,1,1,1,1,
1,1,1,1,1,1,1,6),(0.,0.0153846153846154,0.0307692307692308,0.0461538461538462,
0.0615384615384615,0.0769230769230769,0.0923076923076923,0.107692307692308,
0.123076923076923,0.138461538461538,0.153846153846154,0.169230769230769,
0.184615384615385,0.2,0.215384615384615,0.230769230769231,0.246153846153846,
0.261538461538462,0.276923076923077,0.292307692307692,0.307692307692308,
0.323076923076923,0.338461538461538,0.353846153846154,0.369230769230769,
0.384615384615385,0.4,0.415384615384615,0.430769230769231,0.446153846153846,
0.461538461538462,0.476923076923077,0.492307692307692,0.507692307692308,
0.523076923076923,0.538461538461538,0.553846153846154,0.569230769230769,
0.584615384615384,0.6,0.615384615384615,0.63076923076923,0.646153846153846,
0.661538461538461,0.676923076923076,0.692307692307692,0.707692307692307,
0.723076923076922,0.738461538461538,0.753846153846153,0.769230769230768,
0.784615384615384,0.799999999999999,0.815384615384614,0.83076923076923,
0.846153846153845,0.86153846153846,0.876923076923076,0.892307692307691,
0.907692307692306,0.923076923076922,0.938461538461537,0.953846153846152,
0.969230769230768,0.984615384615383,1.),.UNSPECIFIED.)
CURVE()
GEOMETRIC_REPRESENTATION_ITEM()
RATIONAL_B_SPLINE_CURVE((1.,1.,1.,1.,1.,1.,1.,1.,1.,1.,1.,1.,1.,1.,1.,1.,
1.,1.,1.,1.,1.,1.,1.,1.,1.,1.,1.,1.,1.,1.,1.,1.,1.,1.,1.,1.,1.,1.,1.,1.,
1.,1.,1.,1.,1.,1.,1.,1.,1.,1.,1.,1.,1.,1.,1.,1.,1.,1.,1.,1.,1.,1.,1.,1.,
1.,1.,1.,1.,1.,1.))
REPRESENTATION_ITEM('')
);
#60=(
BOUNDED_CURVE()
B_SPLINE_CURVE(5,(#21505,#21506,#21507,#21508,#21509,#21510,#21511,#21512,
#21513,#21514,#21515,#21516,#21517,#21518,#21519,#21520,#21521,#21522,#21523,
#21524,#21525,#21526,#21527,#21528,#21529,#21530,#21531,#21532,#21533,#21534,
#21535,#21536,#21537,#21538,#21539,#21540,#21541,#21542,#21543,#21544,#21545,
#21546,#21547,#21548,#21549,#21550,#21551,#21552,#21553,#21554,#21555,#21556,
#21557,#21558,#21559,#21560,#21561,#21562,#21563,#21564,#21565,#21566,#21567,
#21568,#21569,#21570,#21571,#21572,#21573,#21574),.UNSPECIFIED.,.F.,.F.)
B_SPLINE_CURVE_WITH_KNOTS((6,1,1,1,1,1,1,1,1,1,1,1,1,1,1,1,1,1,1,1,1,1,
1,1,1,1,1,1,1,1,1,1,1,1,1,1,1,1,1,1,1,1,1,1,1,1,1,1,1,1,1,1,1,1,1,1,1,1,
1,1,1,1,1,1,1,6),(0.,0.0153846153846154,0.0307692307692308,0.0461538461538462,
0.0615384615384615,0.0769230769230769,0.0923076923076923,0.107692307692308,
0.123076923076923,0.138461538461538,0.153846153846154,0.169230769230769,
0.184615384615385,0.2,0.215384615384615,0.230769230769231,0.246153846153846,
0.261538461538462,0.276923076923077,0.292307692307692,0.307692307692308,
0.323076923076923,0.338461538461538,0.353846153846154,0.369230769230769,
0.384615384615385,0.4,0.415384615384615,0.430769230769231,0.446153846153846,
0.461538461538462,0.476923076923077,0.492307692307692,0.507692307692308,
0.523076923076923,0.538461538461538,0.553846153846154,0.569230769230769,
0.584615384615384,0.6,0.615384615384615,0.63076923076923,0.646153846153846,
0.661538461538461,0.676923076923076,0.692307692307692,0.707692307692307,
0.723076923076922,0.738461538461538,0.753846153846153,0.769230769230768,
0.784615384615384,0.799999999999999,0.815384615384614,0.83076923076923,
0.846153846153845,0.86153846153846,0.876923076923076,0.892307692307691,
0.907692307692306,0.923076923076922,0.938461538461537,0.953846153846152,
0.969230769230768,0.984615384615383,1.),.UNSPECIFIED.)
CURVE()
GEOMETRIC_REPRESENTATION_ITEM()
RATIONAL_B_SPLINE_CURVE((1.,1.,1.,1.,1.,1.,1.,1.,1.,1.,1.,1.,1.,1.,1.,1.,
1.,1.,1.,1.,1.,1.,1.,1.,1.,1.,1.,1.,1.,1.,1.,1.,1.,1.,1.,1.,1.,1.,1.,1.,
1.,1.,1.,1.,1.,1.,1.,1.,1.,1.,1.,1.,1.,1.,1.,1.,1.,1.,1.,1.,1.,1.,1.,1.,
1.,1.,1.,1.,1.,1.))
REPRESENTATION_ITEM('')
);
#61=(
BOUNDED_CURVE()
B_SPLINE_CURVE(5,(#21578,#21579,#21580,#21581,#21582,#21583,#21584,#21585,
#21586,#21587,#21588,#21589,#21590,#21591,#21592,#21593,#21594,#21595,#21596,
#21597,#21598,#21599,#21600,#21601,#21602,#21603,#21604,#21605,#21606,#21607,
#21608,#21609,#21610,#21611,#21612,#21613,#21614,#21615,#21616,#21617,#21618,
#21619,#21620,#21621,#21622,#21623,#21624,#21625,#21626,#21627,#21628,#21629,
#21630,#21631,#21632,#21633,#21634,#21635,#21636,#21637,#21638,#21639,#21640,
#21641,#21642,#21643,#21644,#21645,#21646,#21647),.UNSPECIFIED.,.F.,.F.)
B_SPLINE_CURVE_WITH_KNOTS((6,1,1,1,1,1,1,1,1,1,1,1,1,1,1,1,1,1,1,1,1,1,
1,1,1,1,1,1,1,1,1,1,1,1,1,1,1,1,1,1,1,1,1,1,1,1,1,1,1,1,1,1,1,1,1,1,1,1,
1,1,1,1,1,1,1,6),(0.,0.0153846153846154,0.0307692307692308,0.0461538461538462,
0.0615384615384615,0.0769230769230769,0.0923076923076923,0.107692307692308,
0.123076923076923,0.138461538461538,0.153846153846154,0.169230769230769,
0.184615384615385,0.2,0.215384615384615,0.230769230769231,0.246153846153846,
0.261538461538462,0.276923076923077,0.292307692307692,0.307692307692308,
0.323076923076923,0.338461538461538,0.353846153846154,0.369230769230769,
0.384615384615385,0.4,0.415384615384615,0.430769230769231,0.446153846153846,
0.461538461538462,0.476923076923077,0.492307692307692,0.507692307692308,
0.523076923076923,0.538461538461538,0.553846153846154,0.569230769230769,
0.584615384615384,0.6,0.615384615384615,0.63076923076923,0.646153846153846,
0.661538461538461,0.676923076923076,0.692307692307692,0.707692307692307,
0.723076923076922,0.738461538461538,0.753846153846153,0.769230769230768,
0.784615384615384,0.799999999999999,0.815384615384614,0.83076923076923,
0.846153846153845,0.86153846153846,0.876923076923076,0.892307692307691,
0.907692307692306,0.923076923076922,0.938461538461537,0.953846153846152,
0.969230769230768,0.984615384615383,1.),.UNSPECIFIED.)
CURVE()
GEOMETRIC_REPRESENTATION_ITEM()
RATIONAL_B_SPLINE_CURVE((1.,1.,1.,1.,1.,1.,1.,1.,1.,1.,1.,1.,1.,1.,1.,1.,
1.,1.,1.,1.,1.,1.,1.,1.,1.,1.,1.,1.,1.,1.,1.,1.,1.,1.,1.,1.,1.,1.,1.,1.,
1.,1.,1.,1.,1.,1.,1.,1.,1.,1.,1.,1.,1.,1.,1.,1.,1.,1.,1.,1.,1.,1.,1.,1.,
1.,1.,1.,1.,1.,1.))
REPRESENTATION_ITEM('')
);
#62=(
BOUNDED_CURVE()
B_SPLINE_CURVE(5,(#21651,#21652,#21653,#21654,#21655,#21656,#21657,#21658,
#21659,#21660,#21661,#21662,#21663,#21664,#21665,#21666,#21667,#21668,#21669,
#21670,#21671,#21672,#21673,#21674,#21675,#21676,#21677,#21678,#21679,#21680,
#21681,#21682,#21683,#21684,#21685,#21686,#21687,#21688,#21689,#21690,#21691,
#21692,#21693,#21694,#21695,#21696,#21697,#21698,#21699,#21700,#21701,#21702,
#21703,#21704,#21705,#21706,#21707,#21708,#21709,#21710,#21711,#21712,#21713,
#21714,#21715,#21716,#21717,#21718,#21719,#21720),.UNSPECIFIED.,.F.,.F.)
B_SPLINE_CURVE_WITH_KNOTS((6,1,1,1,1,1,1,1,1,1,1,1,1,1,1,1,1,1,1,1,1,1,
1,1,1,1,1,1,1,1,1,1,1,1,1,1,1,1,1,1,1,1,1,1,1,1,1,1,1,1,1,1,1,1,1,1,1,1,
1,1,1,1,1,1,1,6),(0.,0.0153846153846154,0.0307692307692308,0.0461538461538462,
0.0615384615384615,0.0769230769230769,0.0923076923076923,0.107692307692308,
0.123076923076923,0.138461538461538,0.153846153846154,0.169230769230769,
0.184615384615385,0.2,0.215384615384615,0.230769230769231,0.246153846153846,
0.261538461538462,0.276923076923077,0.292307692307692,0.307692307692308,
0.323076923076923,0.338461538461538,0.353846153846154,0.369230769230769,
0.384615384615385,0.4,0.415384615384615,0.430769230769231,0.446153846153846,
0.461538461538462,0.476923076923077,0.492307692307692,0.507692307692308,
0.523076923076923,0.538461538461538,0.553846153846154,0.569230769230769,
0.584615384615384,0.6,0.615384615384615,0.63076923076923,0.646153846153846,
0.661538461538461,0.676923076923076,0.692307692307692,0.707692307692307,
0.723076923076922,0.738461538461538,0.753846153846153,0.769230769230768,
0.784615384615384,0.799999999999999,0.815384615384614,0.83076923076923,
0.846153846153845,0.86153846153846,0.876923076923076,0.892307692307691,
0.907692307692306,0.923076923076922,0.938461538461537,0.953846153846152,
0.969230769230768,0.984615384615383,1.),.UNSPECIFIED.)
CURVE()
GEOMETRIC_REPRESENTATION_ITEM()
RATIONAL_B_SPLINE_CURVE((1.,1.,1.,1.,1.,1.,1.,1.,1.,1.,1.,1.,1.,1.,1.,1.,
1.,1.,1.,1.,1.,1.,1.,1.,1.,1.,1.,1.,1.,1.,1.,1.,1.,1.,1.,1.,1.,1.,1.,1.,
1.,1.,1.,1.,1.,1.,1.,1.,1.,1.,1.,1.,1.,1.,1.,1.,1.,1.,1.,1.,1.,1.,1.,1.,
1.,1.,1.,1.,1.,1.))
REPRESENTATION_ITEM('')
);
#63=(
BOUNDED_CURVE()
B_SPLINE_CURVE(5,(#21724,#21725,#21726,#21727,#21728,#21729,#21730,#21731,
#21732,#21733,#21734,#21735,#21736,#21737,#21738,#21739,#21740,#21741,#21742,
#21743,#21744,#21745,#21746,#21747,#21748,#21749,#21750,#21751,#21752,#21753,
#21754,#21755,#21756,#21757,#21758,#21759,#21760,#21761,#21762,#21763,#21764,
#21765,#21766,#21767,#21768,#21769,#21770,#21771,#21772,#21773,#21774,#21775,
#21776,#21777,#21778,#21779,#21780,#21781,#21782,#21783,#21784,#21785,#21786,
#21787,#21788,#21789,#21790,#21791,#21792,#21793),.UNSPECIFIED.,.F.,.F.)
B_SPLINE_CURVE_WITH_KNOTS((6,1,1,1,1,1,1,1,1,1,1,1,1,1,1,1,1,1,1,1,1,1,
1,1,1,1,1,1,1,1,1,1,1,1,1,1,1,1,1,1,1,1,1,1,1,1,1,1,1,1,1,1,1,1,1,1,1,1,
1,1,1,1,1,1,1,6),(0.,0.0153846153846154,0.0307692307692308,0.0461538461538462,
0.0615384615384615,0.0769230769230769,0.0923076923076923,0.107692307692308,
0.123076923076923,0.138461538461538,0.153846153846154,0.169230769230769,
0.184615384615385,0.2,0.215384615384615,0.230769230769231,0.246153846153846,
0.261538461538462,0.276923076923077,0.292307692307692,0.307692307692308,
0.323076923076923,0.338461538461538,0.353846153846154,0.369230769230769,
0.384615384615385,0.4,0.415384615384615,0.430769230769231,0.446153846153846,
0.461538461538462,0.476923076923077,0.492307692307692,0.507692307692308,
0.523076923076923,0.538461538461538,0.553846153846154,0.569230769230769,
0.584615384615384,0.6,0.615384615384615,0.63076923076923,0.646153846153846,
0.661538461538461,0.676923076923076,0.692307692307692,0.707692307692307,
0.723076923076922,0.738461538461538,0.753846153846153,0.769230769230768,
0.784615384615384,0.799999999999999,0.815384615384614,0.83076923076923,
0.846153846153845,0.86153846153846,0.876923076923076,0.892307692307691,
0.907692307692306,0.923076923076922,0.938461538461537,0.953846153846152,
0.969230769230768,0.984615384615383,1.),.UNSPECIFIED.)
CURVE()
GEOMETRIC_REPRESENTATION_ITEM()
RATIONAL_B_SPLINE_CURVE((1.,1.,1.,1.,1.,1.,1.,1.,1.,1.,1.,1.,1.,1.,1.,1.,
1.,1.,1.,1.,1.,1.,1.,1.,1.,1.,1.,1.,1.,1.,1.,1.,1.,1.,1.,1.,1.,1.,1.,1.,
1.,1.,1.,1.,1.,1.,1.,1.,1.,1.,1.,1.,1.,1.,1.,1.,1.,1.,1.,1.,1.,1.,1.,1.,
1.,1.,1.,1.,1.,1.))
REPRESENTATION_ITEM('')
);
#64=(
BOUNDED_CURVE()
B_SPLINE_CURVE(5,(#21797,#21798,#21799,#21800,#21801,#21802,#21803,#21804,
#21805,#21806,#21807,#21808,#21809,#21810,#21811,#21812,#21813,#21814,#21815,
#21816,#21817,#21818,#21819,#21820,#21821,#21822,#21823,#21824,#21825,#21826,
#21827,#21828,#21829,#21830,#21831,#21832,#21833,#21834,#21835,#21836,#21837,
#21838,#21839,#21840,#21841,#21842,#21843,#21844,#21845,#21846,#21847,#21848,
#21849,#21850,#21851,#21852,#21853,#21854,#21855,#21856,#21857,#21858,#21859,
#21860,#21861,#21862,#21863,#21864,#21865,#21866),.UNSPECIFIED.,.F.,.F.)
B_SPLINE_CURVE_WITH_KNOTS((6,1,1,1,1,1,1,1,1,1,1,1,1,1,1,1,1,1,1,1,1,1,
1,1,1,1,1,1,1,1,1,1,1,1,1,1,1,1,1,1,1,1,1,1,1,1,1,1,1,1,1,1,1,1,1,1,1,1,
1,1,1,1,1,1,1,6),(0.,0.0153846153846154,0.0307692307692308,0.0461538461538462,
0.0615384615384615,0.0769230769230769,0.0923076923076923,0.107692307692308,
0.123076923076923,0.138461538461538,0.153846153846154,0.169230769230769,
0.184615384615385,0.2,0.215384615384615,0.230769230769231,0.246153846153846,
0.261538461538462,0.276923076923077,0.292307692307692,0.307692307692308,
0.323076923076923,0.338461538461538,0.353846153846154,0.369230769230769,
0.384615384615385,0.4,0.415384615384615,0.430769230769231,0.446153846153846,
0.461538461538462,0.476923076923077,0.492307692307692,0.507692307692308,
0.523076923076923,0.538461538461538,0.553846153846154,0.569230769230769,
0.584615384615384,0.6,0.615384615384615,0.63076923076923,0.646153846153846,
0.661538461538461,0.676923076923076,0.692307692307692,0.707692307692307,
0.723076923076922,0.738461538461538,0.753846153846153,0.769230769230768,
0.784615384615384,0.799999999999999,0.815384615384614,0.83076923076923,
0.846153846153845,0.86153846153846,0.876923076923076,0.892307692307691,
0.907692307692306,0.923076923076922,0.938461538461537,0.953846153846152,
0.969230769230768,0.984615384615383,1.),.UNSPECIFIED.)
CURVE()
GEOMETRIC_REPRESENTATION_ITEM()
RATIONAL_B_SPLINE_CURVE((1.,1.,1.,1.,1.,1.,1.,1.,1.,1.,1.,1.,1.,1.,1.,1.,
1.,1.,1.,1.,1.,1.,1.,1.,1.,1.,1.,1.,1.,1.,1.,1.,1.,1.,1.,1.,1.,1.,1.,1.,
1.,1.,1.,1.,1.,1.,1.,1.,1.,1.,1.,1.,1.,1.,1.,1.,1.,1.,1.,1.,1.,1.,1.,1.,
1.,1.,1.,1.,1.,1.))
REPRESENTATION_ITEM('')
);
#65=(
BOUNDED_CURVE()
B_SPLINE_CURVE(5,(#21870,#21871,#21872,#21873,#21874,#21875,#21876,#21877,
#21878,#21879,#21880,#21881,#21882,#21883,#21884,#21885,#21886,#21887,#21888,
#21889,#21890,#21891,#21892,#21893,#21894,#21895,#21896,#21897,#21898,#21899,
#21900,#21901,#21902,#21903,#21904,#21905,#21906,#21907,#21908,#21909,#21910,
#21911,#21912,#21913,#21914,#21915,#21916,#21917,#21918,#21919,#21920,#21921,
#21922,#21923,#21924,#21925,#21926,#21927,#21928,#21929,#21930,#21931,#21932,
#21933,#21934,#21935,#21936,#21937,#21938,#21939),.UNSPECIFIED.,.F.,.F.)
B_SPLINE_CURVE_WITH_KNOTS((6,1,1,1,1,1,1,1,1,1,1,1,1,1,1,1,1,1,1,1,1,1,
1,1,1,1,1,1,1,1,1,1,1,1,1,1,1,1,1,1,1,1,1,1,1,1,1,1,1,1,1,1,1,1,1,1,1,1,
1,1,1,1,1,1,1,6),(0.,0.0153846153846154,0.0307692307692308,0.0461538461538462,
0.0615384615384615,0.0769230769230769,0.0923076923076923,0.107692307692308,
0.123076923076923,0.138461538461538,0.153846153846154,0.169230769230769,
0.184615384615385,0.2,0.215384615384615,0.230769230769231,0.246153846153846,
0.261538461538462,0.276923076923077,0.292307692307692,0.307692307692308,
0.323076923076923,0.338461538461538,0.353846153846154,0.369230769230769,
0.384615384615385,0.4,0.415384615384615,0.430769230769231,0.446153846153846,
0.461538461538462,0.476923076923077,0.492307692307692,0.507692307692308,
0.523076923076923,0.538461538461538,0.553846153846154,0.569230769230769,
0.584615384615384,0.6,0.615384615384615,0.63076923076923,0.646153846153846,
0.661538461538461,0.676923076923076,0.692307692307692,0.707692307692307,
0.723076923076922,0.738461538461538,0.753846153846153,0.769230769230768,
0.784615384615384,0.799999999999999,0.815384615384614,0.83076923076923,
0.846153846153845,0.86153846153846,0.876923076923076,0.892307692307691,
0.907692307692306,0.923076923076922,0.938461538461537,0.953846153846152,
0.969230769230768,0.984615384615383,1.),.UNSPECIFIED.)
CURVE()
GEOMETRIC_REPRESENTATION_ITEM()
RATIONAL_B_SPLINE_CURVE((1.,1.,1.,1.,1.,1.,1.,1.,1.,1.,1.,1.,1.,1.,1.,1.,
1.,1.,1.,1.,1.,1.,1.,1.,1.,1.,1.,1.,1.,1.,1.,1.,1.,1.,1.,1.,1.,1.,1.,1.,
1.,1.,1.,1.,1.,1.,1.,1.,1.,1.,1.,1.,1.,1.,1.,1.,1.,1.,1.,1.,1.,1.,1.,1.,
1.,1.,1.,1.,1.,1.))
REPRESENTATION_ITEM('')
);
#66=(
BOUNDED_CURVE()
B_SPLINE_CURVE(5,(#21943,#21944,#21945,#21946,#21947,#21948,#21949,#21950,
#21951,#21952,#21953,#21954,#21955,#21956,#21957,#21958,#21959,#21960,#21961,
#21962,#21963,#21964,#21965,#21966,#21967,#21968,#21969,#21970,#21971,#21972,
#21973,#21974,#21975,#21976,#21977,#21978,#21979,#21980,#21981,#21982,#21983,
#21984,#21985,#21986,#21987,#21988,#21989,#21990,#21991,#21992,#21993,#21994,
#21995,#21996,#21997,#21998,#21999,#22000,#22001,#22002,#22003,#22004,#22005,
#22006,#22007,#22008,#22009,#22010,#22011,#22012),.UNSPECIFIED.,.F.,.F.)
B_SPLINE_CURVE_WITH_KNOTS((6,1,1,1,1,1,1,1,1,1,1,1,1,1,1,1,1,1,1,1,1,1,
1,1,1,1,1,1,1,1,1,1,1,1,1,1,1,1,1,1,1,1,1,1,1,1,1,1,1,1,1,1,1,1,1,1,1,1,
1,1,1,1,1,1,1,6),(0.,0.0153846153846154,0.0307692307692308,0.0461538461538462,
0.0615384615384615,0.0769230769230769,0.0923076923076923,0.107692307692308,
0.123076923076923,0.138461538461538,0.153846153846154,0.169230769230769,
0.184615384615385,0.2,0.215384615384615,0.230769230769231,0.246153846153846,
0.261538461538462,0.276923076923077,0.292307692307692,0.307692307692308,
0.323076923076923,0.338461538461538,0.353846153846154,0.369230769230769,
0.384615384615385,0.4,0.415384615384615,0.430769230769231,0.446153846153846,
0.461538461538462,0.476923076923077,0.492307692307692,0.507692307692308,
0.523076923076923,0.538461538461538,0.553846153846154,0.569230769230769,
0.584615384615384,0.6,0.615384615384615,0.63076923076923,0.646153846153846,
0.661538461538461,0.676923076923076,0.692307692307692,0.707692307692307,
0.723076923076922,0.738461538461538,0.753846153846153,0.769230769230768,
0.784615384615384,0.799999999999999,0.815384615384614,0.83076923076923,
0.846153846153845,0.86153846153846,0.876923076923076,0.892307692307691,
0.907692307692306,0.923076923076922,0.938461538461537,0.953846153846152,
0.969230769230768,0.984615384615383,1.),.UNSPECIFIED.)
CURVE()
GEOMETRIC_REPRESENTATION_ITEM()
RATIONAL_B_SPLINE_CURVE((1.,1.,1.,1.,1.,1.,1.,1.,1.,1.,1.,1.,1.,1.,1.,1.,
1.,1.,1.,1.,1.,1.,1.,1.,1.,1.,1.,1.,1.,1.,1.,1.,1.,1.,1.,1.,1.,1.,1.,1.,
1.,1.,1.,1.,1.,1.,1.,1.,1.,1.,1.,1.,1.,1.,1.,1.,1.,1.,1.,1.,1.,1.,1.,1.,
1.,1.,1.,1.,1.,1.))
REPRESENTATION_ITEM('')
);
#67=(
BOUNDED_CURVE()
B_SPLINE_CURVE(5,(#22016,#22017,#22018,#22019,#22020,#22021,#22022,#22023,
#22024,#22025,#22026,#22027,#22028,#22029,#22030,#22031,#22032,#22033,#22034,
#22035,#22036,#22037,#22038,#22039,#22040,#22041,#22042,#22043,#22044,#22045,
#22046,#22047,#22048,#22049,#22050,#22051,#22052,#22053,#22054,#22055,#22056,
#22057,#22058,#22059,#22060,#22061,#22062,#22063,#22064,#22065,#22066,#22067,
#22068,#22069,#22070,#22071,#22072,#22073,#22074,#22075,#22076,#22077,#22078,
#22079,#22080,#22081,#22082,#22083,#22084,#22085),.UNSPECIFIED.,.F.,.F.)
B_SPLINE_CURVE_WITH_KNOTS((6,1,1,1,1,1,1,1,1,1,1,1,1,1,1,1,1,1,1,1,1,1,
1,1,1,1,1,1,1,1,1,1,1,1,1,1,1,1,1,1,1,1,1,1,1,1,1,1,1,1,1,1,1,1,1,1,1,1,
1,1,1,1,1,1,1,6),(0.,0.0153846153846154,0.0307692307692308,0.0461538461538462,
0.0615384615384615,0.0769230769230769,0.0923076923076923,0.107692307692308,
0.123076923076923,0.138461538461538,0.153846153846154,0.169230769230769,
0.184615384615385,0.2,0.215384615384615,0.230769230769231,0.246153846153846,
0.261538461538462,0.276923076923077,0.292307692307692,0.307692307692308,
0.323076923076923,0.338461538461538,0.353846153846154,0.369230769230769,
0.384615384615385,0.4,0.415384615384615,0.430769230769231,0.446153846153846,
0.461538461538462,0.476923076923077,0.492307692307692,0.507692307692308,
0.523076923076923,0.538461538461538,0.553846153846154,0.569230769230769,
0.584615384615384,0.6,0.615384615384615,0.63076923076923,0.646153846153846,
0.661538461538461,0.676923076923076,0.692307692307692,0.707692307692307,
0.723076923076922,0.738461538461538,0.753846153846153,0.769230769230768,
0.784615384615384,0.799999999999999,0.815384615384614,0.83076923076923,
0.846153846153845,0.86153846153846,0.876923076923076,0.892307692307691,
0.907692307692306,0.923076923076922,0.938461538461537,0.953846153846152,
0.969230769230768,0.984615384615383,1.),.UNSPECIFIED.)
CURVE()
GEOMETRIC_REPRESENTATION_ITEM()
RATIONAL_B_SPLINE_CURVE((1.,1.,1.,1.,1.,1.,1.,1.,1.,1.,1.,1.,1.,1.,1.,1.,
1.,1.,1.,1.,1.,1.,1.,1.,1.,1.,1.,1.,1.,1.,1.,1.,1.,1.,1.,1.,1.,1.,1.,1.,
1.,1.,1.,1.,1.,1.,1.,1.,1.,1.,1.,1.,1.,1.,1.,1.,1.,1.,1.,1.,1.,1.,1.,1.,
1.,1.,1.,1.,1.,1.))
REPRESENTATION_ITEM('')
);
#68=(
BOUNDED_CURVE()
B_SPLINE_CURVE(5,(#22089,#22090,#22091,#22092,#22093,#22094,#22095,#22096,
#22097,#22098,#22099,#22100,#22101,#22102,#22103,#22104,#22105,#22106,#22107,
#22108,#22109,#22110,#22111,#22112,#22113,#22114,#22115,#22116,#22117,#22118,
#22119,#22120,#22121,#22122,#22123,#22124,#22125,#22126,#22127,#22128,#22129,
#22130,#22131,#22132,#22133,#22134,#22135,#22136,#22137,#22138,#22139,#22140,
#22141,#22142,#22143,#22144,#22145,#22146,#22147,#22148,#22149,#22150,#22151,
#22152,#22153,#22154,#22155,#22156,#22157,#22158),.UNSPECIFIED.,.F.,.F.)
B_SPLINE_CURVE_WITH_KNOTS((6,1,1,1,1,1,1,1,1,1,1,1,1,1,1,1,1,1,1,1,1,1,
1,1,1,1,1,1,1,1,1,1,1,1,1,1,1,1,1,1,1,1,1,1,1,1,1,1,1,1,1,1,1,1,1,1,1,1,
1,1,1,1,1,1,1,6),(0.,0.0153846153846154,0.0307692307692308,0.0461538461538462,
0.0615384615384615,0.0769230769230769,0.0923076923076923,0.107692307692308,
0.123076923076923,0.138461538461538,0.153846153846154,0.169230769230769,
0.184615384615385,0.2,0.215384615384615,0.230769230769231,0.246153846153846,
0.261538461538462,0.276923076923077,0.292307692307692,0.307692307692308,
0.323076923076923,0.338461538461538,0.353846153846154,0.369230769230769,
0.384615384615385,0.4,0.415384615384615,0.430769230769231,0.446153846153846,
0.461538461538462,0.476923076923077,0.492307692307692,0.507692307692308,
0.523076923076923,0.538461538461538,0.553846153846154,0.569230769230769,
0.584615384615384,0.6,0.615384615384615,0.63076923076923,0.646153846153846,
0.661538461538461,0.676923076923076,0.692307692307692,0.707692307692307,
0.723076923076922,0.738461538461538,0.753846153846153,0.769230769230768,
0.784615384615384,0.799999999999999,0.815384615384614,0.83076923076923,
0.846153846153845,0.86153846153846,0.876923076923076,0.892307692307691,
0.907692307692306,0.923076923076922,0.938461538461537,0.953846153846152,
0.969230769230768,0.984615384615383,1.),.UNSPECIFIED.)
CURVE()
GEOMETRIC_REPRESENTATION_ITEM()
RATIONAL_B_SPLINE_CURVE((1.,1.,1.,1.,1.,1.,1.,1.,1.,1.,1.,1.,1.,1.,1.,1.,
1.,1.,1.,1.,1.,1.,1.,1.,1.,1.,1.,1.,1.,1.,1.,1.,1.,1.,1.,1.,1.,1.,1.,1.,
1.,1.,1.,1.,1.,1.,1.,1.,1.,1.,1.,1.,1.,1.,1.,1.,1.,1.,1.,1.,1.,1.,1.,1.,
1.,1.,1.,1.,1.,1.))
REPRESENTATION_ITEM('')
);
#69=(
BOUNDED_CURVE()
B_SPLINE_CURVE(5,(#22162,#22163,#22164,#22165,#22166,#22167,#22168,#22169,
#22170,#22171,#22172,#22173,#22174,#22175,#22176,#22177,#22178,#22179,#22180,
#22181,#22182,#22183,#22184,#22185,#22186,#22187,#22188,#22189,#22190,#22191,
#22192,#22193,#22194,#22195,#22196,#22197,#22198,#22199,#22200,#22201,#22202,
#22203,#22204,#22205,#22206,#22207,#22208,#22209,#22210,#22211,#22212,#22213,
#22214,#22215,#22216,#22217,#22218,#22219,#22220,#22221,#22222,#22223,#22224,
#22225,#22226,#22227,#22228,#22229,#22230,#22231),.UNSPECIFIED.,.F.,.F.)
B_SPLINE_CURVE_WITH_KNOTS((6,1,1,1,1,1,1,1,1,1,1,1,1,1,1,1,1,1,1,1,1,1,
1,1,1,1,1,1,1,1,1,1,1,1,1,1,1,1,1,1,1,1,1,1,1,1,1,1,1,1,1,1,1,1,1,1,1,1,
1,1,1,1,1,1,1,6),(0.,0.0153846153846154,0.0307692307692308,0.0461538461538462,
0.0615384615384615,0.0769230769230769,0.0923076923076923,0.107692307692308,
0.123076923076923,0.138461538461538,0.153846153846154,0.169230769230769,
0.184615384615385,0.2,0.215384615384615,0.230769230769231,0.246153846153846,
0.261538461538462,0.276923076923077,0.292307692307692,0.307692307692308,
0.323076923076923,0.338461538461538,0.353846153846154,0.369230769230769,
0.384615384615385,0.4,0.415384615384615,0.430769230769231,0.446153846153846,
0.461538461538462,0.476923076923077,0.492307692307692,0.507692307692308,
0.523076923076923,0.538461538461538,0.553846153846154,0.569230769230769,
0.584615384615384,0.6,0.615384615384615,0.63076923076923,0.646153846153846,
0.661538461538461,0.676923076923076,0.692307692307692,0.707692307692307,
0.723076923076922,0.738461538461538,0.753846153846153,0.769230769230768,
0.784615384615384,0.799999999999999,0.815384615384614,0.83076923076923,
0.846153846153845,0.86153846153846,0.876923076923076,0.892307692307691,
0.907692307692306,0.923076923076922,0.938461538461537,0.953846153846152,
0.969230769230768,0.984615384615383,1.),.UNSPECIFIED.)
CURVE()
GEOMETRIC_REPRESENTATION_ITEM()
RATIONAL_B_SPLINE_CURVE((1.,1.,1.,1.,1.,1.,1.,1.,1.,1.,1.,1.,1.,1.,1.,1.,
1.,1.,1.,1.,1.,1.,1.,1.,1.,1.,1.,1.,1.,1.,1.,1.,1.,1.,1.,1.,1.,1.,1.,1.,
1.,1.,1.,1.,1.,1.,1.,1.,1.,1.,1.,1.,1.,1.,1.,1.,1.,1.,1.,1.,1.,1.,1.,1.,
1.,1.,1.,1.,1.,1.))
REPRESENTATION_ITEM('')
);
#70=(
BOUNDED_CURVE()
B_SPLINE_CURVE(5,(#22235,#22236,#22237,#22238,#22239,#22240,#22241,#22242,
#22243,#22244,#22245,#22246,#22247,#22248,#22249,#22250,#22251,#22252,#22253,
#22254,#22255,#22256,#22257,#22258,#22259,#22260,#22261,#22262,#22263,#22264,
#22265,#22266,#22267,#22268,#22269,#22270,#22271,#22272,#22273,#22274,#22275,
#22276,#22277,#22278,#22279,#22280,#22281,#22282,#22283,#22284,#22285,#22286,
#22287,#22288,#22289,#22290,#22291,#22292,#22293,#22294,#22295,#22296,#22297,
#22298,#22299,#22300,#22301,#22302,#22303,#22304),.UNSPECIFIED.,.F.,.F.)
B_SPLINE_CURVE_WITH_KNOTS((6,1,1,1,1,1,1,1,1,1,1,1,1,1,1,1,1,1,1,1,1,1,
1,1,1,1,1,1,1,1,1,1,1,1,1,1,1,1,1,1,1,1,1,1,1,1,1,1,1,1,1,1,1,1,1,1,1,1,
1,1,1,1,1,1,1,6),(0.,0.0153846153846154,0.0307692307692308,0.0461538461538462,
0.0615384615384615,0.0769230769230769,0.0923076923076923,0.107692307692308,
0.123076923076923,0.138461538461538,0.153846153846154,0.169230769230769,
0.184615384615385,0.2,0.215384615384615,0.230769230769231,0.246153846153846,
0.261538461538462,0.276923076923077,0.292307692307692,0.307692307692308,
0.323076923076923,0.338461538461538,0.353846153846154,0.369230769230769,
0.384615384615385,0.4,0.415384615384615,0.430769230769231,0.446153846153846,
0.461538461538462,0.476923076923077,0.492307692307692,0.507692307692308,
0.523076923076923,0.538461538461538,0.553846153846154,0.569230769230769,
0.584615384615384,0.6,0.615384615384615,0.63076923076923,0.646153846153846,
0.661538461538461,0.676923076923076,0.692307692307692,0.707692307692307,
0.723076923076922,0.738461538461538,0.753846153846153,0.769230769230768,
0.784615384615384,0.799999999999999,0.815384615384614,0.83076923076923,
0.846153846153845,0.86153846153846,0.876923076923076,0.892307692307691,
0.907692307692306,0.923076923076922,0.938461538461537,0.953846153846152,
0.969230769230768,0.984615384615383,1.),.UNSPECIFIED.)
CURVE()
GEOMETRIC_REPRESENTATION_ITEM()
RATIONAL_B_SPLINE_CURVE((1.,1.,1.,1.,1.,1.,1.,1.,1.,1.,1.,1.,1.,1.,1.,1.,
1.,1.,1.,1.,1.,1.,1.,1.,1.,1.,1.,1.,1.,1.,1.,1.,1.,1.,1.,1.,1.,1.,1.,1.,
1.,1.,1.,1.,1.,1.,1.,1.,1.,1.,1.,1.,1.,1.,1.,1.,1.,1.,1.,1.,1.,1.,1.,1.,
1.,1.,1.,1.,1.,1.))
REPRESENTATION_ITEM('')
);
#71=(
BOUNDED_CURVE()
B_SPLINE_CURVE(5,(#22308,#22309,#22310,#22311,#22312,#22313,#22314,#22315,
#22316,#22317,#22318,#22319,#22320,#22321,#22322,#22323,#22324,#22325,#22326,
#22327,#22328,#22329,#22330,#22331,#22332,#22333,#22334,#22335,#22336,#22337,
#22338,#22339,#22340,#22341,#22342,#22343,#22344,#22345,#22346,#22347,#22348,
#22349,#22350,#22351,#22352,#22353,#22354,#22355,#22356,#22357,#22358,#22359,
#22360,#22361,#22362,#22363,#22364,#22365,#22366,#22367,#22368,#22369,#22370,
#22371,#22372,#22373,#22374,#22375,#22376,#22377),.UNSPECIFIED.,.F.,.F.)
B_SPLINE_CURVE_WITH_KNOTS((6,1,1,1,1,1,1,1,1,1,1,1,1,1,1,1,1,1,1,1,1,1,
1,1,1,1,1,1,1,1,1,1,1,1,1,1,1,1,1,1,1,1,1,1,1,1,1,1,1,1,1,1,1,1,1,1,1,1,
1,1,1,1,1,1,1,6),(0.,0.0153846153846154,0.0307692307692308,0.0461538461538462,
0.0615384615384615,0.0769230769230769,0.0923076923076923,0.107692307692308,
0.123076923076923,0.138461538461538,0.153846153846154,0.169230769230769,
0.184615384615385,0.2,0.215384615384615,0.230769230769231,0.246153846153846,
0.261538461538462,0.276923076923077,0.292307692307692,0.307692307692308,
0.323076923076923,0.338461538461538,0.353846153846154,0.369230769230769,
0.384615384615385,0.4,0.415384615384615,0.430769230769231,0.446153846153846,
0.461538461538462,0.476923076923077,0.492307692307692,0.507692307692308,
0.523076923076923,0.538461538461538,0.553846153846154,0.569230769230769,
0.584615384615384,0.6,0.615384615384615,0.63076923076923,0.646153846153846,
0.661538461538461,0.676923076923076,0.692307692307692,0.707692307692307,
0.723076923076922,0.738461538461538,0.753846153846153,0.769230769230768,
0.784615384615384,0.799999999999999,0.815384615384614,0.83076923076923,
0.846153846153845,0.86153846153846,0.876923076923076,0.892307692307691,
0.907692307692306,0.923076923076922,0.938461538461537,0.953846153846152,
0.969230769230768,0.984615384615383,1.),.UNSPECIFIED.)
CURVE()
GEOMETRIC_REPRESENTATION_ITEM()
RATIONAL_B_SPLINE_CURVE((1.,1.,1.,1.,1.,1.,1.,1.,1.,1.,1.,1.,1.,1.,1.,1.,
1.,1.,1.,1.,1.,1.,1.,1.,1.,1.,1.,1.,1.,1.,1.,1.,1.,1.,1.,1.,1.,1.,1.,1.,
1.,1.,1.,1.,1.,1.,1.,1.,1.,1.,1.,1.,1.,1.,1.,1.,1.,1.,1.,1.,1.,1.,1.,1.,
1.,1.,1.,1.,1.,1.))
REPRESENTATION_ITEM('')
);
#72=(
BOUNDED_CURVE()
B_SPLINE_CURVE(5,(#22381,#22382,#22383,#22384,#22385,#22386,#22387,#22388,
#22389,#22390,#22391,#22392,#22393,#22394,#22395,#22396,#22397,#22398,#22399,
#22400,#22401,#22402,#22403,#22404,#22405,#22406,#22407,#22408,#22409,#22410,
#22411,#22412,#22413,#22414,#22415,#22416,#22417,#22418,#22419,#22420,#22421,
#22422,#22423,#22424,#22425,#22426,#22427,#22428,#22429,#22430,#22431,#22432,
#22433,#22434,#22435,#22436,#22437,#22438,#22439,#22440,#22441,#22442,#22443,
#22444,#22445,#22446,#22447,#22448,#22449,#22450),.UNSPECIFIED.,.F.,.F.)
B_SPLINE_CURVE_WITH_KNOTS((6,1,1,1,1,1,1,1,1,1,1,1,1,1,1,1,1,1,1,1,1,1,
1,1,1,1,1,1,1,1,1,1,1,1,1,1,1,1,1,1,1,1,1,1,1,1,1,1,1,1,1,1,1,1,1,1,1,1,
1,1,1,1,1,1,1,6),(0.,0.0153846153846154,0.0307692307692308,0.0461538461538462,
0.0615384615384615,0.0769230769230769,0.0923076923076923,0.107692307692308,
0.123076923076923,0.138461538461538,0.153846153846154,0.169230769230769,
0.184615384615385,0.2,0.215384615384615,0.230769230769231,0.246153846153846,
0.261538461538462,0.276923076923077,0.292307692307692,0.307692307692308,
0.323076923076923,0.338461538461538,0.353846153846154,0.369230769230769,
0.384615384615385,0.4,0.415384615384615,0.430769230769231,0.446153846153846,
0.461538461538462,0.476923076923077,0.492307692307692,0.507692307692308,
0.523076923076923,0.538461538461538,0.553846153846154,0.569230769230769,
0.584615384615384,0.6,0.615384615384615,0.63076923076923,0.646153846153846,
0.661538461538461,0.676923076923076,0.692307692307692,0.707692307692307,
0.723076923076922,0.738461538461538,0.753846153846153,0.769230769230768,
0.784615384615384,0.799999999999999,0.815384615384614,0.83076923076923,
0.846153846153845,0.86153846153846,0.876923076923076,0.892307692307691,
0.907692307692306,0.923076923076922,0.938461538461537,0.953846153846152,
0.969230769230768,0.984615384615383,1.),.UNSPECIFIED.)
CURVE()
GEOMETRIC_REPRESENTATION_ITEM()
RATIONAL_B_SPLINE_CURVE((1.,1.,1.,1.,1.,1.,1.,1.,1.,1.,1.,1.,1.,1.,1.,1.,
1.,1.,1.,1.,1.,1.,1.,1.,1.,1.,1.,1.,1.,1.,1.,1.,1.,1.,1.,1.,1.,1.,1.,1.,
1.,1.,1.,1.,1.,1.,1.,1.,1.,1.,1.,1.,1.,1.,1.,1.,1.,1.,1.,1.,1.,1.,1.,1.,
1.,1.,1.,1.,1.,1.))
REPRESENTATION_ITEM('')
);
#73=(
BOUNDED_CURVE()
B_SPLINE_CURVE(5,(#22454,#22455,#22456,#22457,#22458,#22459,#22460,#22461,
#22462,#22463,#22464,#22465,#22466,#22467,#22468,#22469,#22470,#22471,#22472,
#22473,#22474,#22475,#22476,#22477,#22478,#22479,#22480,#22481,#22482,#22483,
#22484,#22485,#22486,#22487,#22488,#22489,#22490,#22491,#22492,#22493,#22494,
#22495,#22496,#22497,#22498,#22499,#22500,#22501,#22502,#22503,#22504,#22505,
#22506,#22507,#22508,#22509,#22510,#22511,#22512,#22513,#22514,#22515,#22516,
#22517,#22518,#22519,#22520,#22521,#22522,#22523),.UNSPECIFIED.,.F.,.F.)
B_SPLINE_CURVE_WITH_KNOTS((6,1,1,1,1,1,1,1,1,1,1,1,1,1,1,1,1,1,1,1,1,1,
1,1,1,1,1,1,1,1,1,1,1,1,1,1,1,1,1,1,1,1,1,1,1,1,1,1,1,1,1,1,1,1,1,1,1,1,
1,1,1,1,1,1,1,6),(0.,0.0153846153846154,0.0307692307692308,0.0461538461538462,
0.0615384615384615,0.0769230769230769,0.0923076923076923,0.107692307692308,
0.123076923076923,0.138461538461538,0.153846153846154,0.169230769230769,
0.184615384615385,0.2,0.215384615384615,0.230769230769231,0.246153846153846,
0.261538461538462,0.276923076923077,0.292307692307692,0.307692307692308,
0.323076923076923,0.338461538461538,0.353846153846154,0.369230769230769,
0.384615384615385,0.4,0.415384615384615,0.430769230769231,0.446153846153846,
0.461538461538462,0.476923076923077,0.492307692307692,0.507692307692308,
0.523076923076923,0.538461538461538,0.553846153846154,0.569230769230769,
0.584615384615384,0.6,0.615384615384615,0.63076923076923,0.646153846153846,
0.661538461538461,0.676923076923076,0.692307692307692,0.707692307692307,
0.723076923076922,0.738461538461538,0.753846153846153,0.769230769230768,
0.784615384615384,0.799999999999999,0.815384615384614,0.83076923076923,
0.846153846153845,0.86153846153846,0.876923076923076,0.892307692307691,
0.907692307692306,0.923076923076922,0.938461538461537,0.953846153846152,
0.969230769230768,0.984615384615383,1.),.UNSPECIFIED.)
CURVE()
GEOMETRIC_REPRESENTATION_ITEM()
RATIONAL_B_SPLINE_CURVE((1.,1.,1.,1.,1.,1.,1.,1.,1.,1.,1.,1.,1.,1.,1.,1.,
1.,1.,1.,1.,1.,1.,1.,1.,1.,1.,1.,1.,1.,1.,1.,1.,1.,1.,1.,1.,1.,1.,1.,1.,
1.,1.,1.,1.,1.,1.,1.,1.,1.,1.,1.,1.,1.,1.,1.,1.,1.,1.,1.,1.,1.,1.,1.,1.,
1.,1.,1.,1.,1.,1.))
REPRESENTATION_ITEM('')
);
#74=(
BOUNDED_CURVE()
B_SPLINE_CURVE(5,(#22527,#22528,#22529,#22530,#22531,#22532,#22533,#22534,
#22535,#22536,#22537,#22538,#22539,#22540,#22541,#22542,#22543,#22544,#22545,
#22546,#22547,#22548,#22549,#22550,#22551,#22552,#22553,#22554,#22555,#22556,
#22557,#22558,#22559,#22560,#22561,#22562,#22563,#22564,#22565,#22566,#22567,
#22568,#22569,#22570,#22571,#22572,#22573,#22574,#22575,#22576,#22577,#22578,
#22579,#22580,#22581,#22582,#22583,#22584,#22585,#22586,#22587,#22588,#22589,
#22590,#22591,#22592,#22593,#22594,#22595,#22596),.UNSPECIFIED.,.F.,.F.)
B_SPLINE_CURVE_WITH_KNOTS((6,1,1,1,1,1,1,1,1,1,1,1,1,1,1,1,1,1,1,1,1,1,
1,1,1,1,1,1,1,1,1,1,1,1,1,1,1,1,1,1,1,1,1,1,1,1,1,1,1,1,1,1,1,1,1,1,1,1,
1,1,1,1,1,1,1,6),(0.,0.0153846153846154,0.0307692307692308,0.0461538461538462,
0.0615384615384615,0.0769230769230769,0.0923076923076923,0.107692307692308,
0.123076923076923,0.138461538461538,0.153846153846154,0.169230769230769,
0.184615384615385,0.2,0.215384615384615,0.230769230769231,0.246153846153846,
0.261538461538462,0.276923076923077,0.292307692307692,0.307692307692308,
0.323076923076923,0.338461538461538,0.353846153846154,0.369230769230769,
0.384615384615385,0.4,0.415384615384615,0.430769230769231,0.446153846153846,
0.461538461538462,0.476923076923077,0.492307692307692,0.507692307692308,
0.523076923076923,0.538461538461538,0.553846153846154,0.569230769230769,
0.584615384615384,0.6,0.615384615384615,0.63076923076923,0.646153846153846,
0.661538461538461,0.676923076923076,0.692307692307692,0.707692307692307,
0.723076923076922,0.738461538461538,0.753846153846153,0.769230769230768,
0.784615384615384,0.799999999999999,0.815384615384614,0.83076923076923,
0.846153846153845,0.86153846153846,0.876923076923076,0.892307692307691,
0.907692307692306,0.923076923076922,0.938461538461537,0.953846153846152,
0.969230769230768,0.984615384615383,1.),.UNSPECIFIED.)
CURVE()
GEOMETRIC_REPRESENTATION_ITEM()
RATIONAL_B_SPLINE_CURVE((1.,1.,1.,1.,1.,1.,1.,1.,1.,1.,1.,1.,1.,1.,1.,1.,
1.,1.,1.,1.,1.,1.,1.,1.,1.,1.,1.,1.,1.,1.,1.,1.,1.,1.,1.,1.,1.,1.,1.,1.,
1.,1.,1.,1.,1.,1.,1.,1.,1.,1.,1.,1.,1.,1.,1.,1.,1.,1.,1.,1.,1.,1.,1.,1.,
1.,1.,1.,1.,1.,1.))
REPRESENTATION_ITEM('')
);
#75=(
BOUNDED_CURVE()
B_SPLINE_CURVE(5,(#22600,#22601,#22602,#22603,#22604,#22605,#22606,#22607,
#22608,#22609,#22610,#22611,#22612,#22613,#22614,#22615,#22616,#22617,#22618,
#22619,#22620,#22621,#22622,#22623,#22624,#22625,#22626,#22627,#22628,#22629,
#22630,#22631,#22632,#22633,#22634,#22635,#22636,#22637,#22638,#22639,#22640,
#22641,#22642,#22643,#22644,#22645,#22646,#22647,#22648,#22649,#22650,#22651,
#22652,#22653,#22654,#22655,#22656,#22657,#22658,#22659,#22660,#22661,#22662,
#22663,#22664,#22665,#22666,#22667,#22668,#22669),.UNSPECIFIED.,.F.,.F.)
B_SPLINE_CURVE_WITH_KNOTS((6,1,1,1,1,1,1,1,1,1,1,1,1,1,1,1,1,1,1,1,1,1,
1,1,1,1,1,1,1,1,1,1,1,1,1,1,1,1,1,1,1,1,1,1,1,1,1,1,1,1,1,1,1,1,1,1,1,1,
1,1,1,1,1,1,1,6),(0.,0.0153846153846154,0.0307692307692308,0.0461538461538462,
0.0615384615384615,0.0769230769230769,0.0923076923076923,0.107692307692308,
0.123076923076923,0.138461538461538,0.153846153846154,0.169230769230769,
0.184615384615385,0.2,0.215384615384615,0.230769230769231,0.246153846153846,
0.261538461538462,0.276923076923077,0.292307692307692,0.307692307692308,
0.323076923076923,0.338461538461538,0.353846153846154,0.369230769230769,
0.384615384615385,0.4,0.415384615384615,0.430769230769231,0.446153846153846,
0.461538461538462,0.476923076923077,0.492307692307692,0.507692307692308,
0.523076923076923,0.538461538461538,0.553846153846154,0.569230769230769,
0.584615384615384,0.6,0.615384615384615,0.63076923076923,0.646153846153846,
0.661538461538461,0.676923076923076,0.692307692307692,0.707692307692307,
0.723076923076922,0.738461538461538,0.753846153846153,0.769230769230768,
0.784615384615384,0.799999999999999,0.815384615384614,0.83076923076923,
0.846153846153845,0.86153846153846,0.876923076923076,0.892307692307691,
0.907692307692306,0.923076923076922,0.938461538461537,0.953846153846152,
0.969230769230768,0.984615384615383,1.),.UNSPECIFIED.)
CURVE()
GEOMETRIC_REPRESENTATION_ITEM()
RATIONAL_B_SPLINE_CURVE((1.,1.,1.,1.,1.,1.,1.,1.,1.,1.,1.,1.,1.,1.,1.,1.,
1.,1.,1.,1.,1.,1.,1.,1.,1.,1.,1.,1.,1.,1.,1.,1.,1.,1.,1.,1.,1.,1.,1.,1.,
1.,1.,1.,1.,1.,1.,1.,1.,1.,1.,1.,1.,1.,1.,1.,1.,1.,1.,1.,1.,1.,1.,1.,1.,
1.,1.,1.,1.,1.,1.))
REPRESENTATION_ITEM('')
);
#76=(
BOUNDED_CURVE()
B_SPLINE_CURVE(5,(#22673,#22674,#22675,#22676,#22677,#22678,#22679,#22680,
#22681,#22682,#22683,#22684,#22685,#22686,#22687,#22688,#22689,#22690,#22691,
#22692,#22693,#22694,#22695,#22696,#22697,#22698,#22699,#22700,#22701,#22702,
#22703,#22704,#22705,#22706,#22707,#22708,#22709,#22710,#22711,#22712,#22713,
#22714,#22715,#22716,#22717,#22718,#22719,#22720,#22721,#22722,#22723,#22724,
#22725,#22726,#22727,#22728,#22729,#22730,#22731,#22732,#22733,#22734,#22735,
#22736,#22737,#22738,#22739,#22740,#22741,#22742),.UNSPECIFIED.,.F.,.F.)
B_SPLINE_CURVE_WITH_KNOTS((6,1,1,1,1,1,1,1,1,1,1,1,1,1,1,1,1,1,1,1,1,1,
1,1,1,1,1,1,1,1,1,1,1,1,1,1,1,1,1,1,1,1,1,1,1,1,1,1,1,1,1,1,1,1,1,1,1,1,
1,1,1,1,1,1,1,6),(0.,0.0153846153846154,0.0307692307692308,0.0461538461538462,
0.0615384615384615,0.0769230769230769,0.0923076923076923,0.107692307692308,
0.123076923076923,0.138461538461538,0.153846153846154,0.169230769230769,
0.184615384615385,0.2,0.215384615384615,0.230769230769231,0.246153846153846,
0.261538461538462,0.276923076923077,0.292307692307692,0.307692307692308,
0.323076923076923,0.338461538461538,0.353846153846154,0.369230769230769,
0.384615384615385,0.4,0.415384615384615,0.430769230769231,0.446153846153846,
0.461538461538462,0.476923076923077,0.492307692307692,0.507692307692308,
0.523076923076923,0.538461538461538,0.553846153846154,0.569230769230769,
0.584615384615384,0.6,0.615384615384615,0.63076923076923,0.646153846153846,
0.661538461538461,0.676923076923076,0.692307692307692,0.707692307692307,
0.723076923076922,0.738461538461538,0.753846153846153,0.769230769230768,
0.784615384615384,0.799999999999999,0.815384615384614,0.83076923076923,
0.846153846153845,0.86153846153846,0.876923076923076,0.892307692307691,
0.907692307692306,0.923076923076922,0.938461538461537,0.953846153846152,
0.969230769230768,0.984615384615383,1.),.UNSPECIFIED.)
CURVE()
GEOMETRIC_REPRESENTATION_ITEM()
RATIONAL_B_SPLINE_CURVE((1.,1.,1.,1.,1.,1.,1.,1.,1.,1.,1.,1.,1.,1.,1.,1.,
1.,1.,1.,1.,1.,1.,1.,1.,1.,1.,1.,1.,1.,1.,1.,1.,1.,1.,1.,1.,1.,1.,1.,1.,
1.,1.,1.,1.,1.,1.,1.,1.,1.,1.,1.,1.,1.,1.,1.,1.,1.,1.,1.,1.,1.,1.,1.,1.,
1.,1.,1.,1.,1.,1.))
REPRESENTATION_ITEM('')
);
#77=(
BOUNDED_CURVE()
B_SPLINE_CURVE(5,(#22746,#22747,#22748,#22749,#22750,#22751,#22752,#22753,
#22754,#22755,#22756,#22757,#22758,#22759,#22760,#22761,#22762,#22763,#22764,
#22765,#22766,#22767,#22768,#22769,#22770,#22771,#22772,#22773,#22774,#22775,
#22776,#22777,#22778,#22779,#22780,#22781,#22782,#22783,#22784,#22785,#22786,
#22787,#22788,#22789,#22790,#22791,#22792,#22793,#22794,#22795,#22796,#22797,
#22798,#22799,#22800,#22801,#22802,#22803,#22804,#22805,#22806,#22807,#22808,
#22809,#22810,#22811,#22812,#22813,#22814,#22815),.UNSPECIFIED.,.F.,.F.)
B_SPLINE_CURVE_WITH_KNOTS((6,1,1,1,1,1,1,1,1,1,1,1,1,1,1,1,1,1,1,1,1,1,
1,1,1,1,1,1,1,1,1,1,1,1,1,1,1,1,1,1,1,1,1,1,1,1,1,1,1,1,1,1,1,1,1,1,1,1,
1,1,1,1,1,1,1,6),(0.,0.0153846153846154,0.0307692307692308,0.0461538461538462,
0.0615384615384615,0.0769230769230769,0.0923076923076923,0.107692307692308,
0.123076923076923,0.138461538461538,0.153846153846154,0.169230769230769,
0.184615384615385,0.2,0.215384615384615,0.230769230769231,0.246153846153846,
0.261538461538462,0.276923076923077,0.292307692307692,0.307692307692308,
0.323076923076923,0.338461538461538,0.353846153846154,0.369230769230769,
0.384615384615385,0.4,0.415384615384615,0.430769230769231,0.446153846153846,
0.461538461538462,0.476923076923077,0.492307692307692,0.507692307692308,
0.523076923076923,0.538461538461538,0.553846153846154,0.569230769230769,
0.584615384615384,0.6,0.615384615384615,0.63076923076923,0.646153846153846,
0.661538461538461,0.676923076923076,0.692307692307692,0.707692307692307,
0.723076923076922,0.738461538461538,0.753846153846153,0.769230769230768,
0.784615384615384,0.799999999999999,0.815384615384614,0.83076923076923,
0.846153846153845,0.86153846153846,0.876923076923076,0.892307692307691,
0.907692307692306,0.923076923076922,0.938461538461537,0.953846153846152,
0.969230769230768,0.984615384615383,1.),.UNSPECIFIED.)
CURVE()
GEOMETRIC_REPRESENTATION_ITEM()
RATIONAL_B_SPLINE_CURVE((1.,1.,1.,1.,1.,1.,1.,1.,1.,1.,1.,1.,1.,1.,1.,1.,
1.,1.,1.,1.,1.,1.,1.,1.,1.,1.,1.,1.,1.,1.,1.,1.,1.,1.,1.,1.,1.,1.,1.,1.,
1.,1.,1.,1.,1.,1.,1.,1.,1.,1.,1.,1.,1.,1.,1.,1.,1.,1.,1.,1.,1.,1.,1.,1.,
1.,1.,1.,1.,1.,1.))
REPRESENTATION_ITEM('')
);
#78=(
BOUNDED_CURVE()
B_SPLINE_CURVE(5,(#22819,#22820,#22821,#22822,#22823,#22824,#22825,#22826,
#22827,#22828,#22829,#22830,#22831,#22832,#22833,#22834,#22835,#22836,#22837,
#22838,#22839,#22840,#22841,#22842,#22843,#22844,#22845,#22846,#22847,#22848,
#22849,#22850,#22851,#22852,#22853,#22854,#22855,#22856,#22857,#22858,#22859,
#22860,#22861,#22862,#22863,#22864,#22865,#22866,#22867,#22868,#22869,#22870,
#22871,#22872,#22873,#22874,#22875,#22876,#22877,#22878,#22879,#22880,#22881,
#22882,#22883,#22884,#22885,#22886,#22887,#22888),.UNSPECIFIED.,.F.,.F.)
B_SPLINE_CURVE_WITH_KNOTS((6,1,1,1,1,1,1,1,1,1,1,1,1,1,1,1,1,1,1,1,1,1,
1,1,1,1,1,1,1,1,1,1,1,1,1,1,1,1,1,1,1,1,1,1,1,1,1,1,1,1,1,1,1,1,1,1,1,1,
1,1,1,1,1,1,1,6),(0.,0.0153846153846154,0.0307692307692308,0.0461538461538462,
0.0615384615384615,0.0769230769230769,0.0923076923076923,0.107692307692308,
0.123076923076923,0.138461538461538,0.153846153846154,0.169230769230769,
0.184615384615385,0.2,0.215384615384615,0.230769230769231,0.246153846153846,
0.261538461538462,0.276923076923077,0.292307692307692,0.307692307692308,
0.323076923076923,0.338461538461538,0.353846153846154,0.369230769230769,
0.384615384615385,0.4,0.415384615384615,0.430769230769231,0.446153846153846,
0.461538461538462,0.476923076923077,0.492307692307692,0.507692307692308,
0.523076923076923,0.538461538461538,0.553846153846154,0.569230769230769,
0.584615384615384,0.6,0.615384615384615,0.63076923076923,0.646153846153846,
0.661538461538461,0.676923076923076,0.692307692307692,0.707692307692307,
0.723076923076922,0.738461538461538,0.753846153846153,0.769230769230768,
0.784615384615384,0.799999999999999,0.815384615384614,0.83076923076923,
0.846153846153845,0.86153846153846,0.876923076923076,0.892307692307691,
0.907692307692306,0.923076923076922,0.938461538461537,0.953846153846152,
0.969230769230768,0.984615384615383,1.),.UNSPECIFIED.)
CURVE()
GEOMETRIC_REPRESENTATION_ITEM()
RATIONAL_B_SPLINE_CURVE((1.,1.,1.,1.,1.,1.,1.,1.,1.,1.,1.,1.,1.,1.,1.,1.,
1.,1.,1.,1.,1.,1.,1.,1.,1.,1.,1.,1.,1.,1.,1.,1.,1.,1.,1.,1.,1.,1.,1.,1.,
1.,1.,1.,1.,1.,1.,1.,1.,1.,1.,1.,1.,1.,1.,1.,1.,1.,1.,1.,1.,1.,1.,1.,1.,
1.,1.,1.,1.,1.,1.))
REPRESENTATION_ITEM('')
);
#79=(
BOUNDED_CURVE()
B_SPLINE_CURVE(5,(#22892,#22893,#22894,#22895,#22896,#22897,#22898,#22899,
#22900,#22901,#22902,#22903,#22904,#22905,#22906,#22907,#22908,#22909,#22910,
#22911,#22912,#22913,#22914,#22915,#22916,#22917,#22918,#22919,#22920,#22921,
#22922,#22923,#22924,#22925,#22926,#22927,#22928,#22929,#22930,#22931,#22932,
#22933,#22934,#22935,#22936,#22937,#22938,#22939,#22940,#22941,#22942,#22943,
#22944,#22945,#22946,#22947,#22948,#22949,#22950,#22951,#22952,#22953,#22954,
#22955,#22956,#22957,#22958,#22959,#22960,#22961),.UNSPECIFIED.,.F.,.F.)
B_SPLINE_CURVE_WITH_KNOTS((6,1,1,1,1,1,1,1,1,1,1,1,1,1,1,1,1,1,1,1,1,1,
1,1,1,1,1,1,1,1,1,1,1,1,1,1,1,1,1,1,1,1,1,1,1,1,1,1,1,1,1,1,1,1,1,1,1,1,
1,1,1,1,1,1,1,6),(0.,0.0153846153846154,0.0307692307692308,0.0461538461538462,
0.0615384615384615,0.0769230769230769,0.0923076923076923,0.107692307692308,
0.123076923076923,0.138461538461538,0.153846153846154,0.169230769230769,
0.184615384615385,0.2,0.215384615384615,0.230769230769231,0.246153846153846,
0.261538461538462,0.276923076923077,0.292307692307692,0.307692307692308,
0.323076923076923,0.338461538461538,0.353846153846154,0.369230769230769,
0.384615384615385,0.4,0.415384615384615,0.430769230769231,0.446153846153846,
0.461538461538462,0.476923076923077,0.492307692307692,0.507692307692308,
0.523076923076923,0.538461538461538,0.553846153846154,0.569230769230769,
0.584615384615384,0.6,0.615384615384615,0.63076923076923,0.646153846153846,
0.661538461538461,0.676923076923076,0.692307692307692,0.707692307692307,
0.723076923076922,0.738461538461538,0.753846153846153,0.769230769230768,
0.784615384615384,0.799999999999999,0.815384615384614,0.83076923076923,
0.846153846153845,0.86153846153846,0.876923076923076,0.892307692307691,
0.907692307692306,0.923076923076922,0.938461538461537,0.953846153846152,
0.969230769230768,0.984615384615383,1.),.UNSPECIFIED.)
CURVE()
GEOMETRIC_REPRESENTATION_ITEM()
RATIONAL_B_SPLINE_CURVE((1.,1.,1.,1.,1.,1.,1.,1.,1.,1.,1.,1.,1.,1.,1.,1.,
1.,1.,1.,1.,1.,1.,1.,1.,1.,1.,1.,1.,1.,1.,1.,1.,1.,1.,1.,1.,1.,1.,1.,1.,
1.,1.,1.,1.,1.,1.,1.,1.,1.,1.,1.,1.,1.,1.,1.,1.,1.,1.,1.,1.,1.,1.,1.,1.,
1.,1.,1.,1.,1.,1.))
REPRESENTATION_ITEM('')
);
#80=(
BOUNDED_CURVE()
B_SPLINE_CURVE(5,(#22965,#22966,#22967,#22968,#22969,#22970,#22971,#22972,
#22973,#22974,#22975,#22976,#22977,#22978,#22979,#22980,#22981,#22982,#22983,
#22984,#22985,#22986,#22987,#22988,#22989,#22990,#22991,#22992,#22993,#22994,
#22995,#22996,#22997,#22998,#22999,#23000,#23001,#23002,#23003,#23004,#23005,
#23006,#23007,#23008,#23009,#23010,#23011,#23012,#23013,#23014,#23015,#23016,
#23017,#23018,#23019,#23020,#23021,#23022,#23023,#23024,#23025,#23026,#23027,
#23028,#23029,#23030,#23031,#23032,#23033,#23034),.UNSPECIFIED.,.F.,.F.)
B_SPLINE_CURVE_WITH_KNOTS((6,1,1,1,1,1,1,1,1,1,1,1,1,1,1,1,1,1,1,1,1,1,
1,1,1,1,1,1,1,1,1,1,1,1,1,1,1,1,1,1,1,1,1,1,1,1,1,1,1,1,1,1,1,1,1,1,1,1,
1,1,1,1,1,1,1,6),(0.,0.0153846153846154,0.0307692307692308,0.0461538461538462,
0.0615384615384615,0.0769230769230769,0.0923076923076923,0.107692307692308,
0.123076923076923,0.138461538461538,0.153846153846154,0.169230769230769,
0.184615384615385,0.2,0.215384615384615,0.230769230769231,0.246153846153846,
0.261538461538462,0.276923076923077,0.292307692307692,0.307692307692308,
0.323076923076923,0.338461538461538,0.353846153846154,0.369230769230769,
0.384615384615385,0.4,0.415384615384615,0.430769230769231,0.446153846153846,
0.461538461538462,0.476923076923077,0.492307692307692,0.507692307692308,
0.523076923076923,0.538461538461538,0.553846153846154,0.569230769230769,
0.584615384615384,0.6,0.615384615384615,0.63076923076923,0.646153846153846,
0.661538461538461,0.676923076923076,0.692307692307692,0.707692307692307,
0.723076923076922,0.738461538461538,0.753846153846153,0.769230769230768,
0.784615384615384,0.799999999999999,0.815384615384614,0.83076923076923,
0.846153846153845,0.86153846153846,0.876923076923076,0.892307692307691,
0.907692307692306,0.923076923076922,0.938461538461537,0.953846153846152,
0.969230769230768,0.984615384615383,1.),.UNSPECIFIED.)
CURVE()
GEOMETRIC_REPRESENTATION_ITEM()
RATIONAL_B_SPLINE_CURVE((1.,1.,1.,1.,1.,1.,1.,1.,1.,1.,1.,1.,1.,1.,1.,1.,
1.,1.,1.,1.,1.,1.,1.,1.,1.,1.,1.,1.,1.,1.,1.,1.,1.,1.,1.,1.,1.,1.,1.,1.,
1.,1.,1.,1.,1.,1.,1.,1.,1.,1.,1.,1.,1.,1.,1.,1.,1.,1.,1.,1.,1.,1.,1.,1.,
1.,1.,1.,1.,1.,1.))
REPRESENTATION_ITEM('')
);
#81=(
BOUNDED_CURVE()
B_SPLINE_CURVE(5,(#23038,#23039,#23040,#23041,#23042,#23043,#23044,#23045,
#23046,#23047,#23048,#23049,#23050,#23051,#23052,#23053,#23054,#23055,#23056,
#23057,#23058,#23059,#23060,#23061,#23062,#23063,#23064,#23065,#23066,#23067,
#23068,#23069,#23070,#23071,#23072,#23073,#23074,#23075,#23076,#23077,#23078,
#23079,#23080,#23081,#23082,#23083,#23084,#23085,#23086,#23087,#23088,#23089,
#23090,#23091,#23092,#23093,#23094,#23095,#23096,#23097,#23098,#23099,#23100,
#23101,#23102,#23103,#23104,#23105,#23106,#23107),.UNSPECIFIED.,.F.,.F.)
B_SPLINE_CURVE_WITH_KNOTS((6,1,1,1,1,1,1,1,1,1,1,1,1,1,1,1,1,1,1,1,1,1,
1,1,1,1,1,1,1,1,1,1,1,1,1,1,1,1,1,1,1,1,1,1,1,1,1,1,1,1,1,1,1,1,1,1,1,1,
1,1,1,1,1,1,1,6),(0.,0.0153846153846154,0.0307692307692308,0.0461538461538462,
0.0615384615384615,0.0769230769230769,0.0923076923076923,0.107692307692308,
0.123076923076923,0.138461538461538,0.153846153846154,0.169230769230769,
0.184615384615385,0.2,0.215384615384615,0.230769230769231,0.246153846153846,
0.261538461538462,0.276923076923077,0.292307692307692,0.307692307692308,
0.323076923076923,0.338461538461538,0.353846153846154,0.369230769230769,
0.384615384615385,0.4,0.415384615384615,0.430769230769231,0.446153846153846,
0.461538461538462,0.476923076923077,0.492307692307692,0.507692307692308,
0.523076923076923,0.538461538461538,0.553846153846154,0.569230769230769,
0.584615384615384,0.6,0.615384615384615,0.63076923076923,0.646153846153846,
0.661538461538461,0.676923076923076,0.692307692307692,0.707692307692307,
0.723076923076922,0.738461538461538,0.753846153846153,0.769230769230768,
0.784615384615384,0.799999999999999,0.815384615384614,0.83076923076923,
0.846153846153845,0.86153846153846,0.876923076923076,0.892307692307691,
0.907692307692306,0.923076923076922,0.938461538461537,0.953846153846152,
0.969230769230768,0.984615384615383,1.),.UNSPECIFIED.)
CURVE()
GEOMETRIC_REPRESENTATION_ITEM()
RATIONAL_B_SPLINE_CURVE((1.,1.,1.,1.,1.,1.,1.,1.,1.,1.,1.,1.,1.,1.,1.,1.,
1.,1.,1.,1.,1.,1.,1.,1.,1.,1.,1.,1.,1.,1.,1.,1.,1.,1.,1.,1.,1.,1.,1.,1.,
1.,1.,1.,1.,1.,1.,1.,1.,1.,1.,1.,1.,1.,1.,1.,1.,1.,1.,1.,1.,1.,1.,1.,1.,
1.,1.,1.,1.,1.,1.))
REPRESENTATION_ITEM('')
);
#82=(
BOUNDED_CURVE()
B_SPLINE_CURVE(5,(#23111,#23112,#23113,#23114,#23115,#23116,#23117,#23118,
#23119,#23120,#23121,#23122,#23123,#23124,#23125,#23126,#23127,#23128,#23129,
#23130,#23131,#23132,#23133,#23134,#23135,#23136,#23137,#23138,#23139,#23140,
#23141,#23142,#23143,#23144,#23145,#23146,#23147,#23148,#23149,#23150,#23151,
#23152,#23153,#23154,#23155,#23156,#23157,#23158,#23159,#23160,#23161,#23162,
#23163,#23164,#23165,#23166,#23167,#23168,#23169,#23170,#23171,#23172,#23173,
#23174,#23175,#23176,#23177,#23178,#23179,#23180),.UNSPECIFIED.,.F.,.F.)
B_SPLINE_CURVE_WITH_KNOTS((6,1,1,1,1,1,1,1,1,1,1,1,1,1,1,1,1,1,1,1,1,1,
1,1,1,1,1,1,1,1,1,1,1,1,1,1,1,1,1,1,1,1,1,1,1,1,1,1,1,1,1,1,1,1,1,1,1,1,
1,1,1,1,1,1,1,6),(0.,0.0153846153846154,0.0307692307692308,0.0461538461538462,
0.0615384615384615,0.0769230769230769,0.0923076923076923,0.107692307692308,
0.123076923076923,0.138461538461538,0.153846153846154,0.169230769230769,
0.184615384615385,0.2,0.215384615384615,0.230769230769231,0.246153846153846,
0.261538461538462,0.276923076923077,0.292307692307692,0.307692307692308,
0.323076923076923,0.338461538461538,0.353846153846154,0.369230769230769,
0.384615384615385,0.4,0.415384615384615,0.430769230769231,0.446153846153846,
0.461538461538462,0.476923076923077,0.492307692307692,0.507692307692308,
0.523076923076923,0.538461538461538,0.553846153846154,0.569230769230769,
0.584615384615384,0.6,0.615384615384615,0.63076923076923,0.646153846153846,
0.661538461538461,0.676923076923076,0.692307692307692,0.707692307692307,
0.723076923076922,0.738461538461538,0.753846153846153,0.769230769230768,
0.784615384615384,0.799999999999999,0.815384615384614,0.83076923076923,
0.846153846153845,0.86153846153846,0.876923076923076,0.892307692307691,
0.907692307692306,0.923076923076922,0.938461538461537,0.953846153846152,
0.969230769230768,0.984615384615383,1.),.UNSPECIFIED.)
CURVE()
GEOMETRIC_REPRESENTATION_ITEM()
RATIONAL_B_SPLINE_CURVE((1.,1.,1.,1.,1.,1.,1.,1.,1.,1.,1.,1.,1.,1.,1.,1.,
1.,1.,1.,1.,1.,1.,1.,1.,1.,1.,1.,1.,1.,1.,1.,1.,1.,1.,1.,1.,1.,1.,1.,1.,
1.,1.,1.,1.,1.,1.,1.,1.,1.,1.,1.,1.,1.,1.,1.,1.,1.,1.,1.,1.,1.,1.,1.,1.,
1.,1.,1.,1.,1.,1.))
REPRESENTATION_ITEM('')
);
#83=(
BOUNDED_CURVE()
B_SPLINE_CURVE(5,(#23184,#23185,#23186,#23187,#23188,#23189,#23190,#23191,
#23192,#23193,#23194,#23195,#23196,#23197,#23198,#23199,#23200,#23201,#23202,
#23203,#23204,#23205,#23206,#23207,#23208,#23209,#23210,#23211,#23212,#23213,
#23214,#23215,#23216,#23217,#23218,#23219,#23220,#23221,#23222,#23223,#23224,
#23225,#23226,#23227,#23228,#23229,#23230,#23231,#23232,#23233,#23234,#23235,
#23236,#23237,#23238,#23239,#23240,#23241,#23242,#23243,#23244,#23245,#23246,
#23247,#23248,#23249,#23250,#23251,#23252,#23253),.UNSPECIFIED.,.F.,.F.)
B_SPLINE_CURVE_WITH_KNOTS((6,1,1,1,1,1,1,1,1,1,1,1,1,1,1,1,1,1,1,1,1,1,
1,1,1,1,1,1,1,1,1,1,1,1,1,1,1,1,1,1,1,1,1,1,1,1,1,1,1,1,1,1,1,1,1,1,1,1,
1,1,1,1,1,1,1,6),(0.,0.0153846153846154,0.0307692307692308,0.0461538461538462,
0.0615384615384615,0.0769230769230769,0.0923076923076923,0.107692307692308,
0.123076923076923,0.138461538461538,0.153846153846154,0.169230769230769,
0.184615384615385,0.2,0.215384615384615,0.230769230769231,0.246153846153846,
0.261538461538462,0.276923076923077,0.292307692307692,0.307692307692308,
0.323076923076923,0.338461538461538,0.353846153846154,0.369230769230769,
0.384615384615385,0.4,0.415384615384615,0.430769230769231,0.446153846153846,
0.461538461538462,0.476923076923077,0.492307692307692,0.507692307692308,
0.523076923076923,0.538461538461538,0.553846153846154,0.569230769230769,
0.584615384615384,0.6,0.615384615384615,0.63076923076923,0.646153846153846,
0.661538461538461,0.676923076923076,0.692307692307692,0.707692307692307,
0.723076923076922,0.738461538461538,0.753846153846153,0.769230769230768,
0.784615384615384,0.799999999999999,0.815384615384614,0.83076923076923,
0.846153846153845,0.86153846153846,0.876923076923076,0.892307692307691,
0.907692307692306,0.923076923076922,0.938461538461537,0.953846153846152,
0.969230769230768,0.984615384615383,1.),.UNSPECIFIED.)
CURVE()
GEOMETRIC_REPRESENTATION_ITEM()
RATIONAL_B_SPLINE_CURVE((1.,1.,1.,1.,1.,1.,1.,1.,1.,1.,1.,1.,1.,1.,1.,1.,
1.,1.,1.,1.,1.,1.,1.,1.,1.,1.,1.,1.,1.,1.,1.,1.,1.,1.,1.,1.,1.,1.,1.,1.,
1.,1.,1.,1.,1.,1.,1.,1.,1.,1.,1.,1.,1.,1.,1.,1.,1.,1.,1.,1.,1.,1.,1.,1.,
1.,1.,1.,1.,1.,1.))
REPRESENTATION_ITEM('')
);
#84=(
BOUNDED_CURVE()
B_SPLINE_CURVE(5,(#23257,#23258,#23259,#23260,#23261,#23262,#23263,#23264,
#23265,#23266,#23267,#23268,#23269,#23270,#23271,#23272,#23273,#23274,#23275,
#23276,#23277,#23278,#23279,#23280,#23281,#23282,#23283,#23284,#23285,#23286,
#23287,#23288,#23289,#23290,#23291,#23292,#23293,#23294,#23295,#23296,#23297,
#23298,#23299,#23300,#23301,#23302,#23303,#23304,#23305,#23306,#23307,#23308,
#23309,#23310,#23311,#23312,#23313,#23314,#23315,#23316,#23317,#23318,#23319,
#23320,#23321,#23322,#23323,#23324,#23325,#23326),.UNSPECIFIED.,.F.,.F.)
B_SPLINE_CURVE_WITH_KNOTS((6,1,1,1,1,1,1,1,1,1,1,1,1,1,1,1,1,1,1,1,1,1,
1,1,1,1,1,1,1,1,1,1,1,1,1,1,1,1,1,1,1,1,1,1,1,1,1,1,1,1,1,1,1,1,1,1,1,1,
1,1,1,1,1,1,1,6),(0.,0.0153846153846154,0.0307692307692308,0.0461538461538462,
0.0615384615384615,0.0769230769230769,0.0923076923076923,0.107692307692308,
0.123076923076923,0.138461538461538,0.153846153846154,0.169230769230769,
0.184615384615385,0.2,0.215384615384615,0.230769230769231,0.246153846153846,
0.261538461538462,0.276923076923077,0.292307692307692,0.307692307692308,
0.323076923076923,0.338461538461538,0.353846153846154,0.369230769230769,
0.384615384615385,0.4,0.415384615384615,0.430769230769231,0.446153846153846,
0.461538461538462,0.476923076923077,0.492307692307692,0.507692307692308,
0.523076923076923,0.538461538461538,0.553846153846154,0.569230769230769,
0.584615384615384,0.6,0.615384615384615,0.63076923076923,0.646153846153846,
0.661538461538461,0.676923076923076,0.692307692307692,0.707692307692307,
0.723076923076922,0.738461538461538,0.753846153846153,0.769230769230768,
0.784615384615384,0.799999999999999,0.815384615384614,0.83076923076923,
0.846153846153845,0.86153846153846,0.876923076923076,0.892307692307691,
0.907692307692306,0.923076923076922,0.938461538461537,0.953846153846152,
0.969230769230768,0.984615384615383,1.),.UNSPECIFIED.)
CURVE()
GEOMETRIC_REPRESENTATION_ITEM()
RATIONAL_B_SPLINE_CURVE((1.,1.,1.,1.,1.,1.,1.,1.,1.,1.,1.,1.,1.,1.,1.,1.,
1.,1.,1.,1.,1.,1.,1.,1.,1.,1.,1.,1.,1.,1.,1.,1.,1.,1.,1.,1.,1.,1.,1.,1.,
1.,1.,1.,1.,1.,1.,1.,1.,1.,1.,1.,1.,1.,1.,1.,1.,1.,1.,1.,1.,1.,1.,1.,1.,
1.,1.,1.,1.,1.,1.))
REPRESENTATION_ITEM('')
);
#85=(
BOUNDED_CURVE()
B_SPLINE_CURVE(5,(#23330,#23331,#23332,#23333,#23334,#23335,#23336,#23337,
#23338,#23339,#23340,#23341,#23342,#23343,#23344,#23345,#23346,#23347,#23348,
#23349,#23350,#23351,#23352,#23353,#23354,#23355,#23356,#23357,#23358,#23359,
#23360,#23361,#23362,#23363,#23364,#23365,#23366,#23367,#23368,#23369,#23370,
#23371,#23372,#23373,#23374,#23375,#23376,#23377,#23378,#23379,#23380,#23381,
#23382,#23383,#23384,#23385,#23386,#23387,#23388,#23389,#23390,#23391,#23392,
#23393,#23394,#23395,#23396,#23397,#23398,#23399),.UNSPECIFIED.,.F.,.F.)
B_SPLINE_CURVE_WITH_KNOTS((6,1,1,1,1,1,1,1,1,1,1,1,1,1,1,1,1,1,1,1,1,1,
1,1,1,1,1,1,1,1,1,1,1,1,1,1,1,1,1,1,1,1,1,1,1,1,1,1,1,1,1,1,1,1,1,1,1,1,
1,1,1,1,1,1,1,6),(0.,0.0153846153846154,0.0307692307692308,0.0461538461538462,
0.0615384615384615,0.0769230769230769,0.0923076923076923,0.107692307692308,
0.123076923076923,0.138461538461538,0.153846153846154,0.169230769230769,
0.184615384615385,0.2,0.215384615384615,0.230769230769231,0.246153846153846,
0.261538461538462,0.276923076923077,0.292307692307692,0.307692307692308,
0.323076923076923,0.338461538461538,0.353846153846154,0.369230769230769,
0.384615384615385,0.4,0.415384615384615,0.430769230769231,0.446153846153846,
0.461538461538462,0.476923076923077,0.492307692307692,0.507692307692308,
0.523076923076923,0.538461538461538,0.553846153846154,0.569230769230769,
0.584615384615384,0.6,0.615384615384615,0.63076923076923,0.646153846153846,
0.661538461538461,0.676923076923076,0.692307692307692,0.707692307692307,
0.723076923076922,0.738461538461538,0.753846153846153,0.769230769230768,
0.784615384615384,0.799999999999999,0.815384615384614,0.83076923076923,
0.846153846153845,0.86153846153846,0.876923076923076,0.892307692307691,
0.907692307692306,0.923076923076922,0.938461538461537,0.953846153846152,
0.969230769230768,0.984615384615383,1.),.UNSPECIFIED.)
CURVE()
GEOMETRIC_REPRESENTATION_ITEM()
RATIONAL_B_SPLINE_CURVE((1.,1.,1.,1.,1.,1.,1.,1.,1.,1.,1.,1.,1.,1.,1.,1.,
1.,1.,1.,1.,1.,1.,1.,1.,1.,1.,1.,1.,1.,1.,1.,1.,1.,1.,1.,1.,1.,1.,1.,1.,
1.,1.,1.,1.,1.,1.,1.,1.,1.,1.,1.,1.,1.,1.,1.,1.,1.,1.,1.,1.,1.,1.,1.,1.,
1.,1.,1.,1.,1.,1.))
REPRESENTATION_ITEM('')
);
#86=(
BOUNDED_CURVE()
B_SPLINE_CURVE(5,(#23403,#23404,#23405,#23406,#23407,#23408,#23409,#23410,
#23411,#23412,#23413,#23414,#23415,#23416,#23417,#23418,#23419,#23420,#23421,
#23422,#23423,#23424,#23425,#23426,#23427,#23428,#23429,#23430,#23431,#23432,
#23433,#23434,#23435,#23436,#23437,#23438,#23439,#23440,#23441,#23442,#23443,
#23444,#23445,#23446,#23447,#23448,#23449,#23450,#23451,#23452,#23453,#23454,
#23455,#23456,#23457,#23458,#23459,#23460,#23461,#23462,#23463,#23464,#23465,
#23466,#23467,#23468,#23469,#23470,#23471,#23472),.UNSPECIFIED.,.F.,.F.)
B_SPLINE_CURVE_WITH_KNOTS((6,1,1,1,1,1,1,1,1,1,1,1,1,1,1,1,1,1,1,1,1,1,
1,1,1,1,1,1,1,1,1,1,1,1,1,1,1,1,1,1,1,1,1,1,1,1,1,1,1,1,1,1,1,1,1,1,1,1,
1,1,1,1,1,1,1,6),(0.,0.0153846153846154,0.0307692307692308,0.0461538461538462,
0.0615384615384615,0.0769230769230769,0.0923076923076923,0.107692307692308,
0.123076923076923,0.138461538461538,0.153846153846154,0.169230769230769,
0.184615384615385,0.2,0.215384615384615,0.230769230769231,0.246153846153846,
0.261538461538462,0.276923076923077,0.292307692307692,0.307692307692308,
0.323076923076923,0.338461538461538,0.353846153846154,0.369230769230769,
0.384615384615385,0.4,0.415384615384615,0.430769230769231,0.446153846153846,
0.461538461538462,0.476923076923077,0.492307692307692,0.507692307692308,
0.523076923076923,0.538461538461538,0.553846153846154,0.569230769230769,
0.584615384615384,0.6,0.615384615384615,0.63076923076923,0.646153846153846,
0.661538461538461,0.676923076923076,0.692307692307692,0.707692307692307,
0.723076923076922,0.738461538461538,0.753846153846153,0.769230769230768,
0.784615384615384,0.799999999999999,0.815384615384614,0.83076923076923,
0.846153846153845,0.86153846153846,0.876923076923076,0.892307692307691,
0.907692307692306,0.923076923076922,0.938461538461537,0.953846153846152,
0.969230769230768,0.984615384615383,1.),.UNSPECIFIED.)
CURVE()
GEOMETRIC_REPRESENTATION_ITEM()
RATIONAL_B_SPLINE_CURVE((1.,1.,1.,1.,1.,1.,1.,1.,1.,1.,1.,1.,1.,1.,1.,1.,
1.,1.,1.,1.,1.,1.,1.,1.,1.,1.,1.,1.,1.,1.,1.,1.,1.,1.,1.,1.,1.,1.,1.,1.,
1.,1.,1.,1.,1.,1.,1.,1.,1.,1.,1.,1.,1.,1.,1.,1.,1.,1.,1.,1.,1.,1.,1.,1.,
1.,1.,1.,1.,1.,1.))
REPRESENTATION_ITEM('')
);
#87=(
BOUNDED_CURVE()
B_SPLINE_CURVE(5,(#23476,#23477,#23478,#23479,#23480,#23481,#23482,#23483,
#23484,#23485,#23486,#23487,#23488,#23489,#23490,#23491,#23492,#23493,#23494,
#23495,#23496,#23497,#23498,#23499,#23500,#23501,#23502,#23503,#23504,#23505,
#23506,#23507,#23508,#23509,#23510,#23511,#23512,#23513,#23514,#23515,#23516,
#23517,#23518,#23519,#23520,#23521,#23522,#23523,#23524,#23525,#23526,#23527,
#23528,#23529,#23530,#23531,#23532,#23533,#23534,#23535,#23536,#23537,#23538,
#23539,#23540,#23541,#23542,#23543,#23544,#23545),.UNSPECIFIED.,.F.,.F.)
B_SPLINE_CURVE_WITH_KNOTS((6,1,1,1,1,1,1,1,1,1,1,1,1,1,1,1,1,1,1,1,1,1,
1,1,1,1,1,1,1,1,1,1,1,1,1,1,1,1,1,1,1,1,1,1,1,1,1,1,1,1,1,1,1,1,1,1,1,1,
1,1,1,1,1,1,1,6),(0.,0.0153846153846154,0.0307692307692308,0.0461538461538462,
0.0615384615384615,0.0769230769230769,0.0923076923076923,0.107692307692308,
0.123076923076923,0.138461538461538,0.153846153846154,0.169230769230769,
0.184615384615385,0.2,0.215384615384615,0.230769230769231,0.246153846153846,
0.261538461538462,0.276923076923077,0.292307692307692,0.307692307692308,
0.323076923076923,0.338461538461538,0.353846153846154,0.369230769230769,
0.384615384615385,0.4,0.415384615384615,0.430769230769231,0.446153846153846,
0.461538461538462,0.476923076923077,0.492307692307692,0.507692307692308,
0.523076923076923,0.538461538461538,0.553846153846154,0.569230769230769,
0.584615384615384,0.6,0.615384615384615,0.63076923076923,0.646153846153846,
0.661538461538461,0.676923076923076,0.692307692307692,0.707692307692307,
0.723076923076922,0.738461538461538,0.753846153846153,0.769230769230768,
0.784615384615384,0.799999999999999,0.815384615384614,0.83076923076923,
0.846153846153845,0.86153846153846,0.876923076923076,0.892307692307691,
0.907692307692306,0.923076923076922,0.938461538461537,0.953846153846152,
0.969230769230768,0.984615384615383,1.),.UNSPECIFIED.)
CURVE()
GEOMETRIC_REPRESENTATION_ITEM()
RATIONAL_B_SPLINE_CURVE((1.,1.,1.,1.,1.,1.,1.,1.,1.,1.,1.,1.,1.,1.,1.,1.,
1.,1.,1.,1.,1.,1.,1.,1.,1.,1.,1.,1.,1.,1.,1.,1.,1.,1.,1.,1.,1.,1.,1.,1.,
1.,1.,1.,1.,1.,1.,1.,1.,1.,1.,1.,1.,1.,1.,1.,1.,1.,1.,1.,1.,1.,1.,1.,1.,
1.,1.,1.,1.,1.,1.))
REPRESENTATION_ITEM('')
);
#88=(
BOUNDED_CURVE()
B_SPLINE_CURVE(5,(#23549,#23550,#23551,#23552,#23553,#23554,#23555,#23556,
#23557,#23558,#23559,#23560,#23561,#23562,#23563,#23564,#23565,#23566,#23567,
#23568,#23569,#23570,#23571,#23572,#23573,#23574,#23575,#23576,#23577,#23578,
#23579,#23580,#23581,#23582,#23583,#23584,#23585,#23586,#23587,#23588,#23589,
#23590,#23591,#23592,#23593,#23594,#23595,#23596,#23597,#23598,#23599,#23600,
#23601,#23602,#23603,#23604,#23605,#23606,#23607,#23608,#23609,#23610,#23611,
#23612,#23613,#23614,#23615,#23616,#23617,#23618),.UNSPECIFIED.,.F.,.F.)
B_SPLINE_CURVE_WITH_KNOTS((6,1,1,1,1,1,1,1,1,1,1,1,1,1,1,1,1,1,1,1,1,1,
1,1,1,1,1,1,1,1,1,1,1,1,1,1,1,1,1,1,1,1,1,1,1,1,1,1,1,1,1,1,1,1,1,1,1,1,
1,1,1,1,1,1,1,6),(0.,0.0153846153846154,0.0307692307692308,0.0461538461538462,
0.0615384615384615,0.0769230769230769,0.0923076923076923,0.107692307692308,
0.123076923076923,0.138461538461538,0.153846153846154,0.169230769230769,
0.184615384615385,0.2,0.215384615384615,0.230769230769231,0.246153846153846,
0.261538461538462,0.276923076923077,0.292307692307692,0.307692307692308,
0.323076923076923,0.338461538461538,0.353846153846154,0.369230769230769,
0.384615384615385,0.4,0.415384615384615,0.430769230769231,0.446153846153846,
0.461538461538462,0.476923076923077,0.492307692307692,0.507692307692308,
0.523076923076923,0.538461538461538,0.553846153846154,0.569230769230769,
0.584615384615384,0.6,0.615384615384615,0.63076923076923,0.646153846153846,
0.661538461538461,0.676923076923076,0.692307692307692,0.707692307692307,
0.723076923076922,0.738461538461538,0.753846153846153,0.769230769230768,
0.784615384615384,0.799999999999999,0.815384615384614,0.83076923076923,
0.846153846153845,0.86153846153846,0.876923076923076,0.892307692307691,
0.907692307692306,0.923076923076922,0.938461538461537,0.953846153846152,
0.969230769230768,0.984615384615383,1.),.UNSPECIFIED.)
CURVE()
GEOMETRIC_REPRESENTATION_ITEM()
RATIONAL_B_SPLINE_CURVE((1.,1.,1.,1.,1.,1.,1.,1.,1.,1.,1.,1.,1.,1.,1.,1.,
1.,1.,1.,1.,1.,1.,1.,1.,1.,1.,1.,1.,1.,1.,1.,1.,1.,1.,1.,1.,1.,1.,1.,1.,
1.,1.,1.,1.,1.,1.,1.,1.,1.,1.,1.,1.,1.,1.,1.,1.,1.,1.,1.,1.,1.,1.,1.,1.,
1.,1.,1.,1.,1.,1.))
REPRESENTATION_ITEM('')
);
#89=(
BOUNDED_CURVE()
B_SPLINE_CURVE(5,(#23622,#23623,#23624,#23625,#23626,#23627,#23628,#23629,
#23630,#23631,#23632,#23633,#23634,#23635,#23636,#23637,#23638,#23639,#23640,
#23641,#23642,#23643,#23644,#23645,#23646,#23647,#23648,#23649,#23650,#23651,
#23652,#23653,#23654,#23655,#23656,#23657,#23658,#23659,#23660,#23661,#23662,
#23663,#23664,#23665,#23666,#23667,#23668,#23669,#23670,#23671,#23672,#23673,
#23674,#23675,#23676,#23677,#23678,#23679,#23680,#23681,#23682,#23683,#23684,
#23685,#23686,#23687,#23688,#23689,#23690,#23691),.UNSPECIFIED.,.F.,.F.)
B_SPLINE_CURVE_WITH_KNOTS((6,1,1,1,1,1,1,1,1,1,1,1,1,1,1,1,1,1,1,1,1,1,
1,1,1,1,1,1,1,1,1,1,1,1,1,1,1,1,1,1,1,1,1,1,1,1,1,1,1,1,1,1,1,1,1,1,1,1,
1,1,1,1,1,1,1,6),(0.,0.0153846153846154,0.0307692307692308,0.0461538461538462,
0.0615384615384615,0.0769230769230769,0.0923076923076923,0.107692307692308,
0.123076923076923,0.138461538461538,0.153846153846154,0.169230769230769,
0.184615384615385,0.2,0.215384615384615,0.230769230769231,0.246153846153846,
0.261538461538462,0.276923076923077,0.292307692307692,0.307692307692308,
0.323076923076923,0.338461538461538,0.353846153846154,0.369230769230769,
0.384615384615385,0.4,0.415384615384615,0.430769230769231,0.446153846153846,
0.461538461538462,0.476923076923077,0.492307692307692,0.507692307692308,
0.523076923076923,0.538461538461538,0.553846153846154,0.569230769230769,
0.584615384615384,0.6,0.615384615384615,0.63076923076923,0.646153846153846,
0.661538461538461,0.676923076923076,0.692307692307692,0.707692307692307,
0.723076923076922,0.738461538461538,0.753846153846153,0.769230769230768,
0.784615384615384,0.799999999999999,0.815384615384614,0.83076923076923,
0.846153846153845,0.86153846153846,0.876923076923076,0.892307692307691,
0.907692307692306,0.923076923076922,0.938461538461537,0.953846153846152,
0.969230769230768,0.984615384615383,1.),.UNSPECIFIED.)
CURVE()
GEOMETRIC_REPRESENTATION_ITEM()
RATIONAL_B_SPLINE_CURVE((1.,1.,1.,1.,1.,1.,1.,1.,1.,1.,1.,1.,1.,1.,1.,1.,
1.,1.,1.,1.,1.,1.,1.,1.,1.,1.,1.,1.,1.,1.,1.,1.,1.,1.,1.,1.,1.,1.,1.,1.,
1.,1.,1.,1.,1.,1.,1.,1.,1.,1.,1.,1.,1.,1.,1.,1.,1.,1.,1.,1.,1.,1.,1.,1.,
1.,1.,1.,1.,1.,1.))
REPRESENTATION_ITEM('')
);
#90=(
BOUNDED_CURVE()
B_SPLINE_CURVE(5,(#23694,#23695,#23696,#23697,#23698,#23699,#23700,#23701,
#23702,#23703,#23704,#23705,#23706,#23707,#23708,#23709,#23710,#23711,#23712,
#23713,#23714,#23715,#23716,#23717,#23718,#23719,#23720,#23721,#23722,#23723,
#23724,#23725,#23726,#23727,#23728,#23729,#23730,#23731,#23732,#23733,#23734,
#23735,#23736,#23737,#23738,#23739,#23740,#23741,#23742,#23743,#23744,#23745,
#23746,#23747,#23748,#23749,#23750,#23751,#23752,#23753,#23754,#23755,#23756,
#23757,#23758,#23759,#23760,#23761,#23762,#23763),.UNSPECIFIED.,.F.,.F.)
B_SPLINE_CURVE_WITH_KNOTS((6,1,1,1,1,1,1,1,1,1,1,1,1,1,1,1,1,1,1,1,1,1,
1,1,1,1,1,1,1,1,1,1,1,1,1,1,1,1,1,1,1,1,1,1,1,1,1,1,1,1,1,1,1,1,1,1,1,1,
1,1,1,1,1,1,1,6),(0.,0.0153846153846154,0.0307692307692308,0.0461538461538462,
0.0615384615384615,0.0769230769230769,0.0923076923076923,0.107692307692308,
0.123076923076923,0.138461538461538,0.153846153846154,0.169230769230769,
0.184615384615385,0.2,0.215384615384615,0.230769230769231,0.246153846153846,
0.261538461538462,0.276923076923077,0.292307692307692,0.307692307692308,
0.323076923076923,0.338461538461538,0.353846153846154,0.369230769230769,
0.384615384615385,0.4,0.415384615384615,0.430769230769231,0.446153846153846,
0.461538461538462,0.476923076923077,0.492307692307692,0.507692307692308,
0.523076923076923,0.538461538461538,0.553846153846154,0.569230769230769,
0.584615384615384,0.6,0.615384615384615,0.63076923076923,0.646153846153846,
0.661538461538461,0.676923076923076,0.692307692307692,0.707692307692307,
0.723076923076922,0.738461538461538,0.753846153846153,0.769230769230768,
0.784615384615384,0.799999999999999,0.815384615384614,0.83076923076923,
0.846153846153845,0.86153846153846,0.876923076923076,0.892307692307691,
0.907692307692306,0.923076923076922,0.938461538461537,0.953846153846152,
0.969230769230768,0.984615384615383,1.),.UNSPECIFIED.)
CURVE()
GEOMETRIC_REPRESENTATION_ITEM()
RATIONAL_B_SPLINE_CURVE((1.,1.,1.,1.,1.,1.,1.,1.,1.,1.,1.,1.,1.,1.,1.,1.,
1.,1.,1.,1.,1.,1.,1.,1.,1.,1.,1.,1.,1.,1.,1.,1.,1.,1.,1.,1.,1.,1.,1.,1.,
1.,1.,1.,1.,1.,1.,1.,1.,1.,1.,1.,1.,1.,1.,1.,1.,1.,1.,1.,1.,1.,1.,1.,1.,
1.,1.,1.,1.,1.,1.))
REPRESENTATION_ITEM('')
);
#91=(
BOUNDED_CURVE()
B_SPLINE_CURVE(5,(#23917,#23918,#23919,#23920,#23921,#23922,#23923,#23924,
#23925,#23926,#23927,#23928,#23929,#23930,#23931,#23932,#23933,#23934,#23935,
#23936,#23937,#23938,#23939,#23940,#23941,#23942,#23943,#23944,#23945,#23946,
#23947,#23948,#23949,#23950,#23951,#23952,#23953,#23954,#23955,#23956,#23957,
#23958,#23959,#23960,#23961,#23962,#23963,#23964,#23965,#23966,#23967,#23968,
#23969,#23970,#23971,#23972,#23973,#23974,#23975,#23976,#23977,#23978,#23979,
#23980,#23981,#23982,#23983,#23984,#23985,#23986),.UNSPECIFIED.,.F.,.F.)
B_SPLINE_CURVE_WITH_KNOTS((6,1,1,1,1,1,1,1,1,1,1,1,1,1,1,1,1,1,1,1,1,1,
1,1,1,1,1,1,1,1,1,1,1,1,1,1,1,1,1,1,1,1,1,1,1,1,1,1,1,1,1,1,1,1,1,1,1,1,
1,1,1,1,1,1,1,6),(-1.,-0.984615384615383,-0.969230769230768,-0.953846153846152,
-0.938461538461537,-0.923076923076922,-0.907692307692306,-0.892307692307691,
-0.876923076923076,-0.86153846153846,-0.846153846153845,-0.83076923076923,
-0.815384615384614,-0.799999999999999,-0.784615384615384,-0.769230769230768,
-0.753846153846153,-0.738461538461538,-0.723076923076922,-0.707692307692307,
-0.692307692307692,-0.676923076923076,-0.661538461538461,-0.646153846153846,
-0.63076923076923,-0.615384615384615,-0.6,-0.584615384615384,-0.569230769230769,
-0.553846153846154,-0.538461538461538,-0.523076923076923,-0.507692307692308,
-0.492307692307692,-0.476923076923077,-0.461538461538462,-0.446153846153846,
-0.430769230769231,-0.415384615384615,-0.4,-0.384615384615385,-0.369230769230769,
-0.353846153846154,-0.338461538461538,-0.323076923076923,-0.307692307692308,
-0.292307692307692,-0.276923076923077,-0.261538461538462,-0.246153846153846,
-0.230769230769231,-0.215384615384615,-0.2,-0.184615384615385,-0.169230769230769,
-0.153846153846154,-0.138461538461538,-0.123076923076923,-0.107692307692308,
-0.0923076923076923,-0.0769230769230769,-0.0615384615384615,-0.0461538461538462,
-0.0307692307692308,-0.0153846153846154,0.),.UNSPECIFIED.)
CURVE()
GEOMETRIC_REPRESENTATION_ITEM()
RATIONAL_B_SPLINE_CURVE((1.,1.,1.,1.,1.,1.,1.,1.,1.,1.,1.,1.,1.,1.,1.,1.,
1.,1.,1.,1.,1.,1.,1.,1.,1.,1.,1.,1.,1.,1.,1.,1.,1.,1.,1.,1.,1.,1.,1.,1.,
1.,1.,1.,1.,1.,1.,1.,1.,1.,1.,1.,1.,1.,1.,1.,1.,1.,1.,1.,1.,1.,1.,1.,1.,
1.,1.,1.,1.,1.,1.))
REPRESENTATION_ITEM('')
);
#92=(
BOUNDED_CURVE()
B_SPLINE_CURVE(5,(#24133,#24134,#24135,#24136,#24137,#24138,#24139,#24140,
#24141,#24142,#24143,#24144,#24145,#24146,#24147,#24148,#24149,#24150,#24151,
#24152,#24153,#24154,#24155,#24156,#24157,#24158,#24159,#24160,#24161,#24162,
#24163,#24164,#24165,#24166,#24167,#24168,#24169,#24170,#24171,#24172,#24173,
#24174,#24175,#24176,#24177,#24178,#24179,#24180,#24181,#24182,#24183,#24184,
#24185,#24186,#24187,#24188,#24189,#24190,#24191,#24192,#24193,#24194,#24195,
#24196,#24197,#24198,#24199,#24200,#24201,#24202),.UNSPECIFIED.,.F.,.F.)
B_SPLINE_CURVE_WITH_KNOTS((6,1,1,1,1,1,1,1,1,1,1,1,1,1,1,1,1,1,1,1,1,1,
1,1,1,1,1,1,1,1,1,1,1,1,1,1,1,1,1,1,1,1,1,1,1,1,1,1,1,1,1,1,1,1,1,1,1,1,
1,1,1,1,1,1,1,6),(-1.,-0.984615384615383,-0.969230769230768,-0.953846153846152,
-0.938461538461537,-0.923076923076922,-0.907692307692306,-0.892307692307691,
-0.876923076923076,-0.86153846153846,-0.846153846153845,-0.83076923076923,
-0.815384615384614,-0.799999999999999,-0.784615384615384,-0.769230769230768,
-0.753846153846153,-0.738461538461538,-0.723076923076922,-0.707692307692307,
-0.692307692307692,-0.676923076923076,-0.661538461538461,-0.646153846153846,
-0.63076923076923,-0.615384615384615,-0.6,-0.584615384615384,-0.569230769230769,
-0.553846153846154,-0.538461538461538,-0.523076923076923,-0.507692307692308,
-0.492307692307692,-0.476923076923077,-0.461538461538462,-0.446153846153846,
-0.430769230769231,-0.415384615384615,-0.4,-0.384615384615385,-0.369230769230769,
-0.353846153846154,-0.338461538461538,-0.323076923076923,-0.307692307692308,
-0.292307692307692,-0.276923076923077,-0.261538461538462,-0.246153846153846,
-0.230769230769231,-0.215384615384615,-0.2,-0.184615384615385,-0.169230769230769,
-0.153846153846154,-0.138461538461538,-0.123076923076923,-0.107692307692308,
-0.0923076923076923,-0.0769230769230769,-0.0615384615384615,-0.0461538461538462,
-0.0307692307692308,-0.0153846153846154,0.),.UNSPECIFIED.)
CURVE()
GEOMETRIC_REPRESENTATION_ITEM()
RATIONAL_B_SPLINE_CURVE((1.,1.,1.,1.,1.,1.,1.,1.,1.,1.,1.,1.,1.,1.,1.,1.,
1.,1.,1.,1.,1.,1.,1.,1.,1.,1.,1.,1.,1.,1.,1.,1.,1.,1.,1.,1.,1.,1.,1.,1.,
1.,1.,1.,1.,1.,1.,1.,1.,1.,1.,1.,1.,1.,1.,1.,1.,1.,1.,1.,1.,1.,1.,1.,1.,
1.,1.,1.,1.,1.,1.))
REPRESENTATION_ITEM('')
);
#93=(
BOUNDED_CURVE()
B_SPLINE_CURVE(5,(#24349,#24350,#24351,#24352,#24353,#24354,#24355,#24356,
#24357,#24358,#24359,#24360,#24361,#24362,#24363,#24364,#24365,#24366,#24367,
#24368,#24369,#24370,#24371,#24372,#24373,#24374,#24375,#24376,#24377,#24378,
#24379,#24380,#24381,#24382,#24383,#24384,#24385,#24386,#24387,#24388,#24389,
#24390,#24391,#24392,#24393,#24394,#24395,#24396,#24397,#24398,#24399,#24400,
#24401,#24402,#24403,#24404,#24405,#24406,#24407,#24408,#24409,#24410,#24411,
#24412,#24413,#24414,#24415,#24416,#24417,#24418),.UNSPECIFIED.,.F.,.F.)
B_SPLINE_CURVE_WITH_KNOTS((6,1,1,1,1,1,1,1,1,1,1,1,1,1,1,1,1,1,1,1,1,1,
1,1,1,1,1,1,1,1,1,1,1,1,1,1,1,1,1,1,1,1,1,1,1,1,1,1,1,1,1,1,1,1,1,1,1,1,
1,1,1,1,1,1,1,6),(-1.,-0.984615384615383,-0.969230769230768,-0.953846153846152,
-0.938461538461537,-0.923076923076922,-0.907692307692306,-0.892307692307691,
-0.876923076923076,-0.86153846153846,-0.846153846153845,-0.83076923076923,
-0.815384615384614,-0.799999999999999,-0.784615384615384,-0.769230769230768,
-0.753846153846153,-0.738461538461538,-0.723076923076922,-0.707692307692307,
-0.692307692307692,-0.676923076923076,-0.661538461538461,-0.646153846153846,
-0.63076923076923,-0.615384615384615,-0.6,-0.584615384615384,-0.569230769230769,
-0.553846153846154,-0.538461538461538,-0.523076923076923,-0.507692307692308,
-0.492307692307692,-0.476923076923077,-0.461538461538462,-0.446153846153846,
-0.430769230769231,-0.415384615384615,-0.4,-0.384615384615385,-0.369230769230769,
-0.353846153846154,-0.338461538461538,-0.323076923076923,-0.307692307692308,
-0.292307692307692,-0.276923076923077,-0.261538461538462,-0.246153846153846,
-0.230769230769231,-0.215384615384615,-0.2,-0.184615384615385,-0.169230769230769,
-0.153846153846154,-0.138461538461538,-0.123076923076923,-0.107692307692308,
-0.0923076923076923,-0.0769230769230769,-0.0615384615384615,-0.0461538461538462,
-0.0307692307692308,-0.0153846153846154,0.),.UNSPECIFIED.)
CURVE()
GEOMETRIC_REPRESENTATION_ITEM()
RATIONAL_B_SPLINE_CURVE((1.,1.,1.,1.,1.,1.,1.,1.,1.,1.,1.,1.,1.,1.,1.,1.,
1.,1.,1.,1.,1.,1.,1.,1.,1.,1.,1.,1.,1.,1.,1.,1.,1.,1.,1.,1.,1.,1.,1.,1.,
1.,1.,1.,1.,1.,1.,1.,1.,1.,1.,1.,1.,1.,1.,1.,1.,1.,1.,1.,1.,1.,1.,1.,1.,
1.,1.,1.,1.,1.,1.))
REPRESENTATION_ITEM('')
);
#94=(
BOUNDED_CURVE()
B_SPLINE_CURVE(5,(#24565,#24566,#24567,#24568,#24569,#24570,#24571,#24572,
#24573,#24574,#24575,#24576,#24577,#24578,#24579,#24580,#24581,#24582,#24583,
#24584,#24585,#24586,#24587,#24588,#24589,#24590,#24591,#24592,#24593,#24594,
#24595,#24596,#24597,#24598,#24599,#24600,#24601,#24602,#24603,#24604,#24605,
#24606,#24607,#24608,#24609,#24610,#24611,#24612,#24613,#24614,#24615,#24616,
#24617,#24618,#24619,#24620,#24621,#24622,#24623,#24624,#24625,#24626,#24627,
#24628,#24629,#24630,#24631,#24632,#24633,#24634),.UNSPECIFIED.,.F.,.F.)
B_SPLINE_CURVE_WITH_KNOTS((6,1,1,1,1,1,1,1,1,1,1,1,1,1,1,1,1,1,1,1,1,1,
1,1,1,1,1,1,1,1,1,1,1,1,1,1,1,1,1,1,1,1,1,1,1,1,1,1,1,1,1,1,1,1,1,1,1,1,
1,1,1,1,1,1,1,6),(-1.,-0.984615384615383,-0.969230769230768,-0.953846153846152,
-0.938461538461537,-0.923076923076922,-0.907692307692306,-0.892307692307691,
-0.876923076923076,-0.86153846153846,-0.846153846153845,-0.83076923076923,
-0.815384615384614,-0.799999999999999,-0.784615384615384,-0.769230769230768,
-0.753846153846153,-0.738461538461538,-0.723076923076922,-0.707692307692307,
-0.692307692307692,-0.676923076923076,-0.661538461538461,-0.646153846153846,
-0.63076923076923,-0.615384615384615,-0.6,-0.584615384615384,-0.569230769230769,
-0.553846153846154,-0.538461538461538,-0.523076923076923,-0.507692307692308,
-0.492307692307692,-0.476923076923077,-0.461538461538462,-0.446153846153846,
-0.430769230769231,-0.415384615384615,-0.4,-0.384615384615385,-0.369230769230769,
-0.353846153846154,-0.338461538461538,-0.323076923076923,-0.307692307692308,
-0.292307692307692,-0.276923076923077,-0.261538461538462,-0.246153846153846,
-0.230769230769231,-0.215384615384615,-0.2,-0.184615384615385,-0.169230769230769,
-0.153846153846154,-0.138461538461538,-0.123076923076923,-0.107692307692308,
-0.0923076923076923,-0.0769230769230769,-0.0615384615384615,-0.0461538461538462,
-0.0307692307692308,-0.0153846153846154,0.),.UNSPECIFIED.)
CURVE()
GEOMETRIC_REPRESENTATION_ITEM()
RATIONAL_B_SPLINE_CURVE((1.,1.,1.,1.,1.,1.,1.,1.,1.,1.,1.,1.,1.,1.,1.,1.,
1.,1.,1.,1.,1.,1.,1.,1.,1.,1.,1.,1.,1.,1.,1.,1.,1.,1.,1.,1.,1.,1.,1.,1.,
1.,1.,1.,1.,1.,1.,1.,1.,1.,1.,1.,1.,1.,1.,1.,1.,1.,1.,1.,1.,1.,1.,1.,1.,
1.,1.,1.,1.,1.,1.))
REPRESENTATION_ITEM('')
);
#95=(
BOUNDED_CURVE()
B_SPLINE_CURVE(5,(#24781,#24782,#24783,#24784,#24785,#24786,#24787,#24788,
#24789,#24790,#24791,#24792,#24793,#24794,#24795,#24796,#24797,#24798,#24799,
#24800,#24801,#24802,#24803,#24804,#24805,#24806,#24807,#24808,#24809,#24810,
#24811,#24812,#24813,#24814,#24815,#24816,#24817,#24818,#24819,#24820,#24821,
#24822,#24823,#24824,#24825,#24826,#24827,#24828,#24829,#24830,#24831,#24832,
#24833,#24834,#24835,#24836,#24837,#24838,#24839,#24840,#24841,#24842,#24843,
#24844,#24845,#24846,#24847,#24848,#24849,#24850),.UNSPECIFIED.,.F.,.F.)
B_SPLINE_CURVE_WITH_KNOTS((6,1,1,1,1,1,1,1,1,1,1,1,1,1,1,1,1,1,1,1,1,1,
1,1,1,1,1,1,1,1,1,1,1,1,1,1,1,1,1,1,1,1,1,1,1,1,1,1,1,1,1,1,1,1,1,1,1,1,
1,1,1,1,1,1,1,6),(-1.,-0.984615384615383,-0.969230769230768,-0.953846153846152,
-0.938461538461537,-0.923076923076922,-0.907692307692306,-0.892307692307691,
-0.876923076923076,-0.86153846153846,-0.846153846153845,-0.83076923076923,
-0.815384615384614,-0.799999999999999,-0.784615384615384,-0.769230769230768,
-0.753846153846153,-0.738461538461538,-0.723076923076922,-0.707692307692307,
-0.692307692307692,-0.676923076923076,-0.661538461538461,-0.646153846153846,
-0.63076923076923,-0.615384615384615,-0.6,-0.584615384615384,-0.569230769230769,
-0.553846153846154,-0.538461538461538,-0.523076923076923,-0.507692307692308,
-0.492307692307692,-0.476923076923077,-0.461538461538462,-0.446153846153846,
-0.430769230769231,-0.415384615384615,-0.4,-0.384615384615385,-0.369230769230769,
-0.353846153846154,-0.338461538461538,-0.323076923076923,-0.307692307692308,
-0.292307692307692,-0.276923076923077,-0.261538461538462,-0.246153846153846,
-0.230769230769231,-0.215384615384615,-0.2,-0.184615384615385,-0.169230769230769,
-0.153846153846154,-0.138461538461538,-0.123076923076923,-0.107692307692308,
-0.0923076923076923,-0.0769230769230769,-0.0615384615384615,-0.0461538461538462,
-0.0307692307692308,-0.0153846153846154,0.),.UNSPECIFIED.)
CURVE()
GEOMETRIC_REPRESENTATION_ITEM()
RATIONAL_B_SPLINE_CURVE((1.,1.,1.,1.,1.,1.,1.,1.,1.,1.,1.,1.,1.,1.,1.,1.,
1.,1.,1.,1.,1.,1.,1.,1.,1.,1.,1.,1.,1.,1.,1.,1.,1.,1.,1.,1.,1.,1.,1.,1.,
1.,1.,1.,1.,1.,1.,1.,1.,1.,1.,1.,1.,1.,1.,1.,1.,1.,1.,1.,1.,1.,1.,1.,1.,
1.,1.,1.,1.,1.,1.))
REPRESENTATION_ITEM('')
);
#96=(
BOUNDED_CURVE()
B_SPLINE_CURVE(5,(#24997,#24998,#24999,#25000,#25001,#25002,#25003,#25004,
#25005,#25006,#25007,#25008,#25009,#25010,#25011,#25012,#25013,#25014,#25015,
#25016,#25017,#25018,#25019,#25020,#25021,#25022,#25023,#25024,#25025,#25026,
#25027,#25028,#25029,#25030,#25031,#25032,#25033,#25034,#25035,#25036,#25037,
#25038,#25039,#25040,#25041,#25042,#25043,#25044,#25045,#25046,#25047,#25048,
#25049,#25050,#25051,#25052,#25053,#25054,#25055,#25056,#25057,#25058,#25059,
#25060,#25061,#25062,#25063,#25064,#25065,#25066),.UNSPECIFIED.,.F.,.F.)
B_SPLINE_CURVE_WITH_KNOTS((6,1,1,1,1,1,1,1,1,1,1,1,1,1,1,1,1,1,1,1,1,1,
1,1,1,1,1,1,1,1,1,1,1,1,1,1,1,1,1,1,1,1,1,1,1,1,1,1,1,1,1,1,1,1,1,1,1,1,
1,1,1,1,1,1,1,6),(-1.,-0.984615384615383,-0.969230769230768,-0.953846153846152,
-0.938461538461537,-0.923076923076922,-0.907692307692306,-0.892307692307691,
-0.876923076923076,-0.86153846153846,-0.846153846153845,-0.83076923076923,
-0.815384615384614,-0.799999999999999,-0.784615384615384,-0.769230769230768,
-0.753846153846153,-0.738461538461538,-0.723076923076922,-0.707692307692307,
-0.692307692307692,-0.676923076923076,-0.661538461538461,-0.646153846153846,
-0.63076923076923,-0.615384615384615,-0.6,-0.584615384615384,-0.569230769230769,
-0.553846153846154,-0.538461538461538,-0.523076923076923,-0.507692307692308,
-0.492307692307692,-0.476923076923077,-0.461538461538462,-0.446153846153846,
-0.430769230769231,-0.415384615384615,-0.4,-0.384615384615385,-0.369230769230769,
-0.353846153846154,-0.338461538461538,-0.323076923076923,-0.307692307692308,
-0.292307692307692,-0.276923076923077,-0.261538461538462,-0.246153846153846,
-0.230769230769231,-0.215384615384615,-0.2,-0.184615384615385,-0.169230769230769,
-0.153846153846154,-0.138461538461538,-0.123076923076923,-0.107692307692308,
-0.0923076923076923,-0.0769230769230769,-0.0615384615384615,-0.0461538461538462,
-0.0307692307692308,-0.0153846153846154,0.),.UNSPECIFIED.)
CURVE()
GEOMETRIC_REPRESENTATION_ITEM()
RATIONAL_B_SPLINE_CURVE((1.,1.,1.,1.,1.,1.,1.,1.,1.,1.,1.,1.,1.,1.,1.,1.,
1.,1.,1.,1.,1.,1.,1.,1.,1.,1.,1.,1.,1.,1.,1.,1.,1.,1.,1.,1.,1.,1.,1.,1.,
1.,1.,1.,1.,1.,1.,1.,1.,1.,1.,1.,1.,1.,1.,1.,1.,1.,1.,1.,1.,1.,1.,1.,1.,
1.,1.,1.,1.,1.,1.))
REPRESENTATION_ITEM('')
);
#97=(
BOUNDED_CURVE()
B_SPLINE_CURVE(5,(#25213,#25214,#25215,#25216,#25217,#25218,#25219,#25220,
#25221,#25222,#25223,#25224,#25225,#25226,#25227,#25228,#25229,#25230,#25231,
#25232,#25233,#25234,#25235,#25236,#25237,#25238,#25239,#25240,#25241,#25242,
#25243,#25244,#25245,#25246,#25247,#25248,#25249,#25250,#25251,#25252,#25253,
#25254,#25255,#25256,#25257,#25258,#25259,#25260,#25261,#25262,#25263,#25264,
#25265,#25266,#25267,#25268,#25269,#25270,#25271,#25272,#25273,#25274,#25275,
#25276,#25277,#25278,#25279,#25280,#25281,#25282),.UNSPECIFIED.,.F.,.F.)
B_SPLINE_CURVE_WITH_KNOTS((6,1,1,1,1,1,1,1,1,1,1,1,1,1,1,1,1,1,1,1,1,1,
1,1,1,1,1,1,1,1,1,1,1,1,1,1,1,1,1,1,1,1,1,1,1,1,1,1,1,1,1,1,1,1,1,1,1,1,
1,1,1,1,1,1,1,6),(-1.,-0.984615384615383,-0.969230769230768,-0.953846153846152,
-0.938461538461537,-0.923076923076922,-0.907692307692306,-0.892307692307691,
-0.876923076923076,-0.86153846153846,-0.846153846153845,-0.83076923076923,
-0.815384615384614,-0.799999999999999,-0.784615384615384,-0.769230769230768,
-0.753846153846153,-0.738461538461538,-0.723076923076922,-0.707692307692307,
-0.692307692307692,-0.676923076923076,-0.661538461538461,-0.646153846153846,
-0.63076923076923,-0.615384615384615,-0.6,-0.584615384615384,-0.569230769230769,
-0.553846153846154,-0.538461538461538,-0.523076923076923,-0.507692307692308,
-0.492307692307692,-0.476923076923077,-0.461538461538462,-0.446153846153846,
-0.430769230769231,-0.415384615384615,-0.4,-0.384615384615385,-0.369230769230769,
-0.353846153846154,-0.338461538461538,-0.323076923076923,-0.307692307692308,
-0.292307692307692,-0.276923076923077,-0.261538461538462,-0.246153846153846,
-0.230769230769231,-0.215384615384615,-0.2,-0.184615384615385,-0.169230769230769,
-0.153846153846154,-0.138461538461538,-0.123076923076923,-0.107692307692308,
-0.0923076923076923,-0.0769230769230769,-0.0615384615384615,-0.0461538461538462,
-0.0307692307692308,-0.0153846153846154,0.),.UNSPECIFIED.)
CURVE()
GEOMETRIC_REPRESENTATION_ITEM()
RATIONAL_B_SPLINE_CURVE((1.,1.,1.,1.,1.,1.,1.,1.,1.,1.,1.,1.,1.,1.,1.,1.,
1.,1.,1.,1.,1.,1.,1.,1.,1.,1.,1.,1.,1.,1.,1.,1.,1.,1.,1.,1.,1.,1.,1.,1.,
1.,1.,1.,1.,1.,1.,1.,1.,1.,1.,1.,1.,1.,1.,1.,1.,1.,1.,1.,1.,1.,1.,1.,1.,
1.,1.,1.,1.,1.,1.))
REPRESENTATION_ITEM('')
);
#98=(
BOUNDED_CURVE()
B_SPLINE_CURVE(5,(#25429,#25430,#25431,#25432,#25433,#25434,#25435,#25436,
#25437,#25438,#25439,#25440,#25441,#25442,#25443,#25444,#25445,#25446,#25447,
#25448,#25449,#25450,#25451,#25452,#25453,#25454,#25455,#25456,#25457,#25458,
#25459,#25460,#25461,#25462,#25463,#25464,#25465,#25466,#25467,#25468,#25469,
#25470,#25471,#25472,#25473,#25474,#25475,#25476,#25477,#25478,#25479,#25480,
#25481,#25482,#25483,#25484,#25485,#25486,#25487,#25488,#25489,#25490,#25491,
#25492,#25493,#25494,#25495,#25496,#25497,#25498),.UNSPECIFIED.,.F.,.F.)
B_SPLINE_CURVE_WITH_KNOTS((6,1,1,1,1,1,1,1,1,1,1,1,1,1,1,1,1,1,1,1,1,1,
1,1,1,1,1,1,1,1,1,1,1,1,1,1,1,1,1,1,1,1,1,1,1,1,1,1,1,1,1,1,1,1,1,1,1,1,
1,1,1,1,1,1,1,6),(-1.,-0.984615384615383,-0.969230769230768,-0.953846153846152,
-0.938461538461537,-0.923076923076922,-0.907692307692306,-0.892307692307691,
-0.876923076923076,-0.86153846153846,-0.846153846153845,-0.83076923076923,
-0.815384615384614,-0.799999999999999,-0.784615384615384,-0.769230769230768,
-0.753846153846153,-0.738461538461538,-0.723076923076922,-0.707692307692307,
-0.692307692307692,-0.676923076923076,-0.661538461538461,-0.646153846153846,
-0.63076923076923,-0.615384615384615,-0.6,-0.584615384615384,-0.569230769230769,
-0.553846153846154,-0.538461538461538,-0.523076923076923,-0.507692307692308,
-0.492307692307692,-0.476923076923077,-0.461538461538462,-0.446153846153846,
-0.430769230769231,-0.415384615384615,-0.4,-0.384615384615385,-0.369230769230769,
-0.353846153846154,-0.338461538461538,-0.323076923076923,-0.307692307692308,
-0.292307692307692,-0.276923076923077,-0.261538461538462,-0.246153846153846,
-0.230769230769231,-0.215384615384615,-0.2,-0.184615384615385,-0.169230769230769,
-0.153846153846154,-0.138461538461538,-0.123076923076923,-0.107692307692308,
-0.0923076923076923,-0.0769230769230769,-0.0615384615384615,-0.0461538461538462,
-0.0307692307692308,-0.0153846153846154,0.),.UNSPECIFIED.)
CURVE()
GEOMETRIC_REPRESENTATION_ITEM()
RATIONAL_B_SPLINE_CURVE((1.,1.,1.,1.,1.,1.,1.,1.,1.,1.,1.,1.,1.,1.,1.,1.,
1.,1.,1.,1.,1.,1.,1.,1.,1.,1.,1.,1.,1.,1.,1.,1.,1.,1.,1.,1.,1.,1.,1.,1.,
1.,1.,1.,1.,1.,1.,1.,1.,1.,1.,1.,1.,1.,1.,1.,1.,1.,1.,1.,1.,1.,1.,1.,1.,
1.,1.,1.,1.,1.,1.))
REPRESENTATION_ITEM('')
);
#99=(
BOUNDED_CURVE()
B_SPLINE_CURVE(5,(#25645,#25646,#25647,#25648,#25649,#25650,#25651,#25652,
#25653,#25654,#25655,#25656,#25657,#25658,#25659,#25660,#25661,#25662,#25663,
#25664,#25665,#25666,#25667,#25668,#25669,#25670,#25671,#25672,#25673,#25674,
#25675,#25676,#25677,#25678,#25679,#25680,#25681,#25682,#25683,#25684,#25685,
#25686,#25687,#25688,#25689,#25690,#25691,#25692,#25693,#25694,#25695,#25696,
#25697,#25698,#25699,#25700,#25701,#25702,#25703,#25704,#25705,#25706,#25707,
#25708,#25709,#25710,#25711,#25712,#25713,#25714),.UNSPECIFIED.,.F.,.F.)
B_SPLINE_CURVE_WITH_KNOTS((6,1,1,1,1,1,1,1,1,1,1,1,1,1,1,1,1,1,1,1,1,1,
1,1,1,1,1,1,1,1,1,1,1,1,1,1,1,1,1,1,1,1,1,1,1,1,1,1,1,1,1,1,1,1,1,1,1,1,
1,1,1,1,1,1,1,6),(-1.,-0.984615384615383,-0.969230769230768,-0.953846153846152,
-0.938461538461537,-0.923076923076922,-0.907692307692306,-0.892307692307691,
-0.876923076923076,-0.86153846153846,-0.846153846153845,-0.83076923076923,
-0.815384615384614,-0.799999999999999,-0.784615384615384,-0.769230769230768,
-0.753846153846153,-0.738461538461538,-0.723076923076922,-0.707692307692307,
-0.692307692307692,-0.676923076923076,-0.661538461538461,-0.646153846153846,
-0.63076923076923,-0.615384615384615,-0.6,-0.584615384615384,-0.569230769230769,
-0.553846153846154,-0.538461538461538,-0.523076923076923,-0.507692307692308,
-0.492307692307692,-0.476923076923077,-0.461538461538462,-0.446153846153846,
-0.430769230769231,-0.415384615384615,-0.4,-0.384615384615385,-0.369230769230769,
-0.353846153846154,-0.338461538461538,-0.323076923076923,-0.307692307692308,
-0.292307692307692,-0.276923076923077,-0.261538461538462,-0.246153846153846,
-0.230769230769231,-0.215384615384615,-0.2,-0.184615384615385,-0.169230769230769,
-0.153846153846154,-0.138461538461538,-0.123076923076923,-0.107692307692308,
-0.0923076923076923,-0.0769230769230769,-0.0615384615384615,-0.0461538461538462,
-0.0307692307692308,-0.0153846153846154,0.),.UNSPECIFIED.)
CURVE()
GEOMETRIC_REPRESENTATION_ITEM()
RATIONAL_B_SPLINE_CURVE((1.,1.,1.,1.,1.,1.,1.,1.,1.,1.,1.,1.,1.,1.,1.,1.,
1.,1.,1.,1.,1.,1.,1.,1.,1.,1.,1.,1.,1.,1.,1.,1.,1.,1.,1.,1.,1.,1.,1.,1.,
1.,1.,1.,1.,1.,1.,1.,1.,1.,1.,1.,1.,1.,1.,1.,1.,1.,1.,1.,1.,1.,1.,1.,1.,
1.,1.,1.,1.,1.,1.))
REPRESENTATION_ITEM('')
);
#100=(
BOUNDED_CURVE()
B_SPLINE_CURVE(5,(#25861,#25862,#25863,#25864,#25865,#25866,#25867,#25868,
#25869,#25870,#25871,#25872,#25873,#25874,#25875,#25876,#25877,#25878,#25879,
#25880,#25881,#25882,#25883,#25884,#25885,#25886,#25887,#25888,#25889,#25890,
#25891,#25892,#25893,#25894,#25895,#25896,#25897,#25898,#25899,#25900,#25901,
#25902,#25903,#25904,#25905,#25906,#25907,#25908,#25909,#25910,#25911,#25912,
#25913,#25914,#25915,#25916,#25917,#25918,#25919,#25920,#25921,#25922,#25923,
#25924,#25925,#25926,#25927,#25928,#25929,#25930),.UNSPECIFIED.,.F.,.F.)
B_SPLINE_CURVE_WITH_KNOTS((6,1,1,1,1,1,1,1,1,1,1,1,1,1,1,1,1,1,1,1,1,1,
1,1,1,1,1,1,1,1,1,1,1,1,1,1,1,1,1,1,1,1,1,1,1,1,1,1,1,1,1,1,1,1,1,1,1,1,
1,1,1,1,1,1,1,6),(-1.,-0.984615384615383,-0.969230769230768,-0.953846153846152,
-0.938461538461537,-0.923076923076922,-0.907692307692306,-0.892307692307691,
-0.876923076923076,-0.86153846153846,-0.846153846153845,-0.83076923076923,
-0.815384615384614,-0.799999999999999,-0.784615384615384,-0.769230769230768,
-0.753846153846153,-0.738461538461538,-0.723076923076922,-0.707692307692307,
-0.692307692307692,-0.676923076923076,-0.661538461538461,-0.646153846153846,
-0.63076923076923,-0.615384615384615,-0.6,-0.584615384615384,-0.569230769230769,
-0.553846153846154,-0.538461538461538,-0.523076923076923,-0.507692307692308,
-0.492307692307692,-0.476923076923077,-0.461538461538462,-0.446153846153846,
-0.430769230769231,-0.415384615384615,-0.4,-0.384615384615385,-0.369230769230769,
-0.353846153846154,-0.338461538461538,-0.323076923076923,-0.307692307692308,
-0.292307692307692,-0.276923076923077,-0.261538461538462,-0.246153846153846,
-0.230769230769231,-0.215384615384615,-0.2,-0.184615384615385,-0.169230769230769,
-0.153846153846154,-0.138461538461538,-0.123076923076923,-0.107692307692308,
-0.0923076923076923,-0.0769230769230769,-0.0615384615384615,-0.0461538461538462,
-0.0307692307692308,-0.0153846153846154,0.),.UNSPECIFIED.)
CURVE()
GEOMETRIC_REPRESENTATION_ITEM()
RATIONAL_B_SPLINE_CURVE((1.,1.,1.,1.,1.,1.,1.,1.,1.,1.,1.,1.,1.,1.,1.,1.,
1.,1.,1.,1.,1.,1.,1.,1.,1.,1.,1.,1.,1.,1.,1.,1.,1.,1.,1.,1.,1.,1.,1.,1.,
1.,1.,1.,1.,1.,1.,1.,1.,1.,1.,1.,1.,1.,1.,1.,1.,1.,1.,1.,1.,1.,1.,1.,1.,
1.,1.,1.,1.,1.,1.))
REPRESENTATION_ITEM('')
);
#101=(
BOUNDED_CURVE()
B_SPLINE_CURVE(5,(#26077,#26078,#26079,#26080,#26081,#26082,#26083,#26084,
#26085,#26086,#26087,#26088,#26089,#26090,#26091,#26092,#26093,#26094,#26095,
#26096,#26097,#26098,#26099,#26100,#26101,#26102,#26103,#26104,#26105,#26106,
#26107,#26108,#26109,#26110,#26111,#26112,#26113,#26114,#26115,#26116,#26117,
#26118,#26119,#26120,#26121,#26122,#26123,#26124,#26125,#26126,#26127,#26128,
#26129,#26130,#26131,#26132,#26133,#26134,#26135,#26136,#26137,#26138,#26139,
#26140,#26141,#26142,#26143,#26144,#26145,#26146),.UNSPECIFIED.,.F.,.F.)
B_SPLINE_CURVE_WITH_KNOTS((6,1,1,1,1,1,1,1,1,1,1,1,1,1,1,1,1,1,1,1,1,1,
1,1,1,1,1,1,1,1,1,1,1,1,1,1,1,1,1,1,1,1,1,1,1,1,1,1,1,1,1,1,1,1,1,1,1,1,
1,1,1,1,1,1,1,6),(-1.,-0.984615384615383,-0.969230769230768,-0.953846153846152,
-0.938461538461537,-0.923076923076922,-0.907692307692306,-0.892307692307691,
-0.876923076923076,-0.86153846153846,-0.846153846153845,-0.83076923076923,
-0.815384615384614,-0.799999999999999,-0.784615384615384,-0.769230769230768,
-0.753846153846153,-0.738461538461538,-0.723076923076922,-0.707692307692307,
-0.692307692307692,-0.676923076923076,-0.661538461538461,-0.646153846153846,
-0.63076923076923,-0.615384615384615,-0.6,-0.584615384615384,-0.569230769230769,
-0.553846153846154,-0.538461538461538,-0.523076923076923,-0.507692307692308,
-0.492307692307692,-0.476923076923077,-0.461538461538462,-0.446153846153846,
-0.430769230769231,-0.415384615384615,-0.4,-0.384615384615385,-0.369230769230769,
-0.353846153846154,-0.338461538461538,-0.323076923076923,-0.307692307692308,
-0.292307692307692,-0.276923076923077,-0.261538461538462,-0.246153846153846,
-0.230769230769231,-0.215384615384615,-0.2,-0.184615384615385,-0.169230769230769,
-0.153846153846154,-0.138461538461538,-0.123076923076923,-0.107692307692308,
-0.0923076923076923,-0.0769230769230769,-0.0615384615384615,-0.0461538461538462,
-0.0307692307692308,-0.0153846153846154,0.),.UNSPECIFIED.)
CURVE()
GEOMETRIC_REPRESENTATION_ITEM()
RATIONAL_B_SPLINE_CURVE((1.,1.,1.,1.,1.,1.,1.,1.,1.,1.,1.,1.,1.,1.,1.,1.,
1.,1.,1.,1.,1.,1.,1.,1.,1.,1.,1.,1.,1.,1.,1.,1.,1.,1.,1.,1.,1.,1.,1.,1.,
1.,1.,1.,1.,1.,1.,1.,1.,1.,1.,1.,1.,1.,1.,1.,1.,1.,1.,1.,1.,1.,1.,1.,1.,
1.,1.,1.,1.,1.,1.))
REPRESENTATION_ITEM('')
);
#102=(
BOUNDED_CURVE()
B_SPLINE_CURVE(5,(#26293,#26294,#26295,#26296,#26297,#26298,#26299,#26300,
#26301,#26302,#26303,#26304,#26305,#26306,#26307,#26308,#26309,#26310,#26311,
#26312,#26313,#26314,#26315,#26316,#26317,#26318,#26319,#26320,#26321,#26322,
#26323,#26324,#26325,#26326,#26327,#26328,#26329,#26330,#26331,#26332,#26333,
#26334,#26335,#26336,#26337,#26338,#26339,#26340,#26341,#26342,#26343,#26344,
#26345,#26346,#26347,#26348,#26349,#26350,#26351,#26352,#26353,#26354,#26355,
#26356,#26357,#26358,#26359,#26360,#26361,#26362),.UNSPECIFIED.,.F.,.F.)
B_SPLINE_CURVE_WITH_KNOTS((6,1,1,1,1,1,1,1,1,1,1,1,1,1,1,1,1,1,1,1,1,1,
1,1,1,1,1,1,1,1,1,1,1,1,1,1,1,1,1,1,1,1,1,1,1,1,1,1,1,1,1,1,1,1,1,1,1,1,
1,1,1,1,1,1,1,6),(-1.,-0.984615384615383,-0.969230769230768,-0.953846153846152,
-0.938461538461537,-0.923076923076922,-0.907692307692306,-0.892307692307691,
-0.876923076923076,-0.86153846153846,-0.846153846153845,-0.83076923076923,
-0.815384615384614,-0.799999999999999,-0.784615384615384,-0.769230769230768,
-0.753846153846153,-0.738461538461538,-0.723076923076922,-0.707692307692307,
-0.692307692307692,-0.676923076923076,-0.661538461538461,-0.646153846153846,
-0.63076923076923,-0.615384615384615,-0.6,-0.584615384615384,-0.569230769230769,
-0.553846153846154,-0.538461538461538,-0.523076923076923,-0.507692307692308,
-0.492307692307692,-0.476923076923077,-0.461538461538462,-0.446153846153846,
-0.430769230769231,-0.415384615384615,-0.4,-0.384615384615385,-0.369230769230769,
-0.353846153846154,-0.338461538461538,-0.323076923076923,-0.307692307692308,
-0.292307692307692,-0.276923076923077,-0.261538461538462,-0.246153846153846,
-0.230769230769231,-0.215384615384615,-0.2,-0.184615384615385,-0.169230769230769,
-0.153846153846154,-0.138461538461538,-0.123076923076923,-0.107692307692308,
-0.0923076923076923,-0.0769230769230769,-0.0615384615384615,-0.0461538461538462,
-0.0307692307692308,-0.0153846153846154,0.),.UNSPECIFIED.)
CURVE()
GEOMETRIC_REPRESENTATION_ITEM()
RATIONAL_B_SPLINE_CURVE((1.,1.,1.,1.,1.,1.,1.,1.,1.,1.,1.,1.,1.,1.,1.,1.,
1.,1.,1.,1.,1.,1.,1.,1.,1.,1.,1.,1.,1.,1.,1.,1.,1.,1.,1.,1.,1.,1.,1.,1.,
1.,1.,1.,1.,1.,1.,1.,1.,1.,1.,1.,1.,1.,1.,1.,1.,1.,1.,1.,1.,1.,1.,1.,1.,
1.,1.,1.,1.,1.,1.))
REPRESENTATION_ITEM('')
);
#103=(
BOUNDED_CURVE()
B_SPLINE_CURVE(5,(#26509,#26510,#26511,#26512,#26513,#26514,#26515,#26516,
#26517,#26518,#26519,#26520,#26521,#26522,#26523,#26524,#26525,#26526,#26527,
#26528,#26529,#26530,#26531,#26532,#26533,#26534,#26535,#26536,#26537,#26538,
#26539,#26540,#26541,#26542,#26543,#26544,#26545,#26546,#26547,#26548,#26549,
#26550,#26551,#26552,#26553,#26554,#26555,#26556,#26557,#26558,#26559,#26560,
#26561,#26562,#26563,#26564,#26565,#26566,#26567,#26568,#26569,#26570,#26571,
#26572,#26573,#26574,#26575,#26576,#26577,#26578),.UNSPECIFIED.,.F.,.F.)
B_SPLINE_CURVE_WITH_KNOTS((6,1,1,1,1,1,1,1,1,1,1,1,1,1,1,1,1,1,1,1,1,1,
1,1,1,1,1,1,1,1,1,1,1,1,1,1,1,1,1,1,1,1,1,1,1,1,1,1,1,1,1,1,1,1,1,1,1,1,
1,1,1,1,1,1,1,6),(-1.,-0.984615384615383,-0.969230769230768,-0.953846153846152,
-0.938461538461537,-0.923076923076922,-0.907692307692306,-0.892307692307691,
-0.876923076923076,-0.86153846153846,-0.846153846153845,-0.83076923076923,
-0.815384615384614,-0.799999999999999,-0.784615384615384,-0.769230769230768,
-0.753846153846153,-0.738461538461538,-0.723076923076922,-0.707692307692307,
-0.692307692307692,-0.676923076923076,-0.661538461538461,-0.646153846153846,
-0.63076923076923,-0.615384615384615,-0.6,-0.584615384615384,-0.569230769230769,
-0.553846153846154,-0.538461538461538,-0.523076923076923,-0.507692307692308,
-0.492307692307692,-0.476923076923077,-0.461538461538462,-0.446153846153846,
-0.430769230769231,-0.415384615384615,-0.4,-0.384615384615385,-0.369230769230769,
-0.353846153846154,-0.338461538461538,-0.323076923076923,-0.307692307692308,
-0.292307692307692,-0.276923076923077,-0.261538461538462,-0.246153846153846,
-0.230769230769231,-0.215384615384615,-0.2,-0.184615384615385,-0.169230769230769,
-0.153846153846154,-0.138461538461538,-0.123076923076923,-0.107692307692308,
-0.0923076923076923,-0.0769230769230769,-0.0615384615384615,-0.0461538461538462,
-0.0307692307692308,-0.0153846153846154,0.),.UNSPECIFIED.)
CURVE()
GEOMETRIC_REPRESENTATION_ITEM()
RATIONAL_B_SPLINE_CURVE((1.,1.,1.,1.,1.,1.,1.,1.,1.,1.,1.,1.,1.,1.,1.,1.,
1.,1.,1.,1.,1.,1.,1.,1.,1.,1.,1.,1.,1.,1.,1.,1.,1.,1.,1.,1.,1.,1.,1.,1.,
1.,1.,1.,1.,1.,1.,1.,1.,1.,1.,1.,1.,1.,1.,1.,1.,1.,1.,1.,1.,1.,1.,1.,1.,
1.,1.,1.,1.,1.,1.))
REPRESENTATION_ITEM('')
);
#104=(
BOUNDED_CURVE()
B_SPLINE_CURVE(5,(#26725,#26726,#26727,#26728,#26729,#26730,#26731,#26732,
#26733,#26734,#26735,#26736,#26737,#26738,#26739,#26740,#26741,#26742,#26743,
#26744,#26745,#26746,#26747,#26748,#26749,#26750,#26751,#26752,#26753,#26754,
#26755,#26756,#26757,#26758,#26759,#26760,#26761,#26762,#26763,#26764,#26765,
#26766,#26767,#26768,#26769,#26770,#26771,#26772,#26773,#26774,#26775,#26776,
#26777,#26778,#26779,#26780,#26781,#26782,#26783,#26784,#26785,#26786,#26787,
#26788,#26789,#26790,#26791,#26792,#26793,#26794),.UNSPECIFIED.,.F.,.F.)
B_SPLINE_CURVE_WITH_KNOTS((6,1,1,1,1,1,1,1,1,1,1,1,1,1,1,1,1,1,1,1,1,1,
1,1,1,1,1,1,1,1,1,1,1,1,1,1,1,1,1,1,1,1,1,1,1,1,1,1,1,1,1,1,1,1,1,1,1,1,
1,1,1,1,1,1,1,6),(-1.,-0.984615384615383,-0.969230769230768,-0.953846153846152,
-0.938461538461537,-0.923076923076922,-0.907692307692306,-0.892307692307691,
-0.876923076923076,-0.86153846153846,-0.846153846153845,-0.83076923076923,
-0.815384615384614,-0.799999999999999,-0.784615384615384,-0.769230769230768,
-0.753846153846153,-0.738461538461538,-0.723076923076922,-0.707692307692307,
-0.692307692307692,-0.676923076923076,-0.661538461538461,-0.646153846153846,
-0.63076923076923,-0.615384615384615,-0.6,-0.584615384615384,-0.569230769230769,
-0.553846153846154,-0.538461538461538,-0.523076923076923,-0.507692307692308,
-0.492307692307692,-0.476923076923077,-0.461538461538462,-0.446153846153846,
-0.430769230769231,-0.415384615384615,-0.4,-0.384615384615385,-0.369230769230769,
-0.353846153846154,-0.338461538461538,-0.323076923076923,-0.307692307692308,
-0.292307692307692,-0.276923076923077,-0.261538461538462,-0.246153846153846,
-0.230769230769231,-0.215384615384615,-0.2,-0.184615384615385,-0.169230769230769,
-0.153846153846154,-0.138461538461538,-0.123076923076923,-0.107692307692308,
-0.0923076923076923,-0.0769230769230769,-0.0615384615384615,-0.0461538461538462,
-0.0307692307692308,-0.0153846153846154,0.),.UNSPECIFIED.)
CURVE()
GEOMETRIC_REPRESENTATION_ITEM()
RATIONAL_B_SPLINE_CURVE((1.,1.,1.,1.,1.,1.,1.,1.,1.,1.,1.,1.,1.,1.,1.,1.,
1.,1.,1.,1.,1.,1.,1.,1.,1.,1.,1.,1.,1.,1.,1.,1.,1.,1.,1.,1.,1.,1.,1.,1.,
1.,1.,1.,1.,1.,1.,1.,1.,1.,1.,1.,1.,1.,1.,1.,1.,1.,1.,1.,1.,1.,1.,1.,1.,
1.,1.,1.,1.,1.,1.))
REPRESENTATION_ITEM('')
);
#105=(
BOUNDED_CURVE()
B_SPLINE_CURVE(5,(#26941,#26942,#26943,#26944,#26945,#26946,#26947,#26948,
#26949,#26950,#26951,#26952,#26953,#26954,#26955,#26956,#26957,#26958,#26959,
#26960,#26961,#26962,#26963,#26964,#26965,#26966,#26967,#26968,#26969,#26970,
#26971,#26972,#26973,#26974,#26975,#26976,#26977,#26978,#26979,#26980,#26981,
#26982,#26983,#26984,#26985,#26986,#26987,#26988,#26989,#26990,#26991,#26992,
#26993,#26994,#26995,#26996,#26997,#26998,#26999,#27000,#27001,#27002,#27003,
#27004,#27005,#27006,#27007,#27008,#27009,#27010),.UNSPECIFIED.,.F.,.F.)
B_SPLINE_CURVE_WITH_KNOTS((6,1,1,1,1,1,1,1,1,1,1,1,1,1,1,1,1,1,1,1,1,1,
1,1,1,1,1,1,1,1,1,1,1,1,1,1,1,1,1,1,1,1,1,1,1,1,1,1,1,1,1,1,1,1,1,1,1,1,
1,1,1,1,1,1,1,6),(-1.,-0.984615384615383,-0.969230769230768,-0.953846153846152,
-0.938461538461537,-0.923076923076922,-0.907692307692306,-0.892307692307691,
-0.876923076923076,-0.86153846153846,-0.846153846153845,-0.83076923076923,
-0.815384615384614,-0.799999999999999,-0.784615384615384,-0.769230769230768,
-0.753846153846153,-0.738461538461538,-0.723076923076922,-0.707692307692307,
-0.692307692307692,-0.676923076923076,-0.661538461538461,-0.646153846153846,
-0.63076923076923,-0.615384615384615,-0.6,-0.584615384615384,-0.569230769230769,
-0.553846153846154,-0.538461538461538,-0.523076923076923,-0.507692307692308,
-0.492307692307692,-0.476923076923077,-0.461538461538462,-0.446153846153846,
-0.430769230769231,-0.415384615384615,-0.4,-0.384615384615385,-0.369230769230769,
-0.353846153846154,-0.338461538461538,-0.323076923076923,-0.307692307692308,
-0.292307692307692,-0.276923076923077,-0.261538461538462,-0.246153846153846,
-0.230769230769231,-0.215384615384615,-0.2,-0.184615384615385,-0.169230769230769,
-0.153846153846154,-0.138461538461538,-0.123076923076923,-0.107692307692308,
-0.0923076923076923,-0.0769230769230769,-0.0615384615384615,-0.0461538461538462,
-0.0307692307692308,-0.0153846153846154,0.),.UNSPECIFIED.)
CURVE()
GEOMETRIC_REPRESENTATION_ITEM()
RATIONAL_B_SPLINE_CURVE((1.,1.,1.,1.,1.,1.,1.,1.,1.,1.,1.,1.,1.,1.,1.,1.,
1.,1.,1.,1.,1.,1.,1.,1.,1.,1.,1.,1.,1.,1.,1.,1.,1.,1.,1.,1.,1.,1.,1.,1.,
1.,1.,1.,1.,1.,1.,1.,1.,1.,1.,1.,1.,1.,1.,1.,1.,1.,1.,1.,1.,1.,1.,1.,1.,
1.,1.,1.,1.,1.,1.))
REPRESENTATION_ITEM('')
);
#106=(
BOUNDED_CURVE()
B_SPLINE_CURVE(5,(#27157,#27158,#27159,#27160,#27161,#27162,#27163,#27164,
#27165,#27166,#27167,#27168,#27169,#27170,#27171,#27172,#27173,#27174,#27175,
#27176,#27177,#27178,#27179,#27180,#27181,#27182,#27183,#27184,#27185,#27186,
#27187,#27188,#27189,#27190,#27191,#27192,#27193,#27194,#27195,#27196,#27197,
#27198,#27199,#27200,#27201,#27202,#27203,#27204,#27205,#27206,#27207,#27208,
#27209,#27210,#27211,#27212,#27213,#27214,#27215,#27216,#27217,#27218,#27219,
#27220,#27221,#27222,#27223,#27224,#27225,#27226),.UNSPECIFIED.,.F.,.F.)
B_SPLINE_CURVE_WITH_KNOTS((6,1,1,1,1,1,1,1,1,1,1,1,1,1,1,1,1,1,1,1,1,1,
1,1,1,1,1,1,1,1,1,1,1,1,1,1,1,1,1,1,1,1,1,1,1,1,1,1,1,1,1,1,1,1,1,1,1,1,
1,1,1,1,1,1,1,6),(-1.,-0.984615384615383,-0.969230769230768,-0.953846153846152,
-0.938461538461537,-0.923076923076922,-0.907692307692306,-0.892307692307691,
-0.876923076923076,-0.86153846153846,-0.846153846153845,-0.83076923076923,
-0.815384615384614,-0.799999999999999,-0.784615384615384,-0.769230769230768,
-0.753846153846153,-0.738461538461538,-0.723076923076922,-0.707692307692307,
-0.692307692307692,-0.676923076923076,-0.661538461538461,-0.646153846153846,
-0.63076923076923,-0.615384615384615,-0.6,-0.584615384615384,-0.569230769230769,
-0.553846153846154,-0.538461538461538,-0.523076923076923,-0.507692307692308,
-0.492307692307692,-0.476923076923077,-0.461538461538462,-0.446153846153846,
-0.430769230769231,-0.415384615384615,-0.4,-0.384615384615385,-0.369230769230769,
-0.353846153846154,-0.338461538461538,-0.323076923076923,-0.307692307692308,
-0.292307692307692,-0.276923076923077,-0.261538461538462,-0.246153846153846,
-0.230769230769231,-0.215384615384615,-0.2,-0.184615384615385,-0.169230769230769,
-0.153846153846154,-0.138461538461538,-0.123076923076923,-0.107692307692308,
-0.0923076923076923,-0.0769230769230769,-0.0615384615384615,-0.0461538461538462,
-0.0307692307692308,-0.0153846153846154,0.),.UNSPECIFIED.)
CURVE()
GEOMETRIC_REPRESENTATION_ITEM()
RATIONAL_B_SPLINE_CURVE((1.,1.,1.,1.,1.,1.,1.,1.,1.,1.,1.,1.,1.,1.,1.,1.,
1.,1.,1.,1.,1.,1.,1.,1.,1.,1.,1.,1.,1.,1.,1.,1.,1.,1.,1.,1.,1.,1.,1.,1.,
1.,1.,1.,1.,1.,1.,1.,1.,1.,1.,1.,1.,1.,1.,1.,1.,1.,1.,1.,1.,1.,1.,1.,1.,
1.,1.,1.,1.,1.,1.))
REPRESENTATION_ITEM('')
);
#107=(
BOUNDED_CURVE()
B_SPLINE_CURVE(5,(#27373,#27374,#27375,#27376,#27377,#27378,#27379,#27380,
#27381,#27382,#27383,#27384,#27385,#27386,#27387,#27388,#27389,#27390,#27391,
#27392,#27393,#27394,#27395,#27396,#27397,#27398,#27399,#27400,#27401,#27402,
#27403,#27404,#27405,#27406,#27407,#27408,#27409,#27410,#27411,#27412,#27413,
#27414,#27415,#27416,#27417,#27418,#27419,#27420,#27421,#27422,#27423,#27424,
#27425,#27426,#27427,#27428,#27429,#27430,#27431,#27432,#27433,#27434,#27435,
#27436,#27437,#27438,#27439,#27440,#27441,#27442),.UNSPECIFIED.,.F.,.F.)
B_SPLINE_CURVE_WITH_KNOTS((6,1,1,1,1,1,1,1,1,1,1,1,1,1,1,1,1,1,1,1,1,1,
1,1,1,1,1,1,1,1,1,1,1,1,1,1,1,1,1,1,1,1,1,1,1,1,1,1,1,1,1,1,1,1,1,1,1,1,
1,1,1,1,1,1,1,6),(-1.,-0.984615384615383,-0.969230769230768,-0.953846153846152,
-0.938461538461537,-0.923076923076922,-0.907692307692306,-0.892307692307691,
-0.876923076923076,-0.86153846153846,-0.846153846153845,-0.83076923076923,
-0.815384615384614,-0.799999999999999,-0.784615384615384,-0.769230769230768,
-0.753846153846153,-0.738461538461538,-0.723076923076922,-0.707692307692307,
-0.692307692307692,-0.676923076923076,-0.661538461538461,-0.646153846153846,
-0.63076923076923,-0.615384615384615,-0.6,-0.584615384615384,-0.569230769230769,
-0.553846153846154,-0.538461538461538,-0.523076923076923,-0.507692307692308,
-0.492307692307692,-0.476923076923077,-0.461538461538462,-0.446153846153846,
-0.430769230769231,-0.415384615384615,-0.4,-0.384615384615385,-0.369230769230769,
-0.353846153846154,-0.338461538461538,-0.323076923076923,-0.307692307692308,
-0.292307692307692,-0.276923076923077,-0.261538461538462,-0.246153846153846,
-0.230769230769231,-0.215384615384615,-0.2,-0.184615384615385,-0.169230769230769,
-0.153846153846154,-0.138461538461538,-0.123076923076923,-0.107692307692308,
-0.0923076923076923,-0.0769230769230769,-0.0615384615384615,-0.0461538461538462,
-0.0307692307692308,-0.0153846153846154,0.),.UNSPECIFIED.)
CURVE()
GEOMETRIC_REPRESENTATION_ITEM()
RATIONAL_B_SPLINE_CURVE((1.,1.,1.,1.,1.,1.,1.,1.,1.,1.,1.,1.,1.,1.,1.,1.,
1.,1.,1.,1.,1.,1.,1.,1.,1.,1.,1.,1.,1.,1.,1.,1.,1.,1.,1.,1.,1.,1.,1.,1.,
1.,1.,1.,1.,1.,1.,1.,1.,1.,1.,1.,1.,1.,1.,1.,1.,1.,1.,1.,1.,1.,1.,1.,1.,
1.,1.,1.,1.,1.,1.))
REPRESENTATION_ITEM('')
);
#108=(
BOUNDED_CURVE()
B_SPLINE_CURVE(5,(#27589,#27590,#27591,#27592,#27593,#27594,#27595,#27596,
#27597,#27598,#27599,#27600,#27601,#27602,#27603,#27604,#27605,#27606,#27607,
#27608,#27609,#27610,#27611,#27612,#27613,#27614,#27615,#27616,#27617,#27618,
#27619,#27620,#27621,#27622,#27623,#27624,#27625,#27626,#27627,#27628,#27629,
#27630,#27631,#27632,#27633,#27634,#27635,#27636,#27637,#27638,#27639,#27640,
#27641,#27642,#27643,#27644,#27645,#27646,#27647,#27648,#27649,#27650,#27651,
#27652,#27653,#27654,#27655,#27656,#27657,#27658),.UNSPECIFIED.,.F.,.F.)
B_SPLINE_CURVE_WITH_KNOTS((6,1,1,1,1,1,1,1,1,1,1,1,1,1,1,1,1,1,1,1,1,1,
1,1,1,1,1,1,1,1,1,1,1,1,1,1,1,1,1,1,1,1,1,1,1,1,1,1,1,1,1,1,1,1,1,1,1,1,
1,1,1,1,1,1,1,6),(-1.,-0.984615384615383,-0.969230769230768,-0.953846153846152,
-0.938461538461537,-0.923076923076922,-0.907692307692306,-0.892307692307691,
-0.876923076923076,-0.86153846153846,-0.846153846153845,-0.83076923076923,
-0.815384615384614,-0.799999999999999,-0.784615384615384,-0.769230769230768,
-0.753846153846153,-0.738461538461538,-0.723076923076922,-0.707692307692307,
-0.692307692307692,-0.676923076923076,-0.661538461538461,-0.646153846153846,
-0.63076923076923,-0.615384615384615,-0.6,-0.584615384615384,-0.569230769230769,
-0.553846153846154,-0.538461538461538,-0.523076923076923,-0.507692307692308,
-0.492307692307692,-0.476923076923077,-0.461538461538462,-0.446153846153846,
-0.430769230769231,-0.415384615384615,-0.4,-0.384615384615385,-0.369230769230769,
-0.353846153846154,-0.338461538461538,-0.323076923076923,-0.307692307692308,
-0.292307692307692,-0.276923076923077,-0.261538461538462,-0.246153846153846,
-0.230769230769231,-0.215384615384615,-0.2,-0.184615384615385,-0.169230769230769,
-0.153846153846154,-0.138461538461538,-0.123076923076923,-0.107692307692308,
-0.0923076923076923,-0.0769230769230769,-0.0615384615384615,-0.0461538461538462,
-0.0307692307692308,-0.0153846153846154,0.),.UNSPECIFIED.)
CURVE()
GEOMETRIC_REPRESENTATION_ITEM()
RATIONAL_B_SPLINE_CURVE((1.,1.,1.,1.,1.,1.,1.,1.,1.,1.,1.,1.,1.,1.,1.,1.,
1.,1.,1.,1.,1.,1.,1.,1.,1.,1.,1.,1.,1.,1.,1.,1.,1.,1.,1.,1.,1.,1.,1.,1.,
1.,1.,1.,1.,1.,1.,1.,1.,1.,1.,1.,1.,1.,1.,1.,1.,1.,1.,1.,1.,1.,1.,1.,1.,
1.,1.,1.,1.,1.,1.))
REPRESENTATION_ITEM('')
);
#109=(
BOUNDED_CURVE()
B_SPLINE_CURVE(5,(#27805,#27806,#27807,#27808,#27809,#27810,#27811,#27812,
#27813,#27814,#27815,#27816,#27817,#27818,#27819,#27820,#27821,#27822,#27823,
#27824,#27825,#27826,#27827,#27828,#27829,#27830,#27831,#27832,#27833,#27834,
#27835,#27836,#27837,#27838,#27839,#27840,#27841,#27842,#27843,#27844,#27845,
#27846,#27847,#27848,#27849,#27850,#27851,#27852,#27853,#27854,#27855,#27856,
#27857,#27858,#27859,#27860,#27861,#27862,#27863,#27864,#27865,#27866,#27867,
#27868,#27869,#27870,#27871,#27872,#27873,#27874),.UNSPECIFIED.,.F.,.F.)
B_SPLINE_CURVE_WITH_KNOTS((6,1,1,1,1,1,1,1,1,1,1,1,1,1,1,1,1,1,1,1,1,1,
1,1,1,1,1,1,1,1,1,1,1,1,1,1,1,1,1,1,1,1,1,1,1,1,1,1,1,1,1,1,1,1,1,1,1,1,
1,1,1,1,1,1,1,6),(-1.,-0.984615384615383,-0.969230769230768,-0.953846153846152,
-0.938461538461537,-0.923076923076922,-0.907692307692306,-0.892307692307691,
-0.876923076923076,-0.86153846153846,-0.846153846153845,-0.83076923076923,
-0.815384615384614,-0.799999999999999,-0.784615384615384,-0.769230769230768,
-0.753846153846153,-0.738461538461538,-0.723076923076922,-0.707692307692307,
-0.692307692307692,-0.676923076923076,-0.661538461538461,-0.646153846153846,
-0.63076923076923,-0.615384615384615,-0.6,-0.584615384615384,-0.569230769230769,
-0.553846153846154,-0.538461538461538,-0.523076923076923,-0.507692307692308,
-0.492307692307692,-0.476923076923077,-0.461538461538462,-0.446153846153846,
-0.430769230769231,-0.415384615384615,-0.4,-0.384615384615385,-0.369230769230769,
-0.353846153846154,-0.338461538461538,-0.323076923076923,-0.307692307692308,
-0.292307692307692,-0.276923076923077,-0.261538461538462,-0.246153846153846,
-0.230769230769231,-0.215384615384615,-0.2,-0.184615384615385,-0.169230769230769,
-0.153846153846154,-0.138461538461538,-0.123076923076923,-0.107692307692308,
-0.0923076923076923,-0.0769230769230769,-0.0615384615384615,-0.0461538461538462,
-0.0307692307692308,-0.0153846153846154,0.),.UNSPECIFIED.)
CURVE()
GEOMETRIC_REPRESENTATION_ITEM()
RATIONAL_B_SPLINE_CURVE((1.,1.,1.,1.,1.,1.,1.,1.,1.,1.,1.,1.,1.,1.,1.,1.,
1.,1.,1.,1.,1.,1.,1.,1.,1.,1.,1.,1.,1.,1.,1.,1.,1.,1.,1.,1.,1.,1.,1.,1.,
1.,1.,1.,1.,1.,1.,1.,1.,1.,1.,1.,1.,1.,1.,1.,1.,1.,1.,1.,1.,1.,1.,1.,1.,
1.,1.,1.,1.,1.,1.))
REPRESENTATION_ITEM('')
);
#110=(
BOUNDED_CURVE()
B_SPLINE_CURVE(5,(#28021,#28022,#28023,#28024,#28025,#28026,#28027,#28028,
#28029,#28030,#28031,#28032,#28033,#28034,#28035,#28036,#28037,#28038,#28039,
#28040,#28041,#28042,#28043,#28044,#28045,#28046,#28047,#28048,#28049,#28050,
#28051,#28052,#28053,#28054,#28055,#28056,#28057,#28058,#28059,#28060,#28061,
#28062,#28063,#28064,#28065,#28066,#28067,#28068,#28069,#28070,#28071,#28072,
#28073,#28074,#28075,#28076,#28077,#28078,#28079,#28080,#28081,#28082,#28083,
#28084,#28085,#28086,#28087,#28088,#28089,#28090),.UNSPECIFIED.,.F.,.F.)
B_SPLINE_CURVE_WITH_KNOTS((6,1,1,1,1,1,1,1,1,1,1,1,1,1,1,1,1,1,1,1,1,1,
1,1,1,1,1,1,1,1,1,1,1,1,1,1,1,1,1,1,1,1,1,1,1,1,1,1,1,1,1,1,1,1,1,1,1,1,
1,1,1,1,1,1,1,6),(-1.,-0.984615384615383,-0.969230769230768,-0.953846153846152,
-0.938461538461537,-0.923076923076922,-0.907692307692306,-0.892307692307691,
-0.876923076923076,-0.86153846153846,-0.846153846153845,-0.83076923076923,
-0.815384615384614,-0.799999999999999,-0.784615384615384,-0.769230769230768,
-0.753846153846153,-0.738461538461538,-0.723076923076922,-0.707692307692307,
-0.692307692307692,-0.676923076923076,-0.661538461538461,-0.646153846153846,
-0.63076923076923,-0.615384615384615,-0.6,-0.584615384615384,-0.569230769230769,
-0.553846153846154,-0.538461538461538,-0.523076923076923,-0.507692307692308,
-0.492307692307692,-0.476923076923077,-0.461538461538462,-0.446153846153846,
-0.430769230769231,-0.415384615384615,-0.4,-0.384615384615385,-0.369230769230769,
-0.353846153846154,-0.338461538461538,-0.323076923076923,-0.307692307692308,
-0.292307692307692,-0.276923076923077,-0.261538461538462,-0.246153846153846,
-0.230769230769231,-0.215384615384615,-0.2,-0.184615384615385,-0.169230769230769,
-0.153846153846154,-0.138461538461538,-0.123076923076923,-0.107692307692308,
-0.0923076923076923,-0.0769230769230769,-0.0615384615384615,-0.0461538461538462,
-0.0307692307692308,-0.0153846153846154,0.),.UNSPECIFIED.)
CURVE()
GEOMETRIC_REPRESENTATION_ITEM()
RATIONAL_B_SPLINE_CURVE((1.,1.,1.,1.,1.,1.,1.,1.,1.,1.,1.,1.,1.,1.,1.,1.,
1.,1.,1.,1.,1.,1.,1.,1.,1.,1.,1.,1.,1.,1.,1.,1.,1.,1.,1.,1.,1.,1.,1.,1.,
1.,1.,1.,1.,1.,1.,1.,1.,1.,1.,1.,1.,1.,1.,1.,1.,1.,1.,1.,1.,1.,1.,1.,1.,
1.,1.,1.,1.,1.,1.))
REPRESENTATION_ITEM('')
);
#111=(
BOUNDED_CURVE()
B_SPLINE_CURVE(5,(#28237,#28238,#28239,#28240,#28241,#28242,#28243,#28244,
#28245,#28246,#28247,#28248,#28249,#28250,#28251,#28252,#28253,#28254,#28255,
#28256,#28257,#28258,#28259,#28260,#28261,#28262,#28263,#28264,#28265,#28266,
#28267,#28268,#28269,#28270,#28271,#28272,#28273,#28274,#28275,#28276,#28277,
#28278,#28279,#28280,#28281,#28282,#28283,#28284,#28285,#28286,#28287,#28288,
#28289,#28290,#28291,#28292,#28293,#28294,#28295,#28296,#28297,#28298,#28299,
#28300,#28301,#28302,#28303,#28304,#28305,#28306),.UNSPECIFIED.,.F.,.F.)
B_SPLINE_CURVE_WITH_KNOTS((6,1,1,1,1,1,1,1,1,1,1,1,1,1,1,1,1,1,1,1,1,1,
1,1,1,1,1,1,1,1,1,1,1,1,1,1,1,1,1,1,1,1,1,1,1,1,1,1,1,1,1,1,1,1,1,1,1,1,
1,1,1,1,1,1,1,6),(-1.,-0.984615384615383,-0.969230769230768,-0.953846153846152,
-0.938461538461537,-0.923076923076922,-0.907692307692306,-0.892307692307691,
-0.876923076923076,-0.86153846153846,-0.846153846153845,-0.83076923076923,
-0.815384615384614,-0.799999999999999,-0.784615384615384,-0.769230769230768,
-0.753846153846153,-0.738461538461538,-0.723076923076922,-0.707692307692307,
-0.692307692307692,-0.676923076923076,-0.661538461538461,-0.646153846153846,
-0.63076923076923,-0.615384615384615,-0.6,-0.584615384615384,-0.569230769230769,
-0.553846153846154,-0.538461538461538,-0.523076923076923,-0.507692307692308,
-0.492307692307692,-0.476923076923077,-0.461538461538462,-0.446153846153846,
-0.430769230769231,-0.415384615384615,-0.4,-0.384615384615385,-0.369230769230769,
-0.353846153846154,-0.338461538461538,-0.323076923076923,-0.307692307692308,
-0.292307692307692,-0.276923076923077,-0.261538461538462,-0.246153846153846,
-0.230769230769231,-0.215384615384615,-0.2,-0.184615384615385,-0.169230769230769,
-0.153846153846154,-0.138461538461538,-0.123076923076923,-0.107692307692308,
-0.0923076923076923,-0.0769230769230769,-0.0615384615384615,-0.0461538461538462,
-0.0307692307692308,-0.0153846153846154,0.),.UNSPECIFIED.)
CURVE()
GEOMETRIC_REPRESENTATION_ITEM()
RATIONAL_B_SPLINE_CURVE((1.,1.,1.,1.,1.,1.,1.,1.,1.,1.,1.,1.,1.,1.,1.,1.,
1.,1.,1.,1.,1.,1.,1.,1.,1.,1.,1.,1.,1.,1.,1.,1.,1.,1.,1.,1.,1.,1.,1.,1.,
1.,1.,1.,1.,1.,1.,1.,1.,1.,1.,1.,1.,1.,1.,1.,1.,1.,1.,1.,1.,1.,1.,1.,1.,
1.,1.,1.,1.,1.,1.))
REPRESENTATION_ITEM('')
);
#112=(
BOUNDED_CURVE()
B_SPLINE_CURVE(5,(#28453,#28454,#28455,#28456,#28457,#28458,#28459,#28460,
#28461,#28462,#28463,#28464,#28465,#28466,#28467,#28468,#28469,#28470,#28471,
#28472,#28473,#28474,#28475,#28476,#28477,#28478,#28479,#28480,#28481,#28482,
#28483,#28484,#28485,#28486,#28487,#28488,#28489,#28490,#28491,#28492,#28493,
#28494,#28495,#28496,#28497,#28498,#28499,#28500,#28501,#28502,#28503,#28504,
#28505,#28506,#28507,#28508,#28509,#28510,#28511,#28512,#28513,#28514,#28515,
#28516,#28517,#28518,#28519,#28520,#28521,#28522),.UNSPECIFIED.,.F.,.F.)
B_SPLINE_CURVE_WITH_KNOTS((6,1,1,1,1,1,1,1,1,1,1,1,1,1,1,1,1,1,1,1,1,1,
1,1,1,1,1,1,1,1,1,1,1,1,1,1,1,1,1,1,1,1,1,1,1,1,1,1,1,1,1,1,1,1,1,1,1,1,
1,1,1,1,1,1,1,6),(-1.,-0.984615384615383,-0.969230769230768,-0.953846153846152,
-0.938461538461537,-0.923076923076922,-0.907692307692306,-0.892307692307691,
-0.876923076923076,-0.86153846153846,-0.846153846153845,-0.83076923076923,
-0.815384615384614,-0.799999999999999,-0.784615384615384,-0.769230769230768,
-0.753846153846153,-0.738461538461538,-0.723076923076922,-0.707692307692307,
-0.692307692307692,-0.676923076923076,-0.661538461538461,-0.646153846153846,
-0.63076923076923,-0.615384615384615,-0.6,-0.584615384615384,-0.569230769230769,
-0.553846153846154,-0.538461538461538,-0.523076923076923,-0.507692307692308,
-0.492307692307692,-0.476923076923077,-0.461538461538462,-0.446153846153846,
-0.430769230769231,-0.415384615384615,-0.4,-0.384615384615385,-0.369230769230769,
-0.353846153846154,-0.338461538461538,-0.323076923076923,-0.307692307692308,
-0.292307692307692,-0.276923076923077,-0.261538461538462,-0.246153846153846,
-0.230769230769231,-0.215384615384615,-0.2,-0.184615384615385,-0.169230769230769,
-0.153846153846154,-0.138461538461538,-0.123076923076923,-0.107692307692308,
-0.0923076923076923,-0.0769230769230769,-0.0615384615384615,-0.0461538461538462,
-0.0307692307692308,-0.0153846153846154,0.),.UNSPECIFIED.)
CURVE()
GEOMETRIC_REPRESENTATION_ITEM()
RATIONAL_B_SPLINE_CURVE((1.,1.,1.,1.,1.,1.,1.,1.,1.,1.,1.,1.,1.,1.,1.,1.,
1.,1.,1.,1.,1.,1.,1.,1.,1.,1.,1.,1.,1.,1.,1.,1.,1.,1.,1.,1.,1.,1.,1.,1.,
1.,1.,1.,1.,1.,1.,1.,1.,1.,1.,1.,1.,1.,1.,1.,1.,1.,1.,1.,1.,1.,1.,1.,1.,
1.,1.,1.,1.,1.,1.))
REPRESENTATION_ITEM('')
);
#113=(
BOUNDED_CURVE()
B_SPLINE_CURVE(5,(#28669,#28670,#28671,#28672,#28673,#28674,#28675,#28676,
#28677,#28678,#28679,#28680,#28681,#28682,#28683,#28684,#28685,#28686,#28687,
#28688,#28689,#28690,#28691,#28692,#28693,#28694,#28695,#28696,#28697,#28698,
#28699,#28700,#28701,#28702,#28703,#28704,#28705,#28706,#28707,#28708,#28709,
#28710,#28711,#28712,#28713,#28714,#28715,#28716,#28717,#28718,#28719,#28720,
#28721,#28722,#28723,#28724,#28725,#28726,#28727,#28728,#28729,#28730,#28731,
#28732,#28733,#28734,#28735,#28736,#28737,#28738),.UNSPECIFIED.,.F.,.F.)
B_SPLINE_CURVE_WITH_KNOTS((6,1,1,1,1,1,1,1,1,1,1,1,1,1,1,1,1,1,1,1,1,1,
1,1,1,1,1,1,1,1,1,1,1,1,1,1,1,1,1,1,1,1,1,1,1,1,1,1,1,1,1,1,1,1,1,1,1,1,
1,1,1,1,1,1,1,6),(-1.,-0.984615384615383,-0.969230769230768,-0.953846153846152,
-0.938461538461537,-0.923076923076922,-0.907692307692306,-0.892307692307691,
-0.876923076923076,-0.86153846153846,-0.846153846153845,-0.83076923076923,
-0.815384615384614,-0.799999999999999,-0.784615384615384,-0.769230769230768,
-0.753846153846153,-0.738461538461538,-0.723076923076922,-0.707692307692307,
-0.692307692307692,-0.676923076923076,-0.661538461538461,-0.646153846153846,
-0.63076923076923,-0.615384615384615,-0.6,-0.584615384615384,-0.569230769230769,
-0.553846153846154,-0.538461538461538,-0.523076923076923,-0.507692307692308,
-0.492307692307692,-0.476923076923077,-0.461538461538462,-0.446153846153846,
-0.430769230769231,-0.415384615384615,-0.4,-0.384615384615385,-0.369230769230769,
-0.353846153846154,-0.338461538461538,-0.323076923076923,-0.307692307692308,
-0.292307692307692,-0.276923076923077,-0.261538461538462,-0.246153846153846,
-0.230769230769231,-0.215384615384615,-0.2,-0.184615384615385,-0.169230769230769,
-0.153846153846154,-0.138461538461538,-0.123076923076923,-0.107692307692308,
-0.0923076923076923,-0.0769230769230769,-0.0615384615384615,-0.0461538461538462,
-0.0307692307692308,-0.0153846153846154,0.),.UNSPECIFIED.)
CURVE()
GEOMETRIC_REPRESENTATION_ITEM()
RATIONAL_B_SPLINE_CURVE((1.,1.,1.,1.,1.,1.,1.,1.,1.,1.,1.,1.,1.,1.,1.,1.,
1.,1.,1.,1.,1.,1.,1.,1.,1.,1.,1.,1.,1.,1.,1.,1.,1.,1.,1.,1.,1.,1.,1.,1.,
1.,1.,1.,1.,1.,1.,1.,1.,1.,1.,1.,1.,1.,1.,1.,1.,1.,1.,1.,1.,1.,1.,1.,1.,
1.,1.,1.,1.,1.,1.))
REPRESENTATION_ITEM('')
);
#114=(
BOUNDED_CURVE()
B_SPLINE_CURVE(5,(#28885,#28886,#28887,#28888,#28889,#28890,#28891,#28892,
#28893,#28894,#28895,#28896,#28897,#28898,#28899,#28900,#28901,#28902,#28903,
#28904,#28905,#28906,#28907,#28908,#28909,#28910,#28911,#28912,#28913,#28914,
#28915,#28916,#28917,#28918,#28919,#28920,#28921,#28922,#28923,#28924,#28925,
#28926,#28927,#28928,#28929,#28930,#28931,#28932,#28933,#28934,#28935,#28936,
#28937,#28938,#28939,#28940,#28941,#28942,#28943,#28944,#28945,#28946,#28947,
#28948,#28949,#28950,#28951,#28952,#28953,#28954),.UNSPECIFIED.,.F.,.F.)
B_SPLINE_CURVE_WITH_KNOTS((6,1,1,1,1,1,1,1,1,1,1,1,1,1,1,1,1,1,1,1,1,1,
1,1,1,1,1,1,1,1,1,1,1,1,1,1,1,1,1,1,1,1,1,1,1,1,1,1,1,1,1,1,1,1,1,1,1,1,
1,1,1,1,1,1,1,6),(-1.,-0.984615384615383,-0.969230769230768,-0.953846153846152,
-0.938461538461537,-0.923076923076922,-0.907692307692306,-0.892307692307691,
-0.876923076923076,-0.86153846153846,-0.846153846153845,-0.83076923076923,
-0.815384615384614,-0.799999999999999,-0.784615384615384,-0.769230769230768,
-0.753846153846153,-0.738461538461538,-0.723076923076922,-0.707692307692307,
-0.692307692307692,-0.676923076923076,-0.661538461538461,-0.646153846153846,
-0.63076923076923,-0.615384615384615,-0.6,-0.584615384615384,-0.569230769230769,
-0.553846153846154,-0.538461538461538,-0.523076923076923,-0.507692307692308,
-0.492307692307692,-0.476923076923077,-0.461538461538462,-0.446153846153846,
-0.430769230769231,-0.415384615384615,-0.4,-0.384615384615385,-0.369230769230769,
-0.353846153846154,-0.338461538461538,-0.323076923076923,-0.307692307692308,
-0.292307692307692,-0.276923076923077,-0.261538461538462,-0.246153846153846,
-0.230769230769231,-0.215384615384615,-0.2,-0.184615384615385,-0.169230769230769,
-0.153846153846154,-0.138461538461538,-0.123076923076923,-0.107692307692308,
-0.0923076923076923,-0.0769230769230769,-0.0615384615384615,-0.0461538461538462,
-0.0307692307692308,-0.0153846153846154,0.),.UNSPECIFIED.)
CURVE()
GEOMETRIC_REPRESENTATION_ITEM()
RATIONAL_B_SPLINE_CURVE((1.,1.,1.,1.,1.,1.,1.,1.,1.,1.,1.,1.,1.,1.,1.,1.,
1.,1.,1.,1.,1.,1.,1.,1.,1.,1.,1.,1.,1.,1.,1.,1.,1.,1.,1.,1.,1.,1.,1.,1.,
1.,1.,1.,1.,1.,1.,1.,1.,1.,1.,1.,1.,1.,1.,1.,1.,1.,1.,1.,1.,1.,1.,1.,1.,
1.,1.,1.,1.,1.,1.))
REPRESENTATION_ITEM('')
);
#115=(
BOUNDED_CURVE()
B_SPLINE_CURVE(5,(#29101,#29102,#29103,#29104,#29105,#29106,#29107,#29108,
#29109,#29110,#29111,#29112,#29113,#29114,#29115,#29116,#29117,#29118,#29119,
#29120,#29121,#29122,#29123,#29124,#29125,#29126,#29127,#29128,#29129,#29130,
#29131,#29132,#29133,#29134,#29135,#29136,#29137,#29138,#29139,#29140,#29141,
#29142,#29143,#29144,#29145,#29146,#29147,#29148,#29149,#29150,#29151,#29152,
#29153,#29154,#29155,#29156,#29157,#29158,#29159,#29160,#29161,#29162,#29163,
#29164,#29165,#29166,#29167,#29168,#29169,#29170),.UNSPECIFIED.,.F.,.F.)
B_SPLINE_CURVE_WITH_KNOTS((6,1,1,1,1,1,1,1,1,1,1,1,1,1,1,1,1,1,1,1,1,1,
1,1,1,1,1,1,1,1,1,1,1,1,1,1,1,1,1,1,1,1,1,1,1,1,1,1,1,1,1,1,1,1,1,1,1,1,
1,1,1,1,1,1,1,6),(-1.,-0.984615384615383,-0.969230769230768,-0.953846153846152,
-0.938461538461537,-0.923076923076922,-0.907692307692306,-0.892307692307691,
-0.876923076923076,-0.86153846153846,-0.846153846153845,-0.83076923076923,
-0.815384615384614,-0.799999999999999,-0.784615384615384,-0.769230769230768,
-0.753846153846153,-0.738461538461538,-0.723076923076922,-0.707692307692307,
-0.692307692307692,-0.676923076923076,-0.661538461538461,-0.646153846153846,
-0.63076923076923,-0.615384615384615,-0.6,-0.584615384615384,-0.569230769230769,
-0.553846153846154,-0.538461538461538,-0.523076923076923,-0.507692307692308,
-0.492307692307692,-0.476923076923077,-0.461538461538462,-0.446153846153846,
-0.430769230769231,-0.415384615384615,-0.4,-0.384615384615385,-0.369230769230769,
-0.353846153846154,-0.338461538461538,-0.323076923076923,-0.307692307692308,
-0.292307692307692,-0.276923076923077,-0.261538461538462,-0.246153846153846,
-0.230769230769231,-0.215384615384615,-0.2,-0.184615384615385,-0.169230769230769,
-0.153846153846154,-0.138461538461538,-0.123076923076923,-0.107692307692308,
-0.0923076923076923,-0.0769230769230769,-0.0615384615384615,-0.0461538461538462,
-0.0307692307692308,-0.0153846153846154,0.),.UNSPECIFIED.)
CURVE()
GEOMETRIC_REPRESENTATION_ITEM()
RATIONAL_B_SPLINE_CURVE((1.,1.,1.,1.,1.,1.,1.,1.,1.,1.,1.,1.,1.,1.,1.,1.,
1.,1.,1.,1.,1.,1.,1.,1.,1.,1.,1.,1.,1.,1.,1.,1.,1.,1.,1.,1.,1.,1.,1.,1.,
1.,1.,1.,1.,1.,1.,1.,1.,1.,1.,1.,1.,1.,1.,1.,1.,1.,1.,1.,1.,1.,1.,1.,1.,
1.,1.,1.,1.,1.,1.))
REPRESENTATION_ITEM('')
);
#116=(
BOUNDED_CURVE()
B_SPLINE_CURVE(5,(#29317,#29318,#29319,#29320,#29321,#29322,#29323,#29324,
#29325,#29326,#29327,#29328,#29329,#29330,#29331,#29332,#29333,#29334,#29335,
#29336,#29337,#29338,#29339,#29340,#29341,#29342,#29343,#29344,#29345,#29346,
#29347,#29348,#29349,#29350,#29351,#29352,#29353,#29354,#29355,#29356,#29357,
#29358,#29359,#29360,#29361,#29362,#29363,#29364,#29365,#29366,#29367,#29368,
#29369,#29370,#29371,#29372,#29373,#29374,#29375,#29376,#29377,#29378,#29379,
#29380,#29381,#29382,#29383,#29384,#29385,#29386),.UNSPECIFIED.,.F.,.F.)
B_SPLINE_CURVE_WITH_KNOTS((6,1,1,1,1,1,1,1,1,1,1,1,1,1,1,1,1,1,1,1,1,1,
1,1,1,1,1,1,1,1,1,1,1,1,1,1,1,1,1,1,1,1,1,1,1,1,1,1,1,1,1,1,1,1,1,1,1,1,
1,1,1,1,1,1,1,6),(-1.,-0.984615384615383,-0.969230769230768,-0.953846153846152,
-0.938461538461537,-0.923076923076922,-0.907692307692306,-0.892307692307691,
-0.876923076923076,-0.86153846153846,-0.846153846153845,-0.83076923076923,
-0.815384615384614,-0.799999999999999,-0.784615384615384,-0.769230769230768,
-0.753846153846153,-0.738461538461538,-0.723076923076922,-0.707692307692307,
-0.692307692307692,-0.676923076923076,-0.661538461538461,-0.646153846153846,
-0.63076923076923,-0.615384615384615,-0.6,-0.584615384615384,-0.569230769230769,
-0.553846153846154,-0.538461538461538,-0.523076923076923,-0.507692307692308,
-0.492307692307692,-0.476923076923077,-0.461538461538462,-0.446153846153846,
-0.430769230769231,-0.415384615384615,-0.4,-0.384615384615385,-0.369230769230769,
-0.353846153846154,-0.338461538461538,-0.323076923076923,-0.307692307692308,
-0.292307692307692,-0.276923076923077,-0.261538461538462,-0.246153846153846,
-0.230769230769231,-0.215384615384615,-0.2,-0.184615384615385,-0.169230769230769,
-0.153846153846154,-0.138461538461538,-0.123076923076923,-0.107692307692308,
-0.0923076923076923,-0.0769230769230769,-0.0615384615384615,-0.0461538461538462,
-0.0307692307692308,-0.0153846153846154,0.),.UNSPECIFIED.)
CURVE()
GEOMETRIC_REPRESENTATION_ITEM()
RATIONAL_B_SPLINE_CURVE((1.,1.,1.,1.,1.,1.,1.,1.,1.,1.,1.,1.,1.,1.,1.,1.,
1.,1.,1.,1.,1.,1.,1.,1.,1.,1.,1.,1.,1.,1.,1.,1.,1.,1.,1.,1.,1.,1.,1.,1.,
1.,1.,1.,1.,1.,1.,1.,1.,1.,1.,1.,1.,1.,1.,1.,1.,1.,1.,1.,1.,1.,1.,1.,1.,
1.,1.,1.,1.,1.,1.))
REPRESENTATION_ITEM('')
);
#117=(
BOUNDED_CURVE()
B_SPLINE_CURVE(5,(#29533,#29534,#29535,#29536,#29537,#29538,#29539,#29540,
#29541,#29542,#29543,#29544,#29545,#29546,#29547,#29548,#29549,#29550,#29551,
#29552,#29553,#29554,#29555,#29556,#29557,#29558,#29559,#29560,#29561,#29562,
#29563,#29564,#29565,#29566,#29567,#29568,#29569,#29570,#29571,#29572,#29573,
#29574,#29575,#29576,#29577,#29578,#29579,#29580,#29581,#29582,#29583,#29584,
#29585,#29586,#29587,#29588,#29589,#29590,#29591,#29592,#29593,#29594,#29595,
#29596,#29597,#29598,#29599,#29600,#29601,#29602),.UNSPECIFIED.,.F.,.F.)
B_SPLINE_CURVE_WITH_KNOTS((6,1,1,1,1,1,1,1,1,1,1,1,1,1,1,1,1,1,1,1,1,1,
1,1,1,1,1,1,1,1,1,1,1,1,1,1,1,1,1,1,1,1,1,1,1,1,1,1,1,1,1,1,1,1,1,1,1,1,
1,1,1,1,1,1,1,6),(-1.,-0.984615384615383,-0.969230769230768,-0.953846153846152,
-0.938461538461537,-0.923076923076922,-0.907692307692306,-0.892307692307691,
-0.876923076923076,-0.86153846153846,-0.846153846153845,-0.83076923076923,
-0.815384615384614,-0.799999999999999,-0.784615384615384,-0.769230769230768,
-0.753846153846153,-0.738461538461538,-0.723076923076922,-0.707692307692307,
-0.692307692307692,-0.676923076923076,-0.661538461538461,-0.646153846153846,
-0.63076923076923,-0.615384615384615,-0.6,-0.584615384615384,-0.569230769230769,
-0.553846153846154,-0.538461538461538,-0.523076923076923,-0.507692307692308,
-0.492307692307692,-0.476923076923077,-0.461538461538462,-0.446153846153846,
-0.430769230769231,-0.415384615384615,-0.4,-0.384615384615385,-0.369230769230769,
-0.353846153846154,-0.338461538461538,-0.323076923076923,-0.307692307692308,
-0.292307692307692,-0.276923076923077,-0.261538461538462,-0.246153846153846,
-0.230769230769231,-0.215384615384615,-0.2,-0.184615384615385,-0.169230769230769,
-0.153846153846154,-0.138461538461538,-0.123076923076923,-0.107692307692308,
-0.0923076923076923,-0.0769230769230769,-0.0615384615384615,-0.0461538461538462,
-0.0307692307692308,-0.0153846153846154,0.),.UNSPECIFIED.)
CURVE()
GEOMETRIC_REPRESENTATION_ITEM()
RATIONAL_B_SPLINE_CURVE((1.,1.,1.,1.,1.,1.,1.,1.,1.,1.,1.,1.,1.,1.,1.,1.,
1.,1.,1.,1.,1.,1.,1.,1.,1.,1.,1.,1.,1.,1.,1.,1.,1.,1.,1.,1.,1.,1.,1.,1.,
1.,1.,1.,1.,1.,1.,1.,1.,1.,1.,1.,1.,1.,1.,1.,1.,1.,1.,1.,1.,1.,1.,1.,1.,
1.,1.,1.,1.,1.,1.))
REPRESENTATION_ITEM('')
);
#118=(
BOUNDED_CURVE()
B_SPLINE_CURVE(5,(#29749,#29750,#29751,#29752,#29753,#29754,#29755,#29756,
#29757,#29758,#29759,#29760,#29761,#29762,#29763,#29764,#29765,#29766,#29767,
#29768,#29769,#29770,#29771,#29772,#29773,#29774,#29775,#29776,#29777,#29778,
#29779,#29780,#29781,#29782,#29783,#29784,#29785,#29786,#29787,#29788,#29789,
#29790,#29791,#29792,#29793,#29794,#29795,#29796,#29797,#29798,#29799,#29800,
#29801,#29802,#29803,#29804,#29805,#29806,#29807,#29808,#29809,#29810,#29811,
#29812,#29813,#29814,#29815,#29816,#29817,#29818),.UNSPECIFIED.,.F.,.F.)
B_SPLINE_CURVE_WITH_KNOTS((6,1,1,1,1,1,1,1,1,1,1,1,1,1,1,1,1,1,1,1,1,1,
1,1,1,1,1,1,1,1,1,1,1,1,1,1,1,1,1,1,1,1,1,1,1,1,1,1,1,1,1,1,1,1,1,1,1,1,
1,1,1,1,1,1,1,6),(-1.,-0.984615384615383,-0.969230769230768,-0.953846153846152,
-0.938461538461537,-0.923076923076922,-0.907692307692306,-0.892307692307691,
-0.876923076923076,-0.86153846153846,-0.846153846153845,-0.83076923076923,
-0.815384615384614,-0.799999999999999,-0.784615384615384,-0.769230769230768,
-0.753846153846153,-0.738461538461538,-0.723076923076922,-0.707692307692307,
-0.692307692307692,-0.676923076923076,-0.661538461538461,-0.646153846153846,
-0.63076923076923,-0.615384615384615,-0.6,-0.584615384615384,-0.569230769230769,
-0.553846153846154,-0.538461538461538,-0.523076923076923,-0.507692307692308,
-0.492307692307692,-0.476923076923077,-0.461538461538462,-0.446153846153846,
-0.430769230769231,-0.415384615384615,-0.4,-0.384615384615385,-0.369230769230769,
-0.353846153846154,-0.338461538461538,-0.323076923076923,-0.307692307692308,
-0.292307692307692,-0.276923076923077,-0.261538461538462,-0.246153846153846,
-0.230769230769231,-0.215384615384615,-0.2,-0.184615384615385,-0.169230769230769,
-0.153846153846154,-0.138461538461538,-0.123076923076923,-0.107692307692308,
-0.0923076923076923,-0.0769230769230769,-0.0615384615384615,-0.0461538461538462,
-0.0307692307692308,-0.0153846153846154,0.),.UNSPECIFIED.)
CURVE()
GEOMETRIC_REPRESENTATION_ITEM()
RATIONAL_B_SPLINE_CURVE((1.,1.,1.,1.,1.,1.,1.,1.,1.,1.,1.,1.,1.,1.,1.,1.,
1.,1.,1.,1.,1.,1.,1.,1.,1.,1.,1.,1.,1.,1.,1.,1.,1.,1.,1.,1.,1.,1.,1.,1.,
1.,1.,1.,1.,1.,1.,1.,1.,1.,1.,1.,1.,1.,1.,1.,1.,1.,1.,1.,1.,1.,1.,1.,1.,
1.,1.,1.,1.,1.,1.))
REPRESENTATION_ITEM('')
);
#119=(
BOUNDED_CURVE()
B_SPLINE_CURVE(5,(#29965,#29966,#29967,#29968,#29969,#29970,#29971,#29972,
#29973,#29974,#29975,#29976,#29977,#29978,#29979,#29980,#29981,#29982,#29983,
#29984,#29985,#29986,#29987,#29988,#29989,#29990,#29991,#29992,#29993,#29994,
#29995,#29996,#29997,#29998,#29999,#30000,#30001,#30002,#30003,#30004,#30005,
#30006,#30007,#30008,#30009,#30010,#30011,#30012,#30013,#30014,#30015,#30016,
#30017,#30018,#30019,#30020,#30021,#30022,#30023,#30024,#30025,#30026,#30027,
#30028,#30029,#30030,#30031,#30032,#30033,#30034),.UNSPECIFIED.,.F.,.F.)
B_SPLINE_CURVE_WITH_KNOTS((6,1,1,1,1,1,1,1,1,1,1,1,1,1,1,1,1,1,1,1,1,1,
1,1,1,1,1,1,1,1,1,1,1,1,1,1,1,1,1,1,1,1,1,1,1,1,1,1,1,1,1,1,1,1,1,1,1,1,
1,1,1,1,1,1,1,6),(-1.,-0.984615384615383,-0.969230769230768,-0.953846153846152,
-0.938461538461537,-0.923076923076922,-0.907692307692306,-0.892307692307691,
-0.876923076923076,-0.86153846153846,-0.846153846153845,-0.83076923076923,
-0.815384615384614,-0.799999999999999,-0.784615384615384,-0.769230769230768,
-0.753846153846153,-0.738461538461538,-0.723076923076922,-0.707692307692307,
-0.692307692307692,-0.676923076923076,-0.661538461538461,-0.646153846153846,
-0.63076923076923,-0.615384615384615,-0.6,-0.584615384615384,-0.569230769230769,
-0.553846153846154,-0.538461538461538,-0.523076923076923,-0.507692307692308,
-0.492307692307692,-0.476923076923077,-0.461538461538462,-0.446153846153846,
-0.430769230769231,-0.415384615384615,-0.4,-0.384615384615385,-0.369230769230769,
-0.353846153846154,-0.338461538461538,-0.323076923076923,-0.307692307692308,
-0.292307692307692,-0.276923076923077,-0.261538461538462,-0.246153846153846,
-0.230769230769231,-0.215384615384615,-0.2,-0.184615384615385,-0.169230769230769,
-0.153846153846154,-0.138461538461538,-0.123076923076923,-0.107692307692308,
-0.0923076923076923,-0.0769230769230769,-0.0615384615384615,-0.0461538461538462,
-0.0307692307692308,-0.0153846153846154,0.),.UNSPECIFIED.)
CURVE()
GEOMETRIC_REPRESENTATION_ITEM()
RATIONAL_B_SPLINE_CURVE((1.,1.,1.,1.,1.,1.,1.,1.,1.,1.,1.,1.,1.,1.,1.,1.,
1.,1.,1.,1.,1.,1.,1.,1.,1.,1.,1.,1.,1.,1.,1.,1.,1.,1.,1.,1.,1.,1.,1.,1.,
1.,1.,1.,1.,1.,1.,1.,1.,1.,1.,1.,1.,1.,1.,1.,1.,1.,1.,1.,1.,1.,1.,1.,1.,
1.,1.,1.,1.,1.,1.))
REPRESENTATION_ITEM('')
);
#120=(
BOUNDED_CURVE()
B_SPLINE_CURVE(5,(#30181,#30182,#30183,#30184,#30185,#30186,#30187,#30188,
#30189,#30190,#30191,#30192,#30193,#30194,#30195,#30196,#30197,#30198,#30199,
#30200,#30201,#30202,#30203,#30204,#30205,#30206,#30207,#30208,#30209,#30210,
#30211,#30212,#30213,#30214,#30215,#30216,#30217,#30218,#30219,#30220,#30221,
#30222,#30223,#30224,#30225,#30226,#30227,#30228,#30229,#30230,#30231,#30232,
#30233,#30234,#30235,#30236,#30237,#30238,#30239,#30240,#30241,#30242,#30243,
#30244,#30245,#30246,#30247,#30248,#30249,#30250),.UNSPECIFIED.,.F.,.F.)
B_SPLINE_CURVE_WITH_KNOTS((6,1,1,1,1,1,1,1,1,1,1,1,1,1,1,1,1,1,1,1,1,1,
1,1,1,1,1,1,1,1,1,1,1,1,1,1,1,1,1,1,1,1,1,1,1,1,1,1,1,1,1,1,1,1,1,1,1,1,
1,1,1,1,1,1,1,6),(-1.,-0.984615384615383,-0.969230769230768,-0.953846153846152,
-0.938461538461537,-0.923076923076922,-0.907692307692306,-0.892307692307691,
-0.876923076923076,-0.86153846153846,-0.846153846153845,-0.83076923076923,
-0.815384615384614,-0.799999999999999,-0.784615384615384,-0.769230769230768,
-0.753846153846153,-0.738461538461538,-0.723076923076922,-0.707692307692307,
-0.692307692307692,-0.676923076923076,-0.661538461538461,-0.646153846153846,
-0.63076923076923,-0.615384615384615,-0.6,-0.584615384615384,-0.569230769230769,
-0.553846153846154,-0.538461538461538,-0.523076923076923,-0.507692307692308,
-0.492307692307692,-0.476923076923077,-0.461538461538462,-0.446153846153846,
-0.430769230769231,-0.415384615384615,-0.4,-0.384615384615385,-0.369230769230769,
-0.353846153846154,-0.338461538461538,-0.323076923076923,-0.307692307692308,
-0.292307692307692,-0.276923076923077,-0.261538461538462,-0.246153846153846,
-0.230769230769231,-0.215384615384615,-0.2,-0.184615384615385,-0.169230769230769,
-0.153846153846154,-0.138461538461538,-0.123076923076923,-0.107692307692308,
-0.0923076923076923,-0.0769230769230769,-0.0615384615384615,-0.0461538461538462,
-0.0307692307692308,-0.0153846153846154,0.),.UNSPECIFIED.)
CURVE()
GEOMETRIC_REPRESENTATION_ITEM()
RATIONAL_B_SPLINE_CURVE((1.,1.,1.,1.,1.,1.,1.,1.,1.,1.,1.,1.,1.,1.,1.,1.,
1.,1.,1.,1.,1.,1.,1.,1.,1.,1.,1.,1.,1.,1.,1.,1.,1.,1.,1.,1.,1.,1.,1.,1.,
1.,1.,1.,1.,1.,1.,1.,1.,1.,1.,1.,1.,1.,1.,1.,1.,1.,1.,1.,1.,1.,1.,1.,1.,
1.,1.,1.,1.,1.,1.))
REPRESENTATION_ITEM('')
);
#121=(
BOUNDED_CURVE()
B_SPLINE_CURVE(5,(#30397,#30398,#30399,#30400,#30401,#30402,#30403,#30404,
#30405,#30406,#30407,#30408,#30409,#30410,#30411,#30412,#30413,#30414,#30415,
#30416,#30417,#30418,#30419,#30420,#30421,#30422,#30423,#30424,#30425,#30426,
#30427,#30428,#30429,#30430,#30431,#30432,#30433,#30434,#30435,#30436,#30437,
#30438,#30439,#30440,#30441,#30442,#30443,#30444,#30445,#30446,#30447,#30448,
#30449,#30450,#30451,#30452,#30453,#30454,#30455,#30456,#30457,#30458,#30459,
#30460,#30461,#30462,#30463,#30464,#30465,#30466),.UNSPECIFIED.,.F.,.F.)
B_SPLINE_CURVE_WITH_KNOTS((6,1,1,1,1,1,1,1,1,1,1,1,1,1,1,1,1,1,1,1,1,1,
1,1,1,1,1,1,1,1,1,1,1,1,1,1,1,1,1,1,1,1,1,1,1,1,1,1,1,1,1,1,1,1,1,1,1,1,
1,1,1,1,1,1,1,6),(-1.,-0.984615384615383,-0.969230769230768,-0.953846153846152,
-0.938461538461537,-0.923076923076922,-0.907692307692306,-0.892307692307691,
-0.876923076923076,-0.86153846153846,-0.846153846153845,-0.83076923076923,
-0.815384615384614,-0.799999999999999,-0.784615384615384,-0.769230769230768,
-0.753846153846153,-0.738461538461538,-0.723076923076922,-0.707692307692307,
-0.692307692307692,-0.676923076923076,-0.661538461538461,-0.646153846153846,
-0.63076923076923,-0.615384615384615,-0.6,-0.584615384615384,-0.569230769230769,
-0.553846153846154,-0.538461538461538,-0.523076923076923,-0.507692307692308,
-0.492307692307692,-0.476923076923077,-0.461538461538462,-0.446153846153846,
-0.430769230769231,-0.415384615384615,-0.4,-0.384615384615385,-0.369230769230769,
-0.353846153846154,-0.338461538461538,-0.323076923076923,-0.307692307692308,
-0.292307692307692,-0.276923076923077,-0.261538461538462,-0.246153846153846,
-0.230769230769231,-0.215384615384615,-0.2,-0.184615384615385,-0.169230769230769,
-0.153846153846154,-0.138461538461538,-0.123076923076923,-0.107692307692308,
-0.0923076923076923,-0.0769230769230769,-0.0615384615384615,-0.0461538461538462,
-0.0307692307692308,-0.0153846153846154,0.),.UNSPECIFIED.)
CURVE()
GEOMETRIC_REPRESENTATION_ITEM()
RATIONAL_B_SPLINE_CURVE((1.,1.,1.,1.,1.,1.,1.,1.,1.,1.,1.,1.,1.,1.,1.,1.,
1.,1.,1.,1.,1.,1.,1.,1.,1.,1.,1.,1.,1.,1.,1.,1.,1.,1.,1.,1.,1.,1.,1.,1.,
1.,1.,1.,1.,1.,1.,1.,1.,1.,1.,1.,1.,1.,1.,1.,1.,1.,1.,1.,1.,1.,1.,1.,1.,
1.,1.,1.,1.,1.,1.))
REPRESENTATION_ITEM('')
);
#122=(
BOUNDED_CURVE()
B_SPLINE_CURVE(5,(#30613,#30614,#30615,#30616,#30617,#30618,#30619,#30620,
#30621,#30622,#30623,#30624,#30625,#30626,#30627,#30628,#30629,#30630,#30631,
#30632,#30633,#30634,#30635,#30636,#30637,#30638,#30639,#30640,#30641,#30642,
#30643,#30644,#30645,#30646,#30647,#30648,#30649,#30650,#30651,#30652,#30653,
#30654,#30655,#30656,#30657,#30658,#30659,#30660,#30661,#30662,#30663,#30664,
#30665,#30666,#30667,#30668,#30669,#30670,#30671,#30672,#30673,#30674,#30675,
#30676,#30677,#30678,#30679,#30680,#30681,#30682),.UNSPECIFIED.,.F.,.F.)
B_SPLINE_CURVE_WITH_KNOTS((6,1,1,1,1,1,1,1,1,1,1,1,1,1,1,1,1,1,1,1,1,1,
1,1,1,1,1,1,1,1,1,1,1,1,1,1,1,1,1,1,1,1,1,1,1,1,1,1,1,1,1,1,1,1,1,1,1,1,
1,1,1,1,1,1,1,6),(-1.,-0.984615384615383,-0.969230769230768,-0.953846153846152,
-0.938461538461537,-0.923076923076922,-0.907692307692306,-0.892307692307691,
-0.876923076923076,-0.86153846153846,-0.846153846153845,-0.83076923076923,
-0.815384615384614,-0.799999999999999,-0.784615384615384,-0.769230769230768,
-0.753846153846153,-0.738461538461538,-0.723076923076922,-0.707692307692307,
-0.692307692307692,-0.676923076923076,-0.661538461538461,-0.646153846153846,
-0.63076923076923,-0.615384615384615,-0.6,-0.584615384615384,-0.569230769230769,
-0.553846153846154,-0.538461538461538,-0.523076923076923,-0.507692307692308,
-0.492307692307692,-0.476923076923077,-0.461538461538462,-0.446153846153846,
-0.430769230769231,-0.415384615384615,-0.4,-0.384615384615385,-0.369230769230769,
-0.353846153846154,-0.338461538461538,-0.323076923076923,-0.307692307692308,
-0.292307692307692,-0.276923076923077,-0.261538461538462,-0.246153846153846,
-0.230769230769231,-0.215384615384615,-0.2,-0.184615384615385,-0.169230769230769,
-0.153846153846154,-0.138461538461538,-0.123076923076923,-0.107692307692308,
-0.0923076923076923,-0.0769230769230769,-0.0615384615384615,-0.0461538461538462,
-0.0307692307692308,-0.0153846153846154,0.),.UNSPECIFIED.)
CURVE()
GEOMETRIC_REPRESENTATION_ITEM()
RATIONAL_B_SPLINE_CURVE((1.,1.,1.,1.,1.,1.,1.,1.,1.,1.,1.,1.,1.,1.,1.,1.,
1.,1.,1.,1.,1.,1.,1.,1.,1.,1.,1.,1.,1.,1.,1.,1.,1.,1.,1.,1.,1.,1.,1.,1.,
1.,1.,1.,1.,1.,1.,1.,1.,1.,1.,1.,1.,1.,1.,1.,1.,1.,1.,1.,1.,1.,1.,1.,1.,
1.,1.,1.,1.,1.,1.))
REPRESENTATION_ITEM('')
);
#123=(
BOUNDED_CURVE()
B_SPLINE_CURVE(5,(#30829,#30830,#30831,#30832,#30833,#30834,#30835,#30836,
#30837,#30838,#30839,#30840,#30841,#30842,#30843,#30844,#30845,#30846,#30847,
#30848,#30849,#30850,#30851,#30852,#30853,#30854,#30855,#30856,#30857,#30858,
#30859,#30860,#30861,#30862,#30863,#30864,#30865,#30866,#30867,#30868,#30869,
#30870,#30871,#30872,#30873,#30874,#30875,#30876,#30877,#30878,#30879,#30880,
#30881,#30882,#30883,#30884,#30885,#30886,#30887,#30888,#30889,#30890,#30891,
#30892,#30893,#30894,#30895,#30896,#30897,#30898),.UNSPECIFIED.,.F.,.F.)
B_SPLINE_CURVE_WITH_KNOTS((6,1,1,1,1,1,1,1,1,1,1,1,1,1,1,1,1,1,1,1,1,1,
1,1,1,1,1,1,1,1,1,1,1,1,1,1,1,1,1,1,1,1,1,1,1,1,1,1,1,1,1,1,1,1,1,1,1,1,
1,1,1,1,1,1,1,6),(-1.,-0.984615384615383,-0.969230769230768,-0.953846153846152,
-0.938461538461537,-0.923076923076922,-0.907692307692306,-0.892307692307691,
-0.876923076923076,-0.86153846153846,-0.846153846153845,-0.83076923076923,
-0.815384615384614,-0.799999999999999,-0.784615384615384,-0.769230769230768,
-0.753846153846153,-0.738461538461538,-0.723076923076922,-0.707692307692307,
-0.692307692307692,-0.676923076923076,-0.661538461538461,-0.646153846153846,
-0.63076923076923,-0.615384615384615,-0.6,-0.584615384615384,-0.569230769230769,
-0.553846153846154,-0.538461538461538,-0.523076923076923,-0.507692307692308,
-0.492307692307692,-0.476923076923077,-0.461538461538462,-0.446153846153846,
-0.430769230769231,-0.415384615384615,-0.4,-0.384615384615385,-0.369230769230769,
-0.353846153846154,-0.338461538461538,-0.323076923076923,-0.307692307692308,
-0.292307692307692,-0.276923076923077,-0.261538461538462,-0.246153846153846,
-0.230769230769231,-0.215384615384615,-0.2,-0.184615384615385,-0.169230769230769,
-0.153846153846154,-0.138461538461538,-0.123076923076923,-0.107692307692308,
-0.0923076923076923,-0.0769230769230769,-0.0615384615384615,-0.0461538461538462,
-0.0307692307692308,-0.0153846153846154,0.),.UNSPECIFIED.)
CURVE()
GEOMETRIC_REPRESENTATION_ITEM()
RATIONAL_B_SPLINE_CURVE((1.,1.,1.,1.,1.,1.,1.,1.,1.,1.,1.,1.,1.,1.,1.,1.,
1.,1.,1.,1.,1.,1.,1.,1.,1.,1.,1.,1.,1.,1.,1.,1.,1.,1.,1.,1.,1.,1.,1.,1.,
1.,1.,1.,1.,1.,1.,1.,1.,1.,1.,1.,1.,1.,1.,1.,1.,1.,1.,1.,1.,1.,1.,1.,1.,
1.,1.,1.,1.,1.,1.))
REPRESENTATION_ITEM('')
);
#124=(
BOUNDED_CURVE()
B_SPLINE_CURVE(5,(#31045,#31046,#31047,#31048,#31049,#31050,#31051,#31052,
#31053,#31054,#31055,#31056,#31057,#31058,#31059,#31060,#31061,#31062,#31063,
#31064,#31065,#31066,#31067,#31068,#31069,#31070,#31071,#31072,#31073,#31074,
#31075,#31076,#31077,#31078,#31079,#31080,#31081,#31082,#31083,#31084,#31085,
#31086,#31087,#31088,#31089,#31090,#31091,#31092,#31093,#31094,#31095,#31096,
#31097,#31098,#31099,#31100,#31101,#31102,#31103,#31104,#31105,#31106,#31107,
#31108,#31109,#31110,#31111,#31112,#31113,#31114),.UNSPECIFIED.,.F.,.F.)
B_SPLINE_CURVE_WITH_KNOTS((6,1,1,1,1,1,1,1,1,1,1,1,1,1,1,1,1,1,1,1,1,1,
1,1,1,1,1,1,1,1,1,1,1,1,1,1,1,1,1,1,1,1,1,1,1,1,1,1,1,1,1,1,1,1,1,1,1,1,
1,1,1,1,1,1,1,6),(-1.,-0.984615384615383,-0.969230769230768,-0.953846153846152,
-0.938461538461537,-0.923076923076922,-0.907692307692306,-0.892307692307691,
-0.876923076923076,-0.86153846153846,-0.846153846153845,-0.83076923076923,
-0.815384615384614,-0.799999999999999,-0.784615384615384,-0.769230769230768,
-0.753846153846153,-0.738461538461538,-0.723076923076922,-0.707692307692307,
-0.692307692307692,-0.676923076923076,-0.661538461538461,-0.646153846153846,
-0.63076923076923,-0.615384615384615,-0.6,-0.584615384615384,-0.569230769230769,
-0.553846153846154,-0.538461538461538,-0.523076923076923,-0.507692307692308,
-0.492307692307692,-0.476923076923077,-0.461538461538462,-0.446153846153846,
-0.430769230769231,-0.415384615384615,-0.4,-0.384615384615385,-0.369230769230769,
-0.353846153846154,-0.338461538461538,-0.323076923076923,-0.307692307692308,
-0.292307692307692,-0.276923076923077,-0.261538461538462,-0.246153846153846,
-0.230769230769231,-0.215384615384615,-0.2,-0.184615384615385,-0.169230769230769,
-0.153846153846154,-0.138461538461538,-0.123076923076923,-0.107692307692308,
-0.0923076923076923,-0.0769230769230769,-0.0615384615384615,-0.0461538461538462,
-0.0307692307692308,-0.0153846153846154,0.),.UNSPECIFIED.)
CURVE()
GEOMETRIC_REPRESENTATION_ITEM()
RATIONAL_B_SPLINE_CURVE((1.,1.,1.,1.,1.,1.,1.,1.,1.,1.,1.,1.,1.,1.,1.,1.,
1.,1.,1.,1.,1.,1.,1.,1.,1.,1.,1.,1.,1.,1.,1.,1.,1.,1.,1.,1.,1.,1.,1.,1.,
1.,1.,1.,1.,1.,1.,1.,1.,1.,1.,1.,1.,1.,1.,1.,1.,1.,1.,1.,1.,1.,1.,1.,1.,
1.,1.,1.,1.,1.,1.))
REPRESENTATION_ITEM('')
);
#125=(
BOUNDED_CURVE()
B_SPLINE_CURVE(5,(#31261,#31262,#31263,#31264,#31265,#31266,#31267,#31268,
#31269,#31270,#31271,#31272,#31273,#31274,#31275,#31276,#31277,#31278,#31279,
#31280,#31281,#31282,#31283,#31284,#31285,#31286,#31287,#31288,#31289,#31290,
#31291,#31292,#31293,#31294,#31295,#31296,#31297,#31298,#31299,#31300,#31301,
#31302,#31303,#31304,#31305,#31306,#31307,#31308,#31309,#31310,#31311,#31312,
#31313,#31314,#31315,#31316,#31317,#31318,#31319,#31320,#31321,#31322,#31323,
#31324,#31325,#31326,#31327,#31328,#31329,#31330),.UNSPECIFIED.,.F.,.F.)
B_SPLINE_CURVE_WITH_KNOTS((6,1,1,1,1,1,1,1,1,1,1,1,1,1,1,1,1,1,1,1,1,1,
1,1,1,1,1,1,1,1,1,1,1,1,1,1,1,1,1,1,1,1,1,1,1,1,1,1,1,1,1,1,1,1,1,1,1,1,
1,1,1,1,1,1,1,6),(-1.,-0.984615384615383,-0.969230769230768,-0.953846153846152,
-0.938461538461537,-0.923076923076922,-0.907692307692306,-0.892307692307691,
-0.876923076923076,-0.86153846153846,-0.846153846153845,-0.83076923076923,
-0.815384615384614,-0.799999999999999,-0.784615384615384,-0.769230769230768,
-0.753846153846153,-0.738461538461538,-0.723076923076922,-0.707692307692307,
-0.692307692307692,-0.676923076923076,-0.661538461538461,-0.646153846153846,
-0.63076923076923,-0.615384615384615,-0.6,-0.584615384615384,-0.569230769230769,
-0.553846153846154,-0.538461538461538,-0.523076923076923,-0.507692307692308,
-0.492307692307692,-0.476923076923077,-0.461538461538462,-0.446153846153846,
-0.430769230769231,-0.415384615384615,-0.4,-0.384615384615385,-0.369230769230769,
-0.353846153846154,-0.338461538461538,-0.323076923076923,-0.307692307692308,
-0.292307692307692,-0.276923076923077,-0.261538461538462,-0.246153846153846,
-0.230769230769231,-0.215384615384615,-0.2,-0.184615384615385,-0.169230769230769,
-0.153846153846154,-0.138461538461538,-0.123076923076923,-0.107692307692308,
-0.0923076923076923,-0.0769230769230769,-0.0615384615384615,-0.0461538461538462,
-0.0307692307692308,-0.0153846153846154,0.),.UNSPECIFIED.)
CURVE()
GEOMETRIC_REPRESENTATION_ITEM()
RATIONAL_B_SPLINE_CURVE((1.,1.,1.,1.,1.,1.,1.,1.,1.,1.,1.,1.,1.,1.,1.,1.,
1.,1.,1.,1.,1.,1.,1.,1.,1.,1.,1.,1.,1.,1.,1.,1.,1.,1.,1.,1.,1.,1.,1.,1.,
1.,1.,1.,1.,1.,1.,1.,1.,1.,1.,1.,1.,1.,1.,1.,1.,1.,1.,1.,1.,1.,1.,1.,1.,
1.,1.,1.,1.,1.,1.))
REPRESENTATION_ITEM('')
);
#126=(
BOUNDED_CURVE()
B_SPLINE_CURVE(5,(#31477,#31478,#31479,#31480,#31481,#31482,#31483,#31484,
#31485,#31486,#31487,#31488,#31489,#31490,#31491,#31492,#31493,#31494,#31495,
#31496,#31497,#31498,#31499,#31500,#31501,#31502,#31503,#31504,#31505,#31506,
#31507,#31508,#31509,#31510,#31511,#31512,#31513,#31514,#31515,#31516,#31517,
#31518,#31519,#31520,#31521,#31522,#31523,#31524,#31525,#31526,#31527,#31528,
#31529,#31530,#31531,#31532,#31533,#31534,#31535,#31536,#31537,#31538,#31539,
#31540,#31541,#31542,#31543,#31544,#31545,#31546),.UNSPECIFIED.,.F.,.F.)
B_SPLINE_CURVE_WITH_KNOTS((6,1,1,1,1,1,1,1,1,1,1,1,1,1,1,1,1,1,1,1,1,1,
1,1,1,1,1,1,1,1,1,1,1,1,1,1,1,1,1,1,1,1,1,1,1,1,1,1,1,1,1,1,1,1,1,1,1,1,
1,1,1,1,1,1,1,6),(-1.,-0.984615384615383,-0.969230769230768,-0.953846153846152,
-0.938461538461537,-0.923076923076922,-0.907692307692306,-0.892307692307691,
-0.876923076923076,-0.86153846153846,-0.846153846153845,-0.83076923076923,
-0.815384615384614,-0.799999999999999,-0.784615384615384,-0.769230769230768,
-0.753846153846153,-0.738461538461538,-0.723076923076922,-0.707692307692307,
-0.692307692307692,-0.676923076923076,-0.661538461538461,-0.646153846153846,
-0.63076923076923,-0.615384615384615,-0.6,-0.584615384615384,-0.569230769230769,
-0.553846153846154,-0.538461538461538,-0.523076923076923,-0.507692307692308,
-0.492307692307692,-0.476923076923077,-0.461538461538462,-0.446153846153846,
-0.430769230769231,-0.415384615384615,-0.4,-0.384615384615385,-0.369230769230769,
-0.353846153846154,-0.338461538461538,-0.323076923076923,-0.307692307692308,
-0.292307692307692,-0.276923076923077,-0.261538461538462,-0.246153846153846,
-0.230769230769231,-0.215384615384615,-0.2,-0.184615384615385,-0.169230769230769,
-0.153846153846154,-0.138461538461538,-0.123076923076923,-0.107692307692308,
-0.0923076923076923,-0.0769230769230769,-0.0615384615384615,-0.0461538461538462,
-0.0307692307692308,-0.0153846153846154,0.),.UNSPECIFIED.)
CURVE()
GEOMETRIC_REPRESENTATION_ITEM()
RATIONAL_B_SPLINE_CURVE((1.,1.,1.,1.,1.,1.,1.,1.,1.,1.,1.,1.,1.,1.,1.,1.,
1.,1.,1.,1.,1.,1.,1.,1.,1.,1.,1.,1.,1.,1.,1.,1.,1.,1.,1.,1.,1.,1.,1.,1.,
1.,1.,1.,1.,1.,1.,1.,1.,1.,1.,1.,1.,1.,1.,1.,1.,1.,1.,1.,1.,1.,1.,1.,1.,
1.,1.,1.,1.,1.,1.))
REPRESENTATION_ITEM('')
);
#127=(
BOUNDED_CURVE()
B_SPLINE_CURVE(5,(#31693,#31694,#31695,#31696,#31697,#31698,#31699,#31700,
#31701,#31702,#31703,#31704,#31705,#31706,#31707,#31708,#31709,#31710,#31711,
#31712,#31713,#31714,#31715,#31716,#31717,#31718,#31719,#31720,#31721,#31722,
#31723,#31724,#31725,#31726,#31727,#31728,#31729,#31730,#31731,#31732,#31733,
#31734,#31735,#31736,#31737,#31738,#31739,#31740,#31741,#31742,#31743,#31744,
#31745,#31746,#31747,#31748,#31749,#31750,#31751,#31752,#31753,#31754,#31755,
#31756,#31757,#31758,#31759,#31760,#31761,#31762),.UNSPECIFIED.,.F.,.F.)
B_SPLINE_CURVE_WITH_KNOTS((6,1,1,1,1,1,1,1,1,1,1,1,1,1,1,1,1,1,1,1,1,1,
1,1,1,1,1,1,1,1,1,1,1,1,1,1,1,1,1,1,1,1,1,1,1,1,1,1,1,1,1,1,1,1,1,1,1,1,
1,1,1,1,1,1,1,6),(-1.,-0.984615384615383,-0.969230769230768,-0.953846153846152,
-0.938461538461537,-0.923076923076922,-0.907692307692306,-0.892307692307691,
-0.876923076923076,-0.86153846153846,-0.846153846153845,-0.83076923076923,
-0.815384615384614,-0.799999999999999,-0.784615384615384,-0.769230769230768,
-0.753846153846153,-0.738461538461538,-0.723076923076922,-0.707692307692307,
-0.692307692307692,-0.676923076923076,-0.661538461538461,-0.646153846153846,
-0.63076923076923,-0.615384615384615,-0.6,-0.584615384615384,-0.569230769230769,
-0.553846153846154,-0.538461538461538,-0.523076923076923,-0.507692307692308,
-0.492307692307692,-0.476923076923077,-0.461538461538462,-0.446153846153846,
-0.430769230769231,-0.415384615384615,-0.4,-0.384615384615385,-0.369230769230769,
-0.353846153846154,-0.338461538461538,-0.323076923076923,-0.307692307692308,
-0.292307692307692,-0.276923076923077,-0.261538461538462,-0.246153846153846,
-0.230769230769231,-0.215384615384615,-0.2,-0.184615384615385,-0.169230769230769,
-0.153846153846154,-0.138461538461538,-0.123076923076923,-0.107692307692308,
-0.0923076923076923,-0.0769230769230769,-0.0615384615384615,-0.0461538461538462,
-0.0307692307692308,-0.0153846153846154,0.),.UNSPECIFIED.)
CURVE()
GEOMETRIC_REPRESENTATION_ITEM()
RATIONAL_B_SPLINE_CURVE((1.,1.,1.,1.,1.,1.,1.,1.,1.,1.,1.,1.,1.,1.,1.,1.,
1.,1.,1.,1.,1.,1.,1.,1.,1.,1.,1.,1.,1.,1.,1.,1.,1.,1.,1.,1.,1.,1.,1.,1.,
1.,1.,1.,1.,1.,1.,1.,1.,1.,1.,1.,1.,1.,1.,1.,1.,1.,1.,1.,1.,1.,1.,1.,1.,
1.,1.,1.,1.,1.,1.))
REPRESENTATION_ITEM('')
);
#128=(
BOUNDED_CURVE()
B_SPLINE_CURVE(5,(#31909,#31910,#31911,#31912,#31913,#31914,#31915,#31916,
#31917,#31918,#31919,#31920,#31921,#31922,#31923,#31924,#31925,#31926,#31927,
#31928,#31929,#31930,#31931,#31932,#31933,#31934,#31935,#31936,#31937,#31938,
#31939,#31940,#31941,#31942,#31943,#31944,#31945,#31946,#31947,#31948,#31949,
#31950,#31951,#31952,#31953,#31954,#31955,#31956,#31957,#31958,#31959,#31960,
#31961,#31962,#31963,#31964,#31965,#31966,#31967,#31968,#31969,#31970,#31971,
#31972,#31973,#31974,#31975,#31976,#31977,#31978),.UNSPECIFIED.,.F.,.F.)
B_SPLINE_CURVE_WITH_KNOTS((6,1,1,1,1,1,1,1,1,1,1,1,1,1,1,1,1,1,1,1,1,1,
1,1,1,1,1,1,1,1,1,1,1,1,1,1,1,1,1,1,1,1,1,1,1,1,1,1,1,1,1,1,1,1,1,1,1,1,
1,1,1,1,1,1,1,6),(-1.,-0.984615384615383,-0.969230769230768,-0.953846153846152,
-0.938461538461537,-0.923076923076922,-0.907692307692306,-0.892307692307691,
-0.876923076923076,-0.86153846153846,-0.846153846153845,-0.83076923076923,
-0.815384615384614,-0.799999999999999,-0.784615384615384,-0.769230769230768,
-0.753846153846153,-0.738461538461538,-0.723076923076922,-0.707692307692307,
-0.692307692307692,-0.676923076923076,-0.661538461538461,-0.646153846153846,
-0.63076923076923,-0.615384615384615,-0.6,-0.584615384615384,-0.569230769230769,
-0.553846153846154,-0.538461538461538,-0.523076923076923,-0.507692307692308,
-0.492307692307692,-0.476923076923077,-0.461538461538462,-0.446153846153846,
-0.430769230769231,-0.415384615384615,-0.4,-0.384615384615385,-0.369230769230769,
-0.353846153846154,-0.338461538461538,-0.323076923076923,-0.307692307692308,
-0.292307692307692,-0.276923076923077,-0.261538461538462,-0.246153846153846,
-0.230769230769231,-0.215384615384615,-0.2,-0.184615384615385,-0.169230769230769,
-0.153846153846154,-0.138461538461538,-0.123076923076923,-0.107692307692308,
-0.0923076923076923,-0.0769230769230769,-0.0615384615384615,-0.0461538461538462,
-0.0307692307692308,-0.0153846153846154,0.),.UNSPECIFIED.)
CURVE()
GEOMETRIC_REPRESENTATION_ITEM()
RATIONAL_B_SPLINE_CURVE((1.,1.,1.,1.,1.,1.,1.,1.,1.,1.,1.,1.,1.,1.,1.,1.,
1.,1.,1.,1.,1.,1.,1.,1.,1.,1.,1.,1.,1.,1.,1.,1.,1.,1.,1.,1.,1.,1.,1.,1.,
1.,1.,1.,1.,1.,1.,1.,1.,1.,1.,1.,1.,1.,1.,1.,1.,1.,1.,1.,1.,1.,1.,1.,1.,
1.,1.,1.,1.,1.,1.))
REPRESENTATION_ITEM('')
);
#129=(
BOUNDED_CURVE()
B_SPLINE_CURVE(5,(#32125,#32126,#32127,#32128,#32129,#32130,#32131,#32132,
#32133,#32134,#32135,#32136,#32137,#32138,#32139,#32140,#32141,#32142,#32143,
#32144,#32145,#32146,#32147,#32148,#32149,#32150,#32151,#32152,#32153,#32154,
#32155,#32156,#32157,#32158,#32159,#32160,#32161,#32162,#32163,#32164,#32165,
#32166,#32167,#32168,#32169,#32170,#32171,#32172,#32173,#32174,#32175,#32176,
#32177,#32178,#32179,#32180,#32181,#32182,#32183,#32184,#32185,#32186,#32187,
#32188,#32189,#32190,#32191,#32192,#32193,#32194),.UNSPECIFIED.,.F.,.F.)
B_SPLINE_CURVE_WITH_KNOTS((6,1,1,1,1,1,1,1,1,1,1,1,1,1,1,1,1,1,1,1,1,1,
1,1,1,1,1,1,1,1,1,1,1,1,1,1,1,1,1,1,1,1,1,1,1,1,1,1,1,1,1,1,1,1,1,1,1,1,
1,1,1,1,1,1,1,6),(-1.,-0.984615384615383,-0.969230769230768,-0.953846153846152,
-0.938461538461537,-0.923076923076922,-0.907692307692306,-0.892307692307691,
-0.876923076923076,-0.86153846153846,-0.846153846153845,-0.83076923076923,
-0.815384615384614,-0.799999999999999,-0.784615384615384,-0.769230769230768,
-0.753846153846153,-0.738461538461538,-0.723076923076922,-0.707692307692307,
-0.692307692307692,-0.676923076923076,-0.661538461538461,-0.646153846153846,
-0.63076923076923,-0.615384615384615,-0.6,-0.584615384615384,-0.569230769230769,
-0.553846153846154,-0.538461538461538,-0.523076923076923,-0.507692307692308,
-0.492307692307692,-0.476923076923077,-0.461538461538462,-0.446153846153846,
-0.430769230769231,-0.415384615384615,-0.4,-0.384615384615385,-0.369230769230769,
-0.353846153846154,-0.338461538461538,-0.323076923076923,-0.307692307692308,
-0.292307692307692,-0.276923076923077,-0.261538461538462,-0.246153846153846,
-0.230769230769231,-0.215384615384615,-0.2,-0.184615384615385,-0.169230769230769,
-0.153846153846154,-0.138461538461538,-0.123076923076923,-0.107692307692308,
-0.0923076923076923,-0.0769230769230769,-0.0615384615384615,-0.0461538461538462,
-0.0307692307692308,-0.0153846153846154,0.),.UNSPECIFIED.)
CURVE()
GEOMETRIC_REPRESENTATION_ITEM()
RATIONAL_B_SPLINE_CURVE((1.,1.,1.,1.,1.,1.,1.,1.,1.,1.,1.,1.,1.,1.,1.,1.,
1.,1.,1.,1.,1.,1.,1.,1.,1.,1.,1.,1.,1.,1.,1.,1.,1.,1.,1.,1.,1.,1.,1.,1.,
1.,1.,1.,1.,1.,1.,1.,1.,1.,1.,1.,1.,1.,1.,1.,1.,1.,1.,1.,1.,1.,1.,1.,1.,
1.,1.,1.,1.,1.,1.))
REPRESENTATION_ITEM('')
);
#130=(
BOUNDED_CURVE()
B_SPLINE_CURVE(5,(#32341,#32342,#32343,#32344,#32345,#32346,#32347,#32348,
#32349,#32350,#32351,#32352,#32353,#32354,#32355,#32356,#32357,#32358,#32359,
#32360,#32361,#32362,#32363,#32364,#32365,#32366,#32367,#32368,#32369,#32370,
#32371,#32372,#32373,#32374,#32375,#32376,#32377,#32378,#32379,#32380,#32381,
#32382,#32383,#32384,#32385,#32386,#32387,#32388,#32389,#32390,#32391,#32392,
#32393,#32394,#32395,#32396,#32397,#32398,#32399,#32400,#32401,#32402,#32403,
#32404,#32405,#32406,#32407,#32408,#32409,#32410),.UNSPECIFIED.,.F.,.F.)
B_SPLINE_CURVE_WITH_KNOTS((6,1,1,1,1,1,1,1,1,1,1,1,1,1,1,1,1,1,1,1,1,1,
1,1,1,1,1,1,1,1,1,1,1,1,1,1,1,1,1,1,1,1,1,1,1,1,1,1,1,1,1,1,1,1,1,1,1,1,
1,1,1,1,1,1,1,6),(-1.,-0.984615384615383,-0.969230769230768,-0.953846153846152,
-0.938461538461537,-0.923076923076922,-0.907692307692306,-0.892307692307691,
-0.876923076923076,-0.86153846153846,-0.846153846153845,-0.83076923076923,
-0.815384615384614,-0.799999999999999,-0.784615384615384,-0.769230769230768,
-0.753846153846153,-0.738461538461538,-0.723076923076922,-0.707692307692307,
-0.692307692307692,-0.676923076923076,-0.661538461538461,-0.646153846153846,
-0.63076923076923,-0.615384615384615,-0.6,-0.584615384615384,-0.569230769230769,
-0.553846153846154,-0.538461538461538,-0.523076923076923,-0.507692307692308,
-0.492307692307692,-0.476923076923077,-0.461538461538462,-0.446153846153846,
-0.430769230769231,-0.415384615384615,-0.4,-0.384615384615385,-0.369230769230769,
-0.353846153846154,-0.338461538461538,-0.323076923076923,-0.307692307692308,
-0.292307692307692,-0.276923076923077,-0.261538461538462,-0.246153846153846,
-0.230769230769231,-0.215384615384615,-0.2,-0.184615384615385,-0.169230769230769,
-0.153846153846154,-0.138461538461538,-0.123076923076923,-0.107692307692308,
-0.0923076923076923,-0.0769230769230769,-0.0615384615384615,-0.0461538461538462,
-0.0307692307692308,-0.0153846153846154,0.),.UNSPECIFIED.)
CURVE()
GEOMETRIC_REPRESENTATION_ITEM()
RATIONAL_B_SPLINE_CURVE((1.,1.,1.,1.,1.,1.,1.,1.,1.,1.,1.,1.,1.,1.,1.,1.,
1.,1.,1.,1.,1.,1.,1.,1.,1.,1.,1.,1.,1.,1.,1.,1.,1.,1.,1.,1.,1.,1.,1.,1.,
1.,1.,1.,1.,1.,1.,1.,1.,1.,1.,1.,1.,1.,1.,1.,1.,1.,1.,1.,1.,1.,1.,1.,1.,
1.,1.,1.,1.,1.,1.))
REPRESENTATION_ITEM('')
);
#539=SHAPE_REPRESENTATION_RELATIONSHIP('SRR','None',#32971,#581);
#581=ADVANCED_BREP_SHAPE_REPRESENTATION('',(#677),#32745);
#630=STYLED_ITEM('',(#33256),#677);
#677=MANIFOLD_SOLID_BREP('Body1',#12529);
#840=FACE_BOUND('',#2689,.T.);
#841=FACE_BOUND('',#2693,.T.);
#842=FACE_BOUND('',#2774,.T.);
#1241=PLANE('',#13924);
#1242=PLANE('',#13925);
#1243=PLANE('',#13926);
#1244=PLANE('',#13927);
#1245=PLANE('',#13954);
#1246=PLANE('',#13955);
#1247=PLANE('',#13958);
#1248=PLANE('',#13961);
#1249=PLANE('',#13964);
#1250=PLANE('',#13967);
#1251=PLANE('',#13970);
#1252=PLANE('',#13973);
#1253=PLANE('',#13976);
#1254=PLANE('',#13979);
#1255=PLANE('',#13982);
#1256=PLANE('',#13985);
#1257=PLANE('',#13988);
#1258=PLANE('',#13991);
#1259=PLANE('',#13994);
#1260=PLANE('',#13997);
#1261=PLANE('',#14000);
#1262=PLANE('',#14003);
#1263=PLANE('',#14006);
#1264=PLANE('',#14009);
#1265=PLANE('',#14012);
#1266=PLANE('',#14013);
#1844=FACE_OUTER_BOUND('',#2685,.T.);
#1845=FACE_OUTER_BOUND('',#2686,.T.);
#1846=FACE_OUTER_BOUND('',#2687,.T.);
#1847=FACE_OUTER_BOUND('',#2688,.T.);
#1848=FACE_OUTER_BOUND('',#2690,.T.);
#1849=FACE_OUTER_BOUND('',#2691,.T.);
#1850=FACE_OUTER_BOUND('',#2692,.T.);
#1851=FACE_OUTER_BOUND('',#2694,.T.);
#1852=FACE_OUTER_BOUND('',#2695,.T.);
#1853=FACE_OUTER_BOUND('',#2696,.T.);
#1854=FACE_OUTER_BOUND('',#2697,.T.);
#1855=FACE_OUTER_BOUND('',#2698,.T.);
#1856=FACE_OUTER_BOUND('',#2699,.T.);
#1857=FACE_OUTER_BOUND('',#2700,.T.);
#1858=FACE_OUTER_BOUND('',#2701,.T.);
#1859=FACE_OUTER_BOUND('',#2702,.T.);
#1860=FACE_OUTER_BOUND('',#2703,.T.);
#1861=FACE_OUTER_BOUND('',#2704,.T.);
#1862=FACE_OUTER_BOUND('',#2705,.T.);
#1863=FACE_OUTER_BOUND('',#2706,.T.);
#1864=FACE_OUTER_BOUND('',#2707,.T.);
#1865=FACE_OUTER_BOUND('',#2708,.T.);
#1866=FACE_OUTER_BOUND('',#2709,.T.);
#1867=FACE_OUTER_BOUND('',#2710,.T.);
#1868=FACE_OUTER_BOUND('',#2711,.T.);
#1869=FACE_OUTER_BOUND('',#2712,.T.);
#1870=FACE_OUTER_BOUND('',#2713,.T.);
#1871=FACE_OUTER_BOUND('',#2714,.T.);
#1872=FACE_OUTER_BOUND('',#2715,.T.);
#1873=FACE_OUTER_BOUND('',#2716,.T.);
#1874=FACE_OUTER_BOUND('',#2717,.T.);
#1875=FACE_OUTER_BOUND('',#2718,.T.);
#1876=FACE_OUTER_BOUND('',#2719,.T.);
#1877=FACE_OUTER_BOUND('',#2720,.T.);
#1878=FACE_OUTER_BOUND('',#2721,.T.);
#1879=FACE_OUTER_BOUND('',#2722,.T.);
#1880=FACE_OUTER_BOUND('',#2723,.T.);
#1881=FACE_OUTER_BOUND('',#2724,.T.);
#1882=FACE_OUTER_BOUND('',#2725,.T.);
#1883=FACE_OUTER_BOUND('',#2726,.T.);
#1884=FACE_OUTER_BOUND('',#2727,.T.);
#1885=FACE_OUTER_BOUND('',#2728,.T.);
#1886=FACE_OUTER_BOUND('',#2729,.T.);
#1887=FACE_OUTER_BOUND('',#2730,.T.);
#1888=FACE_OUTER_BOUND('',#2731,.T.);
#1889=FACE_OUTER_BOUND('',#2732,.T.);
#1890=FACE_OUTER_BOUND('',#2733,.T.);
#1891=FACE_OUTER_BOUND('',#2734,.T.);
#1892=FACE_OUTER_BOUND('',#2735,.T.);
#1893=FACE_OUTER_BOUND('',#2736,.T.);
#1894=FACE_OUTER_BOUND('',#2737,.T.);
#1895=FACE_OUTER_BOUND('',#2738,.T.);
#1896=FACE_OUTER_BOUND('',#2739,.T.);
#1897=FACE_OUTER_BOUND('',#2740,.T.);
#1898=FACE_OUTER_BOUND('',#2741,.T.);
#1899=FACE_OUTER_BOUND('',#2742,.T.);
#1900=FACE_OUTER_BOUND('',#2743,.T.);
#1901=FACE_OUTER_BOUND('',#2744,.T.);
#1902=FACE_OUTER_BOUND('',#2745,.T.);
#1903=FACE_OUTER_BOUND('',#2746,.T.);
#1904=FACE_OUTER_BOUND('',#2747,.T.);
#1905=FACE_OUTER_BOUND('',#2748,.T.);
#1906=FACE_OUTER_BOUND('',#2749,.T.);
#1907=FACE_OUTER_BOUND('',#2750,.T.);
#1908=FACE_OUTER_BOUND('',#2751,.T.);
#1909=FACE_OUTER_BOUND('',#2752,.T.);
#1910=FACE_OUTER_BOUND('',#2753,.T.);
#1911=FACE_OUTER_BOUND('',#2754,.T.);
#1912=FACE_OUTER_BOUND('',#2755,.T.);
#1913=FACE_OUTER_BOUND('',#2756,.T.);
#1914=FACE_OUTER_BOUND('',#2757,.T.);
#1915=FACE_OUTER_BOUND('',#2758,.T.);
#1916=FACE_OUTER_BOUND('',#2759,.T.);
#1917=FACE_OUTER_BOUND('',#2760,.T.);
#1918=FACE_OUTER_BOUND('',#2761,.T.);
#1919=FACE_OUTER_BOUND('',#2762,.T.);
#1920=FACE_OUTER_BOUND('',#2763,.T.);
#1921=FACE_OUTER_BOUND('',#2764,.T.);
#1922=FACE_OUTER_BOUND('',#2765,.T.);
#1923=FACE_OUTER_BOUND('',#2766,.T.);
#1924=FACE_OUTER_BOUND('',#2767,.T.);
#1925=FACE_OUTER_BOUND('',#2768,.T.);
#1926=FACE_OUTER_BOUND('',#2769,.T.);
#1927=FACE_OUTER_BOUND('',#2770,.T.);
#1928=FACE_OUTER_BOUND('',#2771,.T.);
#1929=FACE_OUTER_BOUND('',#2772,.T.);
#1930=FACE_OUTER_BOUND('',#2773,.T.);
#1931=FACE_OUTER_BOUND('',#2775,.T.);
#2685=EDGE_LOOP('',(#10980,#10981,#10982,#10983));
#2686=EDGE_LOOP('',(#10984,#10985,#10986,#10987));
#2687=EDGE_LOOP('',(#10988,#10989,#10990,#10991));
#2688=EDGE_LOOP('',(#10992,#10993,#10994,#10995,#10996,#10997,#10998,#10999,
#11000,#11001,#11002,#11003,#11004,#11005,#11006,#11007,#11008,#11009,#11010,
#11011,#11012,#11013,#11014,#11015,#11016,#11017,#11018,#11019,#11020,#11021,
#11022,#11023,#11024,#11025,#11026,#11027,#11028,#11029,#11030,#11031,#11032,
#11033,#11034,#11035,#11036,#11037,#11038,#11039,#11040,#11041,#11042,#11043,
#11044,#11045,#11046,#11047,#11048,#11049,#11050,#11051,#11052,#11053,#11054,
#11055,#11056,#11057,#11058,#11059,#11060,#11061,#11062,#11063,#11064,#11065,
#11066,#11067,#11068,#11069,#11070,#11071));
#2689=EDGE_LOOP('',(#11072,#11073,#11074,#11075));
#2690=EDGE_LOOP('',(#11076,#11077,#11078,#11079));
#2691=EDGE_LOOP('',(#11080,#11081,#11082,#11083));
#2692=EDGE_LOOP('',(#11084));
#2693=EDGE_LOOP('',(#11085,#11086,#11087,#11088));
#2694=EDGE_LOOP('',(#11089,#11090,#11091,#11092));
#2695=EDGE_LOOP('',(#11093,#11094,#11095,#11096));
#2696=EDGE_LOOP('',(#11097,#11098,#11099,#11100));
#2697=EDGE_LOOP('',(#11101,#11102,#11103,#11104));
#2698=EDGE_LOOP('',(#11105,#11106,#11107,#11108));
#2699=EDGE_LOOP('',(#11109,#11110,#11111,#11112));
#2700=EDGE_LOOP('',(#11113,#11114,#11115,#11116));
#2701=EDGE_LOOP('',(#11117,#11118,#11119,#11120));
#2702=EDGE_LOOP('',(#11121,#11122,#11123,#11124));
#2703=EDGE_LOOP('',(#11125,#11126,#11127,#11128));
#2704=EDGE_LOOP('',(#11129,#11130,#11131,#11132));
#2705=EDGE_LOOP('',(#11133,#11134,#11135,#11136));
#2706=EDGE_LOOP('',(#11137,#11138,#11139,#11140));
#2707=EDGE_LOOP('',(#11141,#11142,#11143,#11144));
#2708=EDGE_LOOP('',(#11145,#11146,#11147,#11148));
#2709=EDGE_LOOP('',(#11149,#11150,#11151,#11152));
#2710=EDGE_LOOP('',(#11153,#11154,#11155,#11156));
#2711=EDGE_LOOP('',(#11157,#11158,#11159,#11160));
#2712=EDGE_LOOP('',(#11161,#11162,#11163,#11164));
#2713=EDGE_LOOP('',(#11165,#11166,#11167,#11168));
#2714=EDGE_LOOP('',(#11169,#11170,#11171,#11172));
#2715=EDGE_LOOP('',(#11173,#11174,#11175,#11176));
#2716=EDGE_LOOP('',(#11177,#11178,#11179,#11180));
#2717=EDGE_LOOP('',(#11181,#11182,#11183,#11184));
#2718=EDGE_LOOP('',(#11185,#11186,#11187,#11188));
#2719=EDGE_LOOP('',(#11189,#11190,#11191,#11192));
#2720=EDGE_LOOP('',(#11193,#11194,#11195,#11196));
#2721=EDGE_LOOP('',(#11197,#11198,#11199,#11200));
#2722=EDGE_LOOP('',(#11201,#11202,#11203,#11204));
#2723=EDGE_LOOP('',(#11205,#11206,#11207,#11208));
#2724=EDGE_LOOP('',(#11209,#11210,#11211,#11212));
#2725=EDGE_LOOP('',(#11213,#11214,#11215,#11216));
#2726=EDGE_LOOP('',(#11217,#11218,#11219,#11220));
#2727=EDGE_LOOP('',(#11221,#11222,#11223,#11224));
#2728=EDGE_LOOP('',(#11225,#11226,#11227,#11228));
#2729=EDGE_LOOP('',(#11229,#11230,#11231,#11232));
#2730=EDGE_LOOP('',(#11233,#11234,#11235,#11236));
#2731=EDGE_LOOP('',(#11237,#11238,#11239,#11240));
#2732=EDGE_LOOP('',(#11241,#11242,#11243,#11244));
#2733=EDGE_LOOP('',(#11245,#11246,#11247,#11248));
#2734=EDGE_LOOP('',(#11249,#11250,#11251,#11252));
#2735=EDGE_LOOP('',(#11253,#11254,#11255,#11256));
#2736=EDGE_LOOP('',(#11257,#11258,#11259,#11260));
#2737=EDGE_LOOP('',(#11261,#11262,#11263,#11264));
#2738=EDGE_LOOP('',(#11265,#11266,#11267,#11268));
#2739=EDGE_LOOP('',(#11269,#11270,#11271,#11272));
#2740=EDGE_LOOP('',(#11273,#11274,#11275,#11276));
#2741=EDGE_LOOP('',(#11277,#11278,#11279,#11280));
#2742=EDGE_LOOP('',(#11281,#11282,#11283,#11284));
#2743=EDGE_LOOP('',(#11285,#11286,#11287,#11288));
#2744=EDGE_LOOP('',(#11289,#11290,#11291,#11292));
#2745=EDGE_LOOP('',(#11293,#11294,#11295,#11296));
#2746=EDGE_LOOP('',(#11297,#11298,#11299,#11300));
#2747=EDGE_LOOP('',(#11301,#11302,#11303,#11304));
#2748=EDGE_LOOP('',(#11305,#11306,#11307,#11308));
#2749=EDGE_LOOP('',(#11309,#11310,#11311,#11312));
#2750=EDGE_LOOP('',(#11313,#11314,#11315,#11316));
#2751=EDGE_LOOP('',(#11317,#11318,#11319,#11320));
#2752=EDGE_LOOP('',(#11321,#11322,#11323,#11324));
#2753=EDGE_LOOP('',(#11325,#11326,#11327,#11328));
#2754=EDGE_LOOP('',(#11329,#11330,#11331,#11332));
#2755=EDGE_LOOP('',(#11333,#11334,#11335,#11336));
#2756=EDGE_LOOP('',(#11337,#11338,#11339,#11340));
#2757=EDGE_LOOP('',(#11341,#11342,#11343,#11344));
#2758=EDGE_LOOP('',(#11345,#11346,#11347,#11348));
#2759=EDGE_LOOP('',(#11349,#11350,#11351,#11352));
#2760=EDGE_LOOP('',(#11353,#11354,#11355,#11356));
#2761=EDGE_LOOP('',(#11357,#11358,#11359,#11360));
#2762=EDGE_LOOP('',(#11361,#11362,#11363,#11364));
#2763=EDGE_LOOP('',(#11365,#11366,#11367,#11368));
#2764=EDGE_LOOP('',(#11369,#11370,#11371,#11372));
#2765=EDGE_LOOP('',(#11373,#11374,#11375,#11376));
#2766=EDGE_LOOP('',(#11377,#11378,#11379,#11380));
#2767=EDGE_LOOP('',(#11381,#11382,#11383,#11384));
#2768=EDGE_LOOP('',(#11385,#11386,#11387,#11388));
#2769=EDGE_LOOP('',(#11389,#11390,#11391,#11392));
#2770=EDGE_LOOP('',(#11393,#11394,#11395,#11396));
#2771=EDGE_LOOP('',(#11397,#11398,#11399,#11400));
#2772=EDGE_LOOP('',(#11401,#11402,#11403,#11404));
#2773=EDGE_LOOP('',(#11405,#11406,#11407,#11408,#11409,#11410,#11411,#11412,
#11413,#11414,#11415,#11416,#11417,#11418,#11419,#11420,#11421,#11422,#11423,
#11424,#11425,#11426,#11427,#11428,#11429,#11430,#11431,#11432,#11433,#11434,
#11435,#11436,#11437,#11438,#11439,#11440,#11441,#11442,#11443,#11444,#11445,
#11446,#11447,#11448,#11449,#11450,#11451,#11452,#11453,#11454,#11455,#11456,
#11457,#11458,#11459,#11460,#11461,#11462,#11463,#11464,#11465,#11466,#11467,
#11468,#11469,#11470,#11471,#11472,#11473,#11474,#11475,#11476,#11477,#11478,
#11479,#11480,#11481,#11482,#11483,#11484));
#2774=EDGE_LOOP('',(#11485));
#2775=EDGE_LOOP('',(#11486,#11487,#11488,#11489));
#3812=LINE('',#20825,#4983);
#3813=LINE('',#20827,#4984);
#3814=LINE('',#20829,#4985);
#3815=LINE('',#20830,#4986);
#3816=LINE('',#20833,#4987);
#3817=LINE('',#20835,#4988);
#3818=LINE('',#20836,#4989);
#3819=LINE('',#20839,#4990);
#3820=LINE('',#20841,#4991);
#3821=LINE('',#20842,#4992);
#3822=LINE('',#20919,#4993);
#3823=LINE('',#21065,#4994);
#3824=LINE('',#21211,#4995);
#3825=LINE('',#21357,#4996);
#3826=LINE('',#21503,#4997);
#3827=LINE('',#21649,#4998);
#3828=LINE('',#21795,#4999);
#3829=LINE('',#21941,#5000);
#3830=LINE('',#22087,#5001);
#3831=LINE('',#22233,#5002);
#3832=LINE('',#22379,#5003);
#3833=LINE('',#22525,#5004);
#3834=LINE('',#22671,#5005);
#3835=LINE('',#22817,#5006);
#3836=LINE('',#22963,#5007);
#3837=LINE('',#23109,#5008);
#3838=LINE('',#23255,#5009);
#3839=LINE('',#23401,#5010);
#3840=LINE('',#23547,#5011);
#3841=LINE('',#23693,#5012);
#3842=LINE('',#23771,#5013);
#3843=LINE('',#23915,#5014);
#3844=LINE('',#23987,#5015);
#3845=LINE('',#23990,#5016);
#3846=LINE('',#23991,#5017);
#3847=LINE('',#24203,#5018);
#3848=LINE('',#24207,#5019);
#3849=LINE('',#24419,#5020);
#3850=LINE('',#24422,#5021);
#3851=LINE('',#24423,#5022);
#3852=LINE('',#24635,#5023);
#3853=LINE('',#24639,#5024);
#3854=LINE('',#24851,#5025);
#3855=LINE('',#24854,#5026);
#3856=LINE('',#24855,#5027);
#3857=LINE('',#25067,#5028);
#3858=LINE('',#25071,#5029);
#3859=LINE('',#25283,#5030);
#3860=LINE('',#25286,#5031);
#3861=LINE('',#25287,#5032);
#3862=LINE('',#25499,#5033);
#3863=LINE('',#25503,#5034);
#3864=LINE('',#25715,#5035);
#3865=LINE('',#25718,#5036);
#3866=LINE('',#25719,#5037);
#3867=LINE('',#25931,#5038);
#3868=LINE('',#25935,#5039);
#3869=LINE('',#26147,#5040);
#3870=LINE('',#26150,#5041);
#3871=LINE('',#26151,#5042);
#3872=LINE('',#26363,#5043);
#3873=LINE('',#26367,#5044);
#3874=LINE('',#26579,#5045);
#3875=LINE('',#26582,#5046);
#3876=LINE('',#26583,#5047);
#3877=LINE('',#26795,#5048);
#3878=LINE('',#26799,#5049);
#3879=LINE('',#27011,#5050);
#3880=LINE('',#27014,#5051);
#3881=LINE('',#27015,#5052);
#3882=LINE('',#27227,#5053);
#3883=LINE('',#27231,#5054);
#3884=LINE('',#27443,#5055);
#3885=LINE('',#27446,#5056);
#3886=LINE('',#27447,#5057);
#3887=LINE('',#27659,#5058);
#3888=LINE('',#27663,#5059);
#3889=LINE('',#27875,#5060);
#3890=LINE('',#27878,#5061);
#3891=LINE('',#27879,#5062);
#3892=LINE('',#28091,#5063);
#3893=LINE('',#28095,#5064);
#3894=LINE('',#28307,#5065);
#3895=LINE('',#28310,#5066);
#3896=LINE('',#28311,#5067);
#3897=LINE('',#28523,#5068);
#3898=LINE('',#28527,#5069);
#3899=LINE('',#28739,#5070);
#3900=LINE('',#28742,#5071);
#3901=LINE('',#28743,#5072);
#3902=LINE('',#28955,#5073);
#3903=LINE('',#28959,#5074);
#3904=LINE('',#29171,#5075);
#3905=LINE('',#29174,#5076);
#3906=LINE('',#29175,#5077);
#3907=LINE('',#29387,#5078);
#3908=LINE('',#29391,#5079);
#3909=LINE('',#29603,#5080);
#3910=LINE('',#29606,#5081);
#3911=LINE('',#29607,#5082);
#3912=LINE('',#29819,#5083);
#3913=LINE('',#29823,#5084);
#3914=LINE('',#30035,#5085);
#3915=LINE('',#30038,#5086);
#3916=LINE('',#30039,#5087);
#3917=LINE('',#30251,#5088);
#3918=LINE('',#30255,#5089);
#3919=LINE('',#30467,#5090);
#3920=LINE('',#30470,#5091);
#3921=LINE('',#30471,#5092);
#3922=LINE('',#30683,#5093);
#3923=LINE('',#30687,#5094);
#3924=LINE('',#30899,#5095);
#3925=LINE('',#30902,#5096);
#3926=LINE('',#30903,#5097);
#3927=LINE('',#31115,#5098);
#3928=LINE('',#31119,#5099);
#3929=LINE('',#31331,#5100);
#3930=LINE('',#31334,#5101);
#3931=LINE('',#31335,#5102);
#3932=LINE('',#31547,#5103);
#3933=LINE('',#31551,#5104);
#3934=LINE('',#31763,#5105);
#3935=LINE('',#31766,#5106);
#3936=LINE('',#31767,#5107);
#3937=LINE('',#31979,#5108);
#3938=LINE('',#31983,#5109);
#3939=LINE('',#32195,#5110);
#3940=LINE('',#32198,#5111);
#3941=LINE('',#32199,#5112);
#3942=LINE('',#32411,#5113);
#4983=VECTOR('',#16995,1.);
#4984=VECTOR('',#16996,1.);
#4985=VECTOR('',#16997,1.);
#4986=VECTOR('',#16998,1.);
#4987=VECTOR('',#17001,1.);
#4988=VECTOR('',#17002,1.);
#4989=VECTOR('',#17003,1.);
#4990=VECTOR('',#17006,1.);
#4991=VECTOR('',#17007,1.);
#4992=VECTOR('',#17008,1.);
#4993=VECTOR('',#17013,1.);
#4994=VECTOR('',#17016,1.);
#4995=VECTOR('',#17019,1.);
#4996=VECTOR('',#17022,1.);
#4997=VECTOR('',#17025,1.);
#4998=VECTOR('',#17028,1.);
#4999=VECTOR('',#17031,1.);
#5000=VECTOR('',#17034,1.);
#5001=VECTOR('',#17037,1.);
#5002=VECTOR('',#17040,1.);
#5003=VECTOR('',#17043,1.);
#5004=VECTOR('',#17046,1.);
#5005=VECTOR('',#17049,1.);
#5006=VECTOR('',#17052,1.);
#5007=VECTOR('',#17055,1.);
#5008=VECTOR('',#17058,1.);
#5009=VECTOR('',#17061,1.);
#5010=VECTOR('',#17064,1.);
#5011=VECTOR('',#17067,1.);
#5012=VECTOR('',#17070,1.);
#5013=VECTOR('',#17081,1.4);
#5014=VECTOR('',#17086,1.);
#5015=VECTOR('',#17087,1.);
#5016=VECTOR('',#17090,1.);
#5017=VECTOR('',#17091,1.);
#5018=VECTOR('',#17092,1.);
#5019=VECTOR('',#17097,1.);
#5020=VECTOR('',#17098,1.);
#5021=VECTOR('',#17101,1.);
#5022=VECTOR('',#17102,1.);
#5023=VECTOR('',#17103,1.);
#5024=VECTOR('',#17108,1.);
#5025=VECTOR('',#17109,1.);
#5026=VECTOR('',#17112,1.);
#5027=VECTOR('',#17113,1.);
#5028=VECTOR('',#17114,1.);
#5029=VECTOR('',#17119,1.);
#5030=VECTOR('',#17120,1.);
#5031=VECTOR('',#17123,1.);
#5032=VECTOR('',#17124,1.);
#5033=VECTOR('',#17125,1.);
#5034=VECTOR('',#17130,1.);
#5035=VECTOR('',#17131,1.);
#5036=VECTOR('',#17134,1.);
#5037=VECTOR('',#17135,1.);
#5038=VECTOR('',#17136,1.);
#5039=VECTOR('',#17141,1.);
#5040=VECTOR('',#17142,1.);
#5041=VECTOR('',#17145,1.);
#5042=VECTOR('',#17146,1.);
#5043=VECTOR('',#17147,1.);
#5044=VECTOR('',#17152,1.);
#5045=VECTOR('',#17153,1.);
#5046=VECTOR('',#17156,1.);
#5047=VECTOR('',#17157,1.);
#5048=VECTOR('',#17158,1.);
#5049=VECTOR('',#17163,1.);
#5050=VECTOR('',#17164,1.);
#5051=VECTOR('',#17167,1.);
#5052=VECTOR('',#17168,1.);
#5053=VECTOR('',#17169,1.);
#5054=VECTOR('',#17174,1.);
#5055=VECTOR('',#17175,1.);
#5056=VECTOR('',#17178,1.);
#5057=VECTOR('',#17179,1.);
#5058=VECTOR('',#17180,1.);
#5059=VECTOR('',#17185,1.);
#5060=VECTOR('',#17186,1.);
#5061=VECTOR('',#17189,1.);
#5062=VECTOR('',#17190,1.);
#5063=VECTOR('',#17191,1.);
#5064=VECTOR('',#17196,1.);
#5065=VECTOR('',#17197,1.);
#5066=VECTOR('',#17200,1.);
#5067=VECTOR('',#17201,1.);
#5068=VECTOR('',#17202,1.);
#5069=VECTOR('',#17207,1.);
#5070=VECTOR('',#17208,1.);
#5071=VECTOR('',#17211,1.);
#5072=VECTOR('',#17212,1.);
#5073=VECTOR('',#17213,1.);
#5074=VECTOR('',#17218,1.);
#5075=VECTOR('',#17219,1.);
#5076=VECTOR('',#17222,1.);
#5077=VECTOR('',#17223,1.);
#5078=VECTOR('',#17224,1.);
#5079=VECTOR('',#17229,1.);
#5080=VECTOR('',#17230,1.);
#5081=VECTOR('',#17233,1.);
#5082=VECTOR('',#17234,1.);
#5083=VECTOR('',#17235,1.);
#5084=VECTOR('',#17240,1.);
#5085=VECTOR('',#17241,1.);
#5086=VECTOR('',#17244,1.);
#5087=VECTOR('',#17245,1.);
#5088=VECTOR('',#17246,1.);
#5089=VECTOR('',#17251,1.);
#5090=VECTOR('',#17252,1.);
#5091=VECTOR('',#17255,1.);
#5092=VECTOR('',#17256,1.);
#5093=VECTOR('',#17257,1.);
#5094=VECTOR('',#17262,1.);
#5095=VECTOR('',#17263,1.);
#5096=VECTOR('',#17266,1.);
#5097=VECTOR('',#17267,1.);
#5098=VECTOR('',#17268,1.);
#5099=VECTOR('',#17273,1.);
#5100=VECTOR('',#17274,1.);
#5101=VECTOR('',#17277,1.);
#5102=VECTOR('',#17278,1.);
#5103=VECTOR('',#17279,1.);
#5104=VECTOR('',#17284,1.);
#5105=VECTOR('',#17285,1.);
#5106=VECTOR('',#17288,1.);
#5107=VECTOR('',#17289,1.);
#5108=VECTOR('',#17290,1.);
#5109=VECTOR('',#17295,1.);
#5110=VECTOR('',#17296,1.);
#5111=VECTOR('',#17299,1.);
#5112=VECTOR('',#17300,1.);
#5113=VECTOR('',#17301,1.);
#5488=CIRCLE('',#13928,1.75);
#5489=CIRCLE('',#13929,1.75);
#5490=CIRCLE('',#13930,1.75);
#5491=CIRCLE('',#13931,1.75);
#5492=CIRCLE('',#13932,1.75);
#5493=CIRCLE('',#13933,1.75);
#5494=CIRCLE('',#13934,1.75);
#5495=CIRCLE('',#13935,1.75);
#5496=CIRCLE('',#13936,1.75);
#5497=CIRCLE('',#13937,1.75);
#5498=CIRCLE('',#13938,1.75);
#5499=CIRCLE('',#13939,1.75);
#5500=CIRCLE('',#13940,1.75);
#5501=CIRCLE('',#13941,1.75);
#5502=CIRCLE('',#13942,1.75);
#5503=CIRCLE('',#13943,1.75);
#5504=CIRCLE('',#13944,1.75);
#5505=CIRCLE('',#13945,1.75);
#5506=CIRCLE('',#13946,1.75);
#5507=CIRCLE('',#13947,1.75);
#5508=CIRCLE('',#13948,0.6);
#5509=CIRCLE('',#13950,0.6);
#5510=CIRCLE('',#13952,1.4);
#5511=CIRCLE('',#13953,1.4);
#5512=CIRCLE('',#13957,1.75);
#5513=CIRCLE('',#13960,1.75);
#5514=CIRCLE('',#13963,1.75);
#5515=CIRCLE('',#13966,1.75);
#5516=CIRCLE('',#13969,1.75);
#5517=CIRCLE('',#13972,1.75);
#5518=CIRCLE('',#13975,1.75);
#5519=CIRCLE('',#13978,1.75);
#5520=CIRCLE('',#13981,1.75);
#5521=CIRCLE('',#13984,1.75);
#5522=CIRCLE('',#13987,1.75);
#5523=CIRCLE('',#13990,1.75);
#5524=CIRCLE('',#13993,1.75);
#5525=CIRCLE('',#13996,1.75);
#5526=CIRCLE('',#13999,1.75);
#5527=CIRCLE('',#14002,1.75);
#5528=CIRCLE('',#14005,1.75);
#5529=CIRCLE('',#14008,1.75);
#5530=CIRCLE('',#14011,1.75);
#5531=CIRCLE('',#14014,1.75);
#6447=VERTEX_POINT('',#20823);
#6448=VERTEX_POINT('',#20824);
#6449=VERTEX_POINT('',#20826);
#6450=VERTEX_POINT('',#20828);
#6451=VERTEX_POINT('',#20832);
#6452=VERTEX_POINT('',#20834);
#6453=VERTEX_POINT('',#20838);
#6454=VERTEX_POINT('',#20840);
#6455=VERTEX_POINT('',#20844);
#6456=VERTEX_POINT('',#20845);
#6457=VERTEX_POINT('',#20847);
#6458=VERTEX_POINT('',#20918);
#6459=VERTEX_POINT('',#20920);
#6460=VERTEX_POINT('',#20991);
#6461=VERTEX_POINT('',#20993);
#6462=VERTEX_POINT('',#21064);
#6463=VERTEX_POINT('',#21066);
#6464=VERTEX_POINT('',#21137);
#6465=VERTEX_POINT('',#21139);
#6466=VERTEX_POINT('',#21210);
#6467=VERTEX_POINT('',#21212);
#6468=VERTEX_POINT('',#21283);
#6469=VERTEX_POINT('',#21285);
#6470=VERTEX_POINT('',#21356);
#6471=VERTEX_POINT('',#21358);
#6472=VERTEX_POINT('',#21429);
#6473=VERTEX_POINT('',#21431);
#6474=VERTEX_POINT('',#21502);
#6475=VERTEX_POINT('',#21504);
#6476=VERTEX_POINT('',#21575);
#6477=VERTEX_POINT('',#21577);
#6478=VERTEX_POINT('',#21648);
#6479=VERTEX_POINT('',#21650);
#6480=VERTEX_POINT('',#21721);
#6481=VERTEX_POINT('',#21723);
#6482=VERTEX_POINT('',#21794);
#6483=VERTEX_POINT('',#21796);
#6484=VERTEX_POINT('',#21867);
#6485=VERTEX_POINT('',#21869);
#6486=VERTEX_POINT('',#21940);
#6487=VERTEX_POINT('',#21942);
#6488=VERTEX_POINT('',#22013);
#6489=VERTEX_POINT('',#22015);
#6490=VERTEX_POINT('',#22086);
#6491=VERTEX_POINT('',#22088);
#6492=VERTEX_POINT('',#22159);
#6493=VERTEX_POINT('',#22161);
#6494=VERTEX_POINT('',#22232);
#6495=VERTEX_POINT('',#22234);
#6496=VERTEX_POINT('',#22305);
#6497=VERTEX_POINT('',#22307);
#6498=VERTEX_POINT('',#22378);
#6499=VERTEX_POINT('',#22380);
#6500=VERTEX_POINT('',#22451);
#6501=VERTEX_POINT('',#22453);
#6502=VERTEX_POINT('',#22524);
#6503=VERTEX_POINT('',#22526);
#6504=VERTEX_POINT('',#22597);
#6505=VERTEX_POINT('',#22599);
#6506=VERTEX_POINT('',#22670);
#6507=VERTEX_POINT('',#22672);
#6508=VERTEX_POINT('',#22743);
#6509=VERTEX_POINT('',#22745);
#6510=VERTEX_POINT('',#22816);
#6511=VERTEX_POINT('',#22818);
#6512=VERTEX_POINT('',#22889);
#6513=VERTEX_POINT('',#22891);
#6514=VERTEX_POINT('',#22962);
#6515=VERTEX_POINT('',#22964);
#6516=VERTEX_POINT('',#23035);
#6517=VERTEX_POINT('',#23037);
#6518=VERTEX_POINT('',#23108);
#6519=VERTEX_POINT('',#23110);
#6520=VERTEX_POINT('',#23181);
#6521=VERTEX_POINT('',#23183);
#6522=VERTEX_POINT('',#23254);
#6523=VERTEX_POINT('',#23256);
#6524=VERTEX_POINT('',#23327);
#6525=VERTEX_POINT('',#23329);
#6526=VERTEX_POINT('',#23400);
#6527=VERTEX_POINT('',#23402);
#6528=VERTEX_POINT('',#23473);
#6529=VERTEX_POINT('',#23475);
#6530=VERTEX_POINT('',#23546);
#6531=VERTEX_POINT('',#23548);
#6532=VERTEX_POINT('',#23619);
#6533=VERTEX_POINT('',#23621);
#6534=VERTEX_POINT('',#23692);
#6535=VERTEX_POINT('',#23768);
#6536=VERTEX_POINT('',#23770);
#6537=VERTEX_POINT('',#23914);
#6538=VERTEX_POINT('',#23916);
#6539=VERTEX_POINT('',#23989);
#6540=VERTEX_POINT('',#24132);
#6541=VERTEX_POINT('',#24205);
#6542=VERTEX_POINT('',#24348);
#6543=VERTEX_POINT('',#24421);
#6544=VERTEX_POINT('',#24564);
#6545=VERTEX_POINT('',#24637);
#6546=VERTEX_POINT('',#24780);
#6547=VERTEX_POINT('',#24853);
#6548=VERTEX_POINT('',#24996);
#6549=VERTEX_POINT('',#25069);
#6550=VERTEX_POINT('',#25212);
#6551=VERTEX_POINT('',#25285);
#6552=VERTEX_POINT('',#25428);
#6553=VERTEX_POINT('',#25501);
#6554=VERTEX_POINT('',#25644);
#6555=VERTEX_POINT('',#25717);
#6556=VERTEX_POINT('',#25860);
#6557=VERTEX_POINT('',#25933);
#6558=VERTEX_POINT('',#26076);
#6559=VERTEX_POINT('',#26149);
#6560=VERTEX_POINT('',#26292);
#6561=VERTEX_POINT('',#26365);
#6562=VERTEX_POINT('',#26508);
#6563=VERTEX_POINT('',#26581);
#6564=VERTEX_POINT('',#26724);
#6565=VERTEX_POINT('',#26797);
#6566=VERTEX_POINT('',#26940);
#6567=VERTEX_POINT('',#27013);
#6568=VERTEX_POINT('',#27156);
#6569=VERTEX_POINT('',#27229);
#6570=VERTEX_POINT('',#27372);
#6571=VERTEX_POINT('',#27445);
#6572=VERTEX_POINT('',#27588);
#6573=VERTEX_POINT('',#27661);
#6574=VERTEX_POINT('',#27804);
#6575=VERTEX_POINT('',#27877);
#6576=VERTEX_POINT('',#28020);
#6577=VERTEX_POINT('',#28093);
#6578=VERTEX_POINT('',#28236);
#6579=VERTEX_POINT('',#28309);
#6580=VERTEX_POINT('',#28452);
#6581=VERTEX_POINT('',#28525);
#6582=VERTEX_POINT('',#28668);
#6583=VERTEX_POINT('',#28741);
#6584=VERTEX_POINT('',#28884);
#6585=VERTEX_POINT('',#28957);
#6586=VERTEX_POINT('',#29100);
#6587=VERTEX_POINT('',#29173);
#6588=VERTEX_POINT('',#29316);
#6589=VERTEX_POINT('',#29389);
#6590=VERTEX_POINT('',#29532);
#6591=VERTEX_POINT('',#29605);
#6592=VERTEX_POINT('',#29748);
#6593=VERTEX_POINT('',#29821);
#6594=VERTEX_POINT('',#29964);
#6595=VERTEX_POINT('',#30037);
#6596=VERTEX_POINT('',#30180);
#6597=VERTEX_POINT('',#30253);
#6598=VERTEX_POINT('',#30396);
#6599=VERTEX_POINT('',#30469);
#6600=VERTEX_POINT('',#30612);
#6601=VERTEX_POINT('',#30685);
#6602=VERTEX_POINT('',#30828);
#6603=VERTEX_POINT('',#30901);
#6604=VERTEX_POINT('',#31044);
#6605=VERTEX_POINT('',#31117);
#6606=VERTEX_POINT('',#31260);
#6607=VERTEX_POINT('',#31333);
#6608=VERTEX_POINT('',#31476);
#6609=VERTEX_POINT('',#31549);
#6610=VERTEX_POINT('',#31692);
#6611=VERTEX_POINT('',#31765);
#6612=VERTEX_POINT('',#31908);
#6613=VERTEX_POINT('',#31981);
#6614=VERTEX_POINT('',#32124);
#6615=VERTEX_POINT('',#32197);
#6616=VERTEX_POINT('',#32340);
#7993=EDGE_CURVE('',#6447,#6448,#3812,.T.);
#7994=EDGE_CURVE('',#6449,#6447,#3813,.T.);
#7995=EDGE_CURVE('',#6450,#6449,#3814,.T.);
#7996=EDGE_CURVE('',#6448,#6450,#3815,.T.);
#7997=EDGE_CURVE('',#6451,#6447,#3816,.T.);
#7998=EDGE_CURVE('',#6451,#6452,#3817,.T.);
#7999=EDGE_CURVE('',#6449,#6452,#3818,.T.);
#8000=EDGE_CURVE('',#6453,#6451,#3819,.T.);
#8001=EDGE_CURVE('',#6454,#6453,#3820,.T.);
#8002=EDGE_CURVE('',#6452,#6454,#3821,.T.);
#8003=EDGE_CURVE('',#6455,#6456,#5488,.T.);
#8004=EDGE_CURVE('',#6456,#6457,#51,.T.);
#8005=EDGE_CURVE('',#6457,#6458,#3822,.T.);
#8006=EDGE_CURVE('',#6458,#6459,#52,.T.);
#8007=EDGE_CURVE('',#6459,#6460,#5489,.T.);
#8008=EDGE_CURVE('',#6460,#6461,#53,.T.);
#8009=EDGE_CURVE('',#6461,#6462,#3823,.T.);
#8010=EDGE_CURVE('',#6462,#6463,#54,.T.);
#8011=EDGE_CURVE('',#6463,#6464,#5490,.T.);
#8012=EDGE_CURVE('',#6464,#6465,#55,.T.);
#8013=EDGE_CURVE('',#6465,#6466,#3824,.T.);
#8014=EDGE_CURVE('',#6466,#6467,#56,.T.);
#8015=EDGE_CURVE('',#6467,#6468,#5491,.T.);
#8016=EDGE_CURVE('',#6468,#6469,#57,.T.);
#8017=EDGE_CURVE('',#6469,#6470,#3825,.T.);
#8018=EDGE_CURVE('',#6470,#6471,#58,.T.);
#8019=EDGE_CURVE('',#6471,#6472,#5492,.T.);
#8020=EDGE_CURVE('',#6472,#6473,#59,.T.);
#8021=EDGE_CURVE('',#6473,#6474,#3826,.T.);
#8022=EDGE_CURVE('',#6474,#6475,#60,.T.);
#8023=EDGE_CURVE('',#6475,#6476,#5493,.T.);
#8024=EDGE_CURVE('',#6476,#6477,#61,.T.);
#8025=EDGE_CURVE('',#6477,#6478,#3827,.T.);
#8026=EDGE_CURVE('',#6478,#6479,#62,.T.);
#8027=EDGE_CURVE('',#6479,#6480,#5494,.T.);
#8028=EDGE_CURVE('',#6480,#6481,#63,.T.);
#8029=EDGE_CURVE('',#6481,#6482,#3828,.T.);
#8030=EDGE_CURVE('',#6482,#6483,#64,.T.);
#8031=EDGE_CURVE('',#6483,#6484,#5495,.T.);
#8032=EDGE_CURVE('',#6484,#6485,#65,.T.);
#8033=EDGE_CURVE('',#6485,#6486,#3829,.T.);
#8034=EDGE_CURVE('',#6486,#6487,#66,.T.);
#8035=EDGE_CURVE('',#6487,#6488,#5496,.T.);
#8036=EDGE_CURVE('',#6488,#6489,#67,.T.);
#8037=EDGE_CURVE('',#6489,#6490,#3830,.T.);
#8038=EDGE_CURVE('',#6490,#6491,#68,.T.);
#8039=EDGE_CURVE('',#6491,#6492,#5497,.T.);
#8040=EDGE_CURVE('',#6492,#6493,#69,.T.);
#8041=EDGE_CURVE('',#6493,#6494,#3831,.T.);
#8042=EDGE_CURVE('',#6494,#6495,#70,.T.);
#8043=EDGE_CURVE('',#6495,#6496,#5498,.T.);
#8044=EDGE_CURVE('',#6496,#6497,#71,.T.);
#8045=EDGE_CURVE('',#6497,#6498,#3832,.T.);
#8046=EDGE_CURVE('',#6498,#6499,#72,.T.);
#8047=EDGE_CURVE('',#6499,#6500,#5499,.T.);
#8048=EDGE_CURVE('',#6500,#6501,#73,.T.);
#8049=EDGE_CURVE('',#6501,#6502,#3833,.T.);
#8050=EDGE_CURVE('',#6502,#6503,#74,.T.);
#8051=EDGE_CURVE('',#6503,#6504,#5500,.T.);
#8052=EDGE_CURVE('',#6504,#6505,#75,.T.);
#8053=EDGE_CURVE('',#6505,#6506,#3834,.T.);
#8054=EDGE_CURVE('',#6506,#6507,#76,.T.);
#8055=EDGE_CURVE('',#6507,#6508,#5501,.T.);
#8056=EDGE_CURVE('',#6508,#6509,#77,.T.);
#8057=EDGE_CURVE('',#6509,#6510,#3835,.T.);
#8058=EDGE_CURVE('',#6510,#6511,#78,.T.);
#8059=EDGE_CURVE('',#6511,#6512,#5502,.T.);
#8060=EDGE_CURVE('',#6512,#6513,#79,.T.);
#8061=EDGE_CURVE('',#6513,#6514,#3836,.T.);
#8062=EDGE_CURVE('',#6514,#6515,#80,.T.);
#8063=EDGE_CURVE('',#6515,#6516,#5503,.T.);
#8064=EDGE_CURVE('',#6516,#6517,#81,.T.);
#8065=EDGE_CURVE('',#6517,#6518,#3837,.T.);
#8066=EDGE_CURVE('',#6518,#6519,#82,.T.);
#8067=EDGE_CURVE('',#6519,#6520,#5504,.T.);
#8068=EDGE_CURVE('',#6520,#6521,#83,.T.);
#8069=EDGE_CURVE('',#6521,#6522,#3838,.T.);
#8070=EDGE_CURVE('',#6522,#6523,#84,.T.);
#8071=EDGE_CURVE('',#6523,#6524,#5505,.T.);
#8072=EDGE_CURVE('',#6524,#6525,#85,.T.);
#8073=EDGE_CURVE('',#6525,#6526,#3839,.T.);
#8074=EDGE_CURVE('',#6526,#6527,#86,.T.);
#8075=EDGE_CURVE('',#6527,#6528,#5506,.T.);
#8076=EDGE_CURVE('',#6528,#6529,#87,.T.);
#8077=EDGE_CURVE('',#6529,#6530,#3840,.T.);
#8078=EDGE_CURVE('',#6530,#6531,#88,.T.);
#8079=EDGE_CURVE('',#6531,#6532,#5507,.T.);
#8080=EDGE_CURVE('',#6532,#6533,#89,.T.);
#8081=EDGE_CURVE('',#6533,#6534,#3841,.T.);
#8082=EDGE_CURVE('',#6534,#6455,#90,.T.);
#8083=EDGE_CURVE('',#6454,#6450,#5508,.T.);
#8084=EDGE_CURVE('',#6448,#6453,#5509,.T.);
#8085=EDGE_CURVE('',#6535,#6535,#5510,.T.);
#8086=EDGE_CURVE('',#6535,#6536,#3842,.T.);
#8087=EDGE_CURVE('',#6536,#6536,#5511,.T.);
#8088=EDGE_CURVE('',#6537,#6532,#3843,.T.);
#8089=EDGE_CURVE('',#6538,#6537,#91,.T.);
#8090=EDGE_CURVE('',#6533,#6538,#3844,.T.);
#8091=EDGE_CURVE('',#6539,#6538,#3845,.T.);
#8092=EDGE_CURVE('',#6534,#6539,#3846,.T.);
#8093=EDGE_CURVE('',#6540,#6539,#92,.T.);
#8094=EDGE_CURVE('',#6455,#6540,#3847,.T.);
#8095=EDGE_CURVE('',#6541,#6540,#5512,.T.);
#8096=EDGE_CURVE('',#6541,#6456,#3848,.T.);
#8097=EDGE_CURVE('',#6542,#6541,#93,.T.);
#8098=EDGE_CURVE('',#6457,#6542,#3849,.T.);
#8099=EDGE_CURVE('',#6543,#6542,#3850,.T.);
#8100=EDGE_CURVE('',#6458,#6543,#3851,.T.);
#8101=EDGE_CURVE('',#6544,#6543,#94,.T.);
#8102=EDGE_CURVE('',#6459,#6544,#3852,.T.);
#8103=EDGE_CURVE('',#6545,#6544,#5513,.T.);
#8104=EDGE_CURVE('',#6545,#6460,#3853,.T.);
#8105=EDGE_CURVE('',#6546,#6545,#95,.T.);
#8106=EDGE_CURVE('',#6461,#6546,#3854,.T.);
#8107=EDGE_CURVE('',#6547,#6546,#3855,.T.);
#8108=EDGE_CURVE('',#6462,#6547,#3856,.T.);
#8109=EDGE_CURVE('',#6548,#6547,#96,.T.);
#8110=EDGE_CURVE('',#6463,#6548,#3857,.T.);
#8111=EDGE_CURVE('',#6549,#6548,#5514,.T.);
#8112=EDGE_CURVE('',#6549,#6464,#3858,.T.);
#8113=EDGE_CURVE('',#6550,#6549,#97,.T.);
#8114=EDGE_CURVE('',#6465,#6550,#3859,.T.);
#8115=EDGE_CURVE('',#6551,#6550,#3860,.T.);
#8116=EDGE_CURVE('',#6466,#6551,#3861,.T.);
#8117=EDGE_CURVE('',#6552,#6551,#98,.T.);
#8118=EDGE_CURVE('',#6467,#6552,#3862,.T.);
#8119=EDGE_CURVE('',#6553,#6552,#5515,.T.);
#8120=EDGE_CURVE('',#6553,#6468,#3863,.T.);
#8121=EDGE_CURVE('',#6554,#6553,#99,.T.);
#8122=EDGE_CURVE('',#6469,#6554,#3864,.T.);
#8123=EDGE_CURVE('',#6555,#6554,#3865,.T.);
#8124=EDGE_CURVE('',#6470,#6555,#3866,.T.);
#8125=EDGE_CURVE('',#6556,#6555,#100,.T.);
#8126=EDGE_CURVE('',#6471,#6556,#3867,.T.);
#8127=EDGE_CURVE('',#6557,#6556,#5516,.T.);
#8128=EDGE_CURVE('',#6557,#6472,#3868,.T.);
#8129=EDGE_CURVE('',#6558,#6557,#101,.T.);
#8130=EDGE_CURVE('',#6473,#6558,#3869,.T.);
#8131=EDGE_CURVE('',#6559,#6558,#3870,.T.);
#8132=EDGE_CURVE('',#6474,#6559,#3871,.T.);
#8133=EDGE_CURVE('',#6560,#6559,#102,.T.);
#8134=EDGE_CURVE('',#6475,#6560,#3872,.T.);
#8135=EDGE_CURVE('',#6561,#6560,#5517,.T.);
#8136=EDGE_CURVE('',#6561,#6476,#3873,.T.);
#8137=EDGE_CURVE('',#6562,#6561,#103,.T.);
#8138=EDGE_CURVE('',#6477,#6562,#3874,.T.);
#8139=EDGE_CURVE('',#6563,#6562,#3875,.T.);
#8140=EDGE_CURVE('',#6478,#6563,#3876,.T.);
#8141=EDGE_CURVE('',#6564,#6563,#104,.T.);
#8142=EDGE_CURVE('',#6479,#6564,#3877,.T.);
#8143=EDGE_CURVE('',#6565,#6564,#5518,.T.);
#8144=EDGE_CURVE('',#6565,#6480,#3878,.T.);
#8145=EDGE_CURVE('',#6566,#6565,#105,.T.);
#8146=EDGE_CURVE('',#6481,#6566,#3879,.T.);
#8147=EDGE_CURVE('',#6567,#6566,#3880,.T.);
#8148=EDGE_CURVE('',#6482,#6567,#3881,.T.);
#8149=EDGE_CURVE('',#6568,#6567,#106,.T.);
#8150=EDGE_CURVE('',#6483,#6568,#3882,.T.);
#8151=EDGE_CURVE('',#6569,#6568,#5519,.T.);
#8152=EDGE_CURVE('',#6569,#6484,#3883,.T.);
#8153=EDGE_CURVE('',#6570,#6569,#107,.T.);
#8154=EDGE_CURVE('',#6485,#6570,#3884,.T.);
#8155=EDGE_CURVE('',#6571,#6570,#3885,.T.);
#8156=EDGE_CURVE('',#6486,#6571,#3886,.T.);
#8157=EDGE_CURVE('',#6572,#6571,#108,.T.);
#8158=EDGE_CURVE('',#6487,#6572,#3887,.T.);
#8159=EDGE_CURVE('',#6573,#6572,#5520,.T.);
#8160=EDGE_CURVE('',#6573,#6488,#3888,.T.);
#8161=EDGE_CURVE('',#6574,#6573,#109,.T.);
#8162=EDGE_CURVE('',#6489,#6574,#3889,.T.);
#8163=EDGE_CURVE('',#6575,#6574,#3890,.T.);
#8164=EDGE_CURVE('',#6490,#6575,#3891,.T.);
#8165=EDGE_CURVE('',#6576,#6575,#110,.T.);
#8166=EDGE_CURVE('',#6491,#6576,#3892,.T.);
#8167=EDGE_CURVE('',#6577,#6576,#5521,.T.);
#8168=EDGE_CURVE('',#6577,#6492,#3893,.T.);
#8169=EDGE_CURVE('',#6578,#6577,#111,.T.);
#8170=EDGE_CURVE('',#6493,#6578,#3894,.T.);
#8171=EDGE_CURVE('',#6579,#6578,#3895,.T.);
#8172=EDGE_CURVE('',#6494,#6579,#3896,.T.);
#8173=EDGE_CURVE('',#6580,#6579,#112,.T.);
#8174=EDGE_CURVE('',#6495,#6580,#3897,.T.);
#8175=EDGE_CURVE('',#6581,#6580,#5522,.T.);
#8176=EDGE_CURVE('',#6581,#6496,#3898,.T.);
#8177=EDGE_CURVE('',#6582,#6581,#113,.T.);
#8178=EDGE_CURVE('',#6497,#6582,#3899,.T.);
#8179=EDGE_CURVE('',#6583,#6582,#3900,.T.);
#8180=EDGE_CURVE('',#6498,#6583,#3901,.T.);
#8181=EDGE_CURVE('',#6584,#6583,#114,.T.);
#8182=EDGE_CURVE('',#6499,#6584,#3902,.T.);
#8183=EDGE_CURVE('',#6585,#6584,#5523,.T.);
#8184=EDGE_CURVE('',#6585,#6500,#3903,.T.);
#8185=EDGE_CURVE('',#6586,#6585,#115,.T.);
#8186=EDGE_CURVE('',#6501,#6586,#3904,.T.);
#8187=EDGE_CURVE('',#6587,#6586,#3905,.T.);
#8188=EDGE_CURVE('',#6502,#6587,#3906,.T.);
#8189=EDGE_CURVE('',#6588,#6587,#116,.T.);
#8190=EDGE_CURVE('',#6503,#6588,#3907,.T.);
#8191=EDGE_CURVE('',#6589,#6588,#5524,.T.);
#8192=EDGE_CURVE('',#6589,#6504,#3908,.T.);
#8193=EDGE_CURVE('',#6590,#6589,#117,.T.);
#8194=EDGE_CURVE('',#6505,#6590,#3909,.T.);
#8195=EDGE_CURVE('',#6591,#6590,#3910,.T.);
#8196=EDGE_CURVE('',#6506,#6591,#3911,.T.);
#8197=EDGE_CURVE('',#6592,#6591,#118,.T.);
#8198=EDGE_CURVE('',#6507,#6592,#3912,.T.);
#8199=EDGE_CURVE('',#6593,#6592,#5525,.T.);
#8200=EDGE_CURVE('',#6593,#6508,#3913,.T.);
#8201=EDGE_CURVE('',#6594,#6593,#119,.T.);
#8202=EDGE_CURVE('',#6509,#6594,#3914,.T.);
#8203=EDGE_CURVE('',#6595,#6594,#3915,.T.);
#8204=EDGE_CURVE('',#6510,#6595,#3916,.T.);
#8205=EDGE_CURVE('',#6596,#6595,#120,.T.);
#8206=EDGE_CURVE('',#6511,#6596,#3917,.T.);
#8207=EDGE_CURVE('',#6597,#6596,#5526,.T.);
#8208=EDGE_CURVE('',#6597,#6512,#3918,.T.);
#8209=EDGE_CURVE('',#6598,#6597,#121,.T.);
#8210=EDGE_CURVE('',#6513,#6598,#3919,.T.);
#8211=EDGE_CURVE('',#6599,#6598,#3920,.T.);
#8212=EDGE_CURVE('',#6514,#6599,#3921,.T.);
#8213=EDGE_CURVE('',#6600,#6599,#122,.T.);
#8214=EDGE_CURVE('',#6515,#6600,#3922,.T.);
#8215=EDGE_CURVE('',#6601,#6600,#5527,.T.);
#8216=EDGE_CURVE('',#6601,#6516,#3923,.T.);
#8217=EDGE_CURVE('',#6602,#6601,#123,.T.);
#8218=EDGE_CURVE('',#6517,#6602,#3924,.T.);
#8219=EDGE_CURVE('',#6603,#6602,#3925,.T.);
#8220=EDGE_CURVE('',#6518,#6603,#3926,.T.);
#8221=EDGE_CURVE('',#6604,#6603,#124,.T.);
#8222=EDGE_CURVE('',#6519,#6604,#3927,.T.);
#8223=EDGE_CURVE('',#6605,#6604,#5528,.T.);
#8224=EDGE_CURVE('',#6605,#6520,#3928,.T.);
#8225=EDGE_CURVE('',#6606,#6605,#125,.T.);
#8226=EDGE_CURVE('',#6521,#6606,#3929,.T.);
#8227=EDGE_CURVE('',#6607,#6606,#3930,.T.);
#8228=EDGE_CURVE('',#6522,#6607,#3931,.T.);
#8229=EDGE_CURVE('',#6608,#6607,#126,.T.);
#8230=EDGE_CURVE('',#6523,#6608,#3932,.T.);
#8231=EDGE_CURVE('',#6609,#6608,#5529,.T.);
#8232=EDGE_CURVE('',#6609,#6524,#3933,.T.);
#8233=EDGE_CURVE('',#6610,#6609,#127,.T.);
#8234=EDGE_CURVE('',#6525,#6610,#3934,.T.);
#8235=EDGE_CURVE('',#6611,#6610,#3935,.T.);
#8236=EDGE_CURVE('',#6526,#6611,#3936,.T.);
#8237=EDGE_CURVE('',#6612,#6611,#128,.T.);
#8238=EDGE_CURVE('',#6527,#6612,#3937,.T.);
#8239=EDGE_CURVE('',#6613,#6612,#5530,.T.);
#8240=EDGE_CURVE('',#6613,#6528,#3938,.T.);
#8241=EDGE_CURVE('',#6614,#6613,#129,.T.);
#8242=EDGE_CURVE('',#6529,#6614,#3939,.T.);
#8243=EDGE_CURVE('',#6615,#6614,#3940,.T.);
#8244=EDGE_CURVE('',#6530,#6615,#3941,.T.);
#8245=EDGE_CURVE('',#6616,#6615,#130,.T.);
#8246=EDGE_CURVE('',#6531,#6616,#3942,.T.);
#8247=EDGE_CURVE('',#6537,#6616,#5531,.T.);
#10980=ORIENTED_EDGE('',*,*,#7993,.F.);
#10981=ORIENTED_EDGE('',*,*,#7994,.F.);
#10982=ORIENTED_EDGE('',*,*,#7995,.F.);
#10983=ORIENTED_EDGE('',*,*,#7996,.F.);
#10984=ORIENTED_EDGE('',*,*,#7997,.F.);
#10985=ORIENTED_EDGE('',*,*,#7998,.T.);
#10986=ORIENTED_EDGE('',*,*,#7999,.F.);
#10987=ORIENTED_EDGE('',*,*,#7994,.T.);
#10988=ORIENTED_EDGE('',*,*,#8000,.F.);
#10989=ORIENTED_EDGE('',*,*,#8001,.F.);
#10990=ORIENTED_EDGE('',*,*,#8002,.F.);
#10991=ORIENTED_EDGE('',*,*,#7998,.F.);
#10992=ORIENTED_EDGE('',*,*,#8003,.T.);
#10993=ORIENTED_EDGE('',*,*,#8004,.T.);
#10994=ORIENTED_EDGE('',*,*,#8005,.T.);
#10995=ORIENTED_EDGE('',*,*,#8006,.T.);
#10996=ORIENTED_EDGE('',*,*,#8007,.T.);
#10997=ORIENTED_EDGE('',*,*,#8008,.T.);
#10998=ORIENTED_EDGE('',*,*,#8009,.T.);
#10999=ORIENTED_EDGE('',*,*,#8010,.T.);
#11000=ORIENTED_EDGE('',*,*,#8011,.T.);
#11001=ORIENTED_EDGE('',*,*,#8012,.T.);
#11002=ORIENTED_EDGE('',*,*,#8013,.T.);
#11003=ORIENTED_EDGE('',*,*,#8014,.T.);
#11004=ORIENTED_EDGE('',*,*,#8015,.T.);
#11005=ORIENTED_EDGE('',*,*,#8016,.T.);
#11006=ORIENTED_EDGE('',*,*,#8017,.T.);
#11007=ORIENTED_EDGE('',*,*,#8018,.T.);
#11008=ORIENTED_EDGE('',*,*,#8019,.T.);
#11009=ORIENTED_EDGE('',*,*,#8020,.T.);
#11010=ORIENTED_EDGE('',*,*,#8021,.T.);
#11011=ORIENTED_EDGE('',*,*,#8022,.T.);
#11012=ORIENTED_EDGE('',*,*,#8023,.T.);
#11013=ORIENTED_EDGE('',*,*,#8024,.T.);
#11014=ORIENTED_EDGE('',*,*,#8025,.T.);
#11015=ORIENTED_EDGE('',*,*,#8026,.T.);
#11016=ORIENTED_EDGE('',*,*,#8027,.T.);
#11017=ORIENTED_EDGE('',*,*,#8028,.T.);
#11018=ORIENTED_EDGE('',*,*,#8029,.T.);
#11019=ORIENTED_EDGE('',*,*,#8030,.T.);
#11020=ORIENTED_EDGE('',*,*,#8031,.T.);
#11021=ORIENTED_EDGE('',*,*,#8032,.T.);
#11022=ORIENTED_EDGE('',*,*,#8033,.T.);
#11023=ORIENTED_EDGE('',*,*,#8034,.T.);
#11024=ORIENTED_EDGE('',*,*,#8035,.T.);
#11025=ORIENTED_EDGE('',*,*,#8036,.T.);
#11026=ORIENTED_EDGE('',*,*,#8037,.T.);
#11027=ORIENTED_EDGE('',*,*,#8038,.T.);
#11028=ORIENTED_EDGE('',*,*,#8039,.T.);
#11029=ORIENTED_EDGE('',*,*,#8040,.T.);
#11030=ORIENTED_EDGE('',*,*,#8041,.T.);
#11031=ORIENTED_EDGE('',*,*,#8042,.T.);
#11032=ORIENTED_EDGE('',*,*,#8043,.T.);
#11033=ORIENTED_EDGE('',*,*,#8044,.T.);
#11034=ORIENTED_EDGE('',*,*,#8045,.T.);
#11035=ORIENTED_EDGE('',*,*,#8046,.T.);
#11036=ORIENTED_EDGE('',*,*,#8047,.T.);
#11037=ORIENTED_EDGE('',*,*,#8048,.T.);
#11038=ORIENTED_EDGE('',*,*,#8049,.T.);
#11039=ORIENTED_EDGE('',*,*,#8050,.T.);
#11040=ORIENTED_EDGE('',*,*,#8051,.T.);
#11041=ORIENTED_EDGE('',*,*,#8052,.T.);
#11042=ORIENTED_EDGE('',*,*,#8053,.T.);
#11043=ORIENTED_EDGE('',*,*,#8054,.T.);
#11044=ORIENTED_EDGE('',*,*,#8055,.T.);
#11045=ORIENTED_EDGE('',*,*,#8056,.T.);
#11046=ORIENTED_EDGE('',*,*,#8057,.T.);
#11047=ORIENTED_EDGE('',*,*,#8058,.T.);
#11048=ORIENTED_EDGE('',*,*,#8059,.T.);
#11049=ORIENTED_EDGE('',*,*,#8060,.T.);
#11050=ORIENTED_EDGE('',*,*,#8061,.T.);
#11051=ORIENTED_EDGE('',*,*,#8062,.T.);
#11052=ORIENTED_EDGE('',*,*,#8063,.T.);
#11053=ORIENTED_EDGE('',*,*,#8064,.T.);
#11054=ORIENTED_EDGE('',*,*,#8065,.T.);
#11055=ORIENTED_EDGE('',*,*,#8066,.T.);
#11056=ORIENTED_EDGE('',*,*,#8067,.T.);
#11057=ORIENTED_EDGE('',*,*,#8068,.T.);
#11058=ORIENTED_EDGE('',*,*,#8069,.T.);
#11059=ORIENTED_EDGE('',*,*,#8070,.T.);
#11060=ORIENTED_EDGE('',*,*,#8071,.T.);
#11061=ORIENTED_EDGE('',*,*,#8072,.T.);
#11062=ORIENTED_EDGE('',*,*,#8073,.T.);
#11063=ORIENTED_EDGE('',*,*,#8074,.T.);
#11064=ORIENTED_EDGE('',*,*,#8075,.T.);
#11065=ORIENTED_EDGE('',*,*,#8076,.T.);
#11066=ORIENTED_EDGE('',*,*,#8077,.T.);
#11067=ORIENTED_EDGE('',*,*,#8078,.T.);
#11068=ORIENTED_EDGE('',*,*,#8079,.T.);
#11069=ORIENTED_EDGE('',*,*,#8080,.T.);
#11070=ORIENTED_EDGE('',*,*,#8081,.T.);
#11071=ORIENTED_EDGE('',*,*,#8082,.T.);
#11072=ORIENTED_EDGE('',*,*,#7995,.T.);
#11073=ORIENTED_EDGE('',*,*,#7999,.T.);
#11074=ORIENTED_EDGE('',*,*,#8002,.T.);
#11075=ORIENTED_EDGE('',*,*,#8083,.T.);
#11076=ORIENTED_EDGE('',*,*,#7996,.T.);
#11077=ORIENTED_EDGE('',*,*,#8083,.F.);
#11078=ORIENTED_EDGE('',*,*,#8001,.T.);
#11079=ORIENTED_EDGE('',*,*,#8084,.F.);
#11080=ORIENTED_EDGE('',*,*,#8085,.F.);
#11081=ORIENTED_EDGE('',*,*,#8086,.T.);
#11082=ORIENTED_EDGE('',*,*,#8087,.F.);
#11083=ORIENTED_EDGE('',*,*,#8086,.F.);
#11084=ORIENTED_EDGE('',*,*,#8085,.T.);
#11085=ORIENTED_EDGE('',*,*,#7993,.T.);
#11086=ORIENTED_EDGE('',*,*,#8084,.T.);
#11087=ORIENTED_EDGE('',*,*,#8000,.T.);
#11088=ORIENTED_EDGE('',*,*,#7997,.T.);
#11089=ORIENTED_EDGE('',*,*,#8088,.F.);
#11090=ORIENTED_EDGE('',*,*,#8089,.F.);
#11091=ORIENTED_EDGE('',*,*,#8090,.F.);
#11092=ORIENTED_EDGE('',*,*,#8080,.F.);
#11093=ORIENTED_EDGE('',*,*,#8090,.T.);
#11094=ORIENTED_EDGE('',*,*,#8091,.F.);
#11095=ORIENTED_EDGE('',*,*,#8092,.F.);
#11096=ORIENTED_EDGE('',*,*,#8081,.F.);
#11097=ORIENTED_EDGE('',*,*,#8092,.T.);
#11098=ORIENTED_EDGE('',*,*,#8093,.F.);
#11099=ORIENTED_EDGE('',*,*,#8094,.F.);
#11100=ORIENTED_EDGE('',*,*,#8082,.F.);
#11101=ORIENTED_EDGE('',*,*,#8094,.T.);
#11102=ORIENTED_EDGE('',*,*,#8095,.F.);
#11103=ORIENTED_EDGE('',*,*,#8096,.T.);
#11104=ORIENTED_EDGE('',*,*,#8003,.F.);
#11105=ORIENTED_EDGE('',*,*,#8096,.F.);
#11106=ORIENTED_EDGE('',*,*,#8097,.F.);
#11107=ORIENTED_EDGE('',*,*,#8098,.F.);
#11108=ORIENTED_EDGE('',*,*,#8004,.F.);
#11109=ORIENTED_EDGE('',*,*,#8098,.T.);
#11110=ORIENTED_EDGE('',*,*,#8099,.F.);
#11111=ORIENTED_EDGE('',*,*,#8100,.F.);
#11112=ORIENTED_EDGE('',*,*,#8005,.F.);
#11113=ORIENTED_EDGE('',*,*,#8100,.T.);
#11114=ORIENTED_EDGE('',*,*,#8101,.F.);
#11115=ORIENTED_EDGE('',*,*,#8102,.F.);
#11116=ORIENTED_EDGE('',*,*,#8006,.F.);
#11117=ORIENTED_EDGE('',*,*,#8102,.T.);
#11118=ORIENTED_EDGE('',*,*,#8103,.F.);
#11119=ORIENTED_EDGE('',*,*,#8104,.T.);
#11120=ORIENTED_EDGE('',*,*,#8007,.F.);
#11121=ORIENTED_EDGE('',*,*,#8104,.F.);
#11122=ORIENTED_EDGE('',*,*,#8105,.F.);
#11123=ORIENTED_EDGE('',*,*,#8106,.F.);
#11124=ORIENTED_EDGE('',*,*,#8008,.F.);
#11125=ORIENTED_EDGE('',*,*,#8106,.T.);
#11126=ORIENTED_EDGE('',*,*,#8107,.F.);
#11127=ORIENTED_EDGE('',*,*,#8108,.F.);
#11128=ORIENTED_EDGE('',*,*,#8009,.F.);
#11129=ORIENTED_EDGE('',*,*,#8108,.T.);
#11130=ORIENTED_EDGE('',*,*,#8109,.F.);
#11131=ORIENTED_EDGE('',*,*,#8110,.F.);
#11132=ORIENTED_EDGE('',*,*,#8010,.F.);
#11133=ORIENTED_EDGE('',*,*,#8110,.T.);
#11134=ORIENTED_EDGE('',*,*,#8111,.F.);
#11135=ORIENTED_EDGE('',*,*,#8112,.T.);
#11136=ORIENTED_EDGE('',*,*,#8011,.F.);
#11137=ORIENTED_EDGE('',*,*,#8112,.F.);
#11138=ORIENTED_EDGE('',*,*,#8113,.F.);
#11139=ORIENTED_EDGE('',*,*,#8114,.F.);
#11140=ORIENTED_EDGE('',*,*,#8012,.F.);
#11141=ORIENTED_EDGE('',*,*,#8114,.T.);
#11142=ORIENTED_EDGE('',*,*,#8115,.F.);
#11143=ORIENTED_EDGE('',*,*,#8116,.F.);
#11144=ORIENTED_EDGE('',*,*,#8013,.F.);
#11145=ORIENTED_EDGE('',*,*,#8116,.T.);
#11146=ORIENTED_EDGE('',*,*,#8117,.F.);
#11147=ORIENTED_EDGE('',*,*,#8118,.F.);
#11148=ORIENTED_EDGE('',*,*,#8014,.F.);
#11149=ORIENTED_EDGE('',*,*,#8118,.T.);
#11150=ORIENTED_EDGE('',*,*,#8119,.F.);
#11151=ORIENTED_EDGE('',*,*,#8120,.T.);
#11152=ORIENTED_EDGE('',*,*,#8015,.F.);
#11153=ORIENTED_EDGE('',*,*,#8120,.F.);
#11154=ORIENTED_EDGE('',*,*,#8121,.F.);
#11155=ORIENTED_EDGE('',*,*,#8122,.F.);
#11156=ORIENTED_EDGE('',*,*,#8016,.F.);
#11157=ORIENTED_EDGE('',*,*,#8122,.T.);
#11158=ORIENTED_EDGE('',*,*,#8123,.F.);
#11159=ORIENTED_EDGE('',*,*,#8124,.F.);
#11160=ORIENTED_EDGE('',*,*,#8017,.F.);
#11161=ORIENTED_EDGE('',*,*,#8124,.T.);
#11162=ORIENTED_EDGE('',*,*,#8125,.F.);
#11163=ORIENTED_EDGE('',*,*,#8126,.F.);
#11164=ORIENTED_EDGE('',*,*,#8018,.F.);
#11165=ORIENTED_EDGE('',*,*,#8126,.T.);
#11166=ORIENTED_EDGE('',*,*,#8127,.F.);
#11167=ORIENTED_EDGE('',*,*,#8128,.T.);
#11168=ORIENTED_EDGE('',*,*,#8019,.F.);
#11169=ORIENTED_EDGE('',*,*,#8128,.F.);
#11170=ORIENTED_EDGE('',*,*,#8129,.F.);
#11171=ORIENTED_EDGE('',*,*,#8130,.F.);
#11172=ORIENTED_EDGE('',*,*,#8020,.F.);
#11173=ORIENTED_EDGE('',*,*,#8130,.T.);
#11174=ORIENTED_EDGE('',*,*,#8131,.F.);
#11175=ORIENTED_EDGE('',*,*,#8132,.F.);
#11176=ORIENTED_EDGE('',*,*,#8021,.F.);
#11177=ORIENTED_EDGE('',*,*,#8132,.T.);
#11178=ORIENTED_EDGE('',*,*,#8133,.F.);
#11179=ORIENTED_EDGE('',*,*,#8134,.F.);
#11180=ORIENTED_EDGE('',*,*,#8022,.F.);
#11181=ORIENTED_EDGE('',*,*,#8134,.T.);
#11182=ORIENTED_EDGE('',*,*,#8135,.F.);
#11183=ORIENTED_EDGE('',*,*,#8136,.T.);
#11184=ORIENTED_EDGE('',*,*,#8023,.F.);
#11185=ORIENTED_EDGE('',*,*,#8136,.F.);
#11186=ORIENTED_EDGE('',*,*,#8137,.F.);
#11187=ORIENTED_EDGE('',*,*,#8138,.F.);
#11188=ORIENTED_EDGE('',*,*,#8024,.F.);
#11189=ORIENTED_EDGE('',*,*,#8138,.T.);
#11190=ORIENTED_EDGE('',*,*,#8139,.F.);
#11191=ORIENTED_EDGE('',*,*,#8140,.F.);
#11192=ORIENTED_EDGE('',*,*,#8025,.F.);
#11193=ORIENTED_EDGE('',*,*,#8140,.T.);
#11194=ORIENTED_EDGE('',*,*,#8141,.F.);
#11195=ORIENTED_EDGE('',*,*,#8142,.F.);
#11196=ORIENTED_EDGE('',*,*,#8026,.F.);
#11197=ORIENTED_EDGE('',*,*,#8142,.T.);
#11198=ORIENTED_EDGE('',*,*,#8143,.F.);
#11199=ORIENTED_EDGE('',*,*,#8144,.T.);
#11200=ORIENTED_EDGE('',*,*,#8027,.F.);
#11201=ORIENTED_EDGE('',*,*,#8144,.F.);
#11202=ORIENTED_EDGE('',*,*,#8145,.F.);
#11203=ORIENTED_EDGE('',*,*,#8146,.F.);
#11204=ORIENTED_EDGE('',*,*,#8028,.F.);
#11205=ORIENTED_EDGE('',*,*,#8146,.T.);
#11206=ORIENTED_EDGE('',*,*,#8147,.F.);
#11207=ORIENTED_EDGE('',*,*,#8148,.F.);
#11208=ORIENTED_EDGE('',*,*,#8029,.F.);
#11209=ORIENTED_EDGE('',*,*,#8148,.T.);
#11210=ORIENTED_EDGE('',*,*,#8149,.F.);
#11211=ORIENTED_EDGE('',*,*,#8150,.F.);
#11212=ORIENTED_EDGE('',*,*,#8030,.F.);
#11213=ORIENTED_EDGE('',*,*,#8150,.T.);
#11214=ORIENTED_EDGE('',*,*,#8151,.F.);
#11215=ORIENTED_EDGE('',*,*,#8152,.T.);
#11216=ORIENTED_EDGE('',*,*,#8031,.F.);
#11217=ORIENTED_EDGE('',*,*,#8152,.F.);
#11218=ORIENTED_EDGE('',*,*,#8153,.F.);
#11219=ORIENTED_EDGE('',*,*,#8154,.F.);
#11220=ORIENTED_EDGE('',*,*,#8032,.F.);
#11221=ORIENTED_EDGE('',*,*,#8154,.T.);
#11222=ORIENTED_EDGE('',*,*,#8155,.F.);
#11223=ORIENTED_EDGE('',*,*,#8156,.F.);
#11224=ORIENTED_EDGE('',*,*,#8033,.F.);
#11225=ORIENTED_EDGE('',*,*,#8156,.T.);
#11226=ORIENTED_EDGE('',*,*,#8157,.F.);
#11227=ORIENTED_EDGE('',*,*,#8158,.F.);
#11228=ORIENTED_EDGE('',*,*,#8034,.F.);
#11229=ORIENTED_EDGE('',*,*,#8158,.T.);
#11230=ORIENTED_EDGE('',*,*,#8159,.F.);
#11231=ORIENTED_EDGE('',*,*,#8160,.T.);
#11232=ORIENTED_EDGE('',*,*,#8035,.F.);
#11233=ORIENTED_EDGE('',*,*,#8160,.F.);
#11234=ORIENTED_EDGE('',*,*,#8161,.F.);
#11235=ORIENTED_EDGE('',*,*,#8162,.F.);
#11236=ORIENTED_EDGE('',*,*,#8036,.F.);
#11237=ORIENTED_EDGE('',*,*,#8162,.T.);
#11238=ORIENTED_EDGE('',*,*,#8163,.F.);
#11239=ORIENTED_EDGE('',*,*,#8164,.F.);
#11240=ORIENTED_EDGE('',*,*,#8037,.F.);
#11241=ORIENTED_EDGE('',*,*,#8164,.T.);
#11242=ORIENTED_EDGE('',*,*,#8165,.F.);
#11243=ORIENTED_EDGE('',*,*,#8166,.F.);
#11244=ORIENTED_EDGE('',*,*,#8038,.F.);
#11245=ORIENTED_EDGE('',*,*,#8166,.T.);
#11246=ORIENTED_EDGE('',*,*,#8167,.F.);
#11247=ORIENTED_EDGE('',*,*,#8168,.T.);
#11248=ORIENTED_EDGE('',*,*,#8039,.F.);
#11249=ORIENTED_EDGE('',*,*,#8168,.F.);
#11250=ORIENTED_EDGE('',*,*,#8169,.F.);
#11251=ORIENTED_EDGE('',*,*,#8170,.F.);
#11252=ORIENTED_EDGE('',*,*,#8040,.F.);
#11253=ORIENTED_EDGE('',*,*,#8170,.T.);
#11254=ORIENTED_EDGE('',*,*,#8171,.F.);
#11255=ORIENTED_EDGE('',*,*,#8172,.F.);
#11256=ORIENTED_EDGE('',*,*,#8041,.F.);
#11257=ORIENTED_EDGE('',*,*,#8172,.T.);
#11258=ORIENTED_EDGE('',*,*,#8173,.F.);
#11259=ORIENTED_EDGE('',*,*,#8174,.F.);
#11260=ORIENTED_EDGE('',*,*,#8042,.F.);
#11261=ORIENTED_EDGE('',*,*,#8174,.T.);
#11262=ORIENTED_EDGE('',*,*,#8175,.F.);
#11263=ORIENTED_EDGE('',*,*,#8176,.T.);
#11264=ORIENTED_EDGE('',*,*,#8043,.F.);
#11265=ORIENTED_EDGE('',*,*,#8176,.F.);
#11266=ORIENTED_EDGE('',*,*,#8177,.F.);
#11267=ORIENTED_EDGE('',*,*,#8178,.F.);
#11268=ORIENTED_EDGE('',*,*,#8044,.F.);
#11269=ORIENTED_EDGE('',*,*,#8178,.T.);
#11270=ORIENTED_EDGE('',*,*,#8179,.F.);
#11271=ORIENTED_EDGE('',*,*,#8180,.F.);
#11272=ORIENTED_EDGE('',*,*,#8045,.F.);
#11273=ORIENTED_EDGE('',*,*,#8180,.T.);
#11274=ORIENTED_EDGE('',*,*,#8181,.F.);
#11275=ORIENTED_EDGE('',*,*,#8182,.F.);
#11276=ORIENTED_EDGE('',*,*,#8046,.F.);
#11277=ORIENTED_EDGE('',*,*,#8182,.T.);
#11278=ORIENTED_EDGE('',*,*,#8183,.F.);
#11279=ORIENTED_EDGE('',*,*,#8184,.T.);
#11280=ORIENTED_EDGE('',*,*,#8047,.F.);
#11281=ORIENTED_EDGE('',*,*,#8184,.F.);
#11282=ORIENTED_EDGE('',*,*,#8185,.F.);
#11283=ORIENTED_EDGE('',*,*,#8186,.F.);
#11284=ORIENTED_EDGE('',*,*,#8048,.F.);
#11285=ORIENTED_EDGE('',*,*,#8186,.T.);
#11286=ORIENTED_EDGE('',*,*,#8187,.F.);
#11287=ORIENTED_EDGE('',*,*,#8188,.F.);
#11288=ORIENTED_EDGE('',*,*,#8049,.F.);
#11289=ORIENTED_EDGE('',*,*,#8188,.T.);
#11290=ORIENTED_EDGE('',*,*,#8189,.F.);
#11291=ORIENTED_EDGE('',*,*,#8190,.F.);
#11292=ORIENTED_EDGE('',*,*,#8050,.F.);
#11293=ORIENTED_EDGE('',*,*,#8190,.T.);
#11294=ORIENTED_EDGE('',*,*,#8191,.F.);
#11295=ORIENTED_EDGE('',*,*,#8192,.T.);
#11296=ORIENTED_EDGE('',*,*,#8051,.F.);
#11297=ORIENTED_EDGE('',*,*,#8192,.F.);
#11298=ORIENTED_EDGE('',*,*,#8193,.F.);
#11299=ORIENTED_EDGE('',*,*,#8194,.F.);
#11300=ORIENTED_EDGE('',*,*,#8052,.F.);
#11301=ORIENTED_EDGE('',*,*,#8194,.T.);
#11302=ORIENTED_EDGE('',*,*,#8195,.F.);
#11303=ORIENTED_EDGE('',*,*,#8196,.F.);
#11304=ORIENTED_EDGE('',*,*,#8053,.F.);
#11305=ORIENTED_EDGE('',*,*,#8196,.T.);
#11306=ORIENTED_EDGE('',*,*,#8197,.F.);
#11307=ORIENTED_EDGE('',*,*,#8198,.F.);
#11308=ORIENTED_EDGE('',*,*,#8054,.F.);
#11309=ORIENTED_EDGE('',*,*,#8198,.T.);
#11310=ORIENTED_EDGE('',*,*,#8199,.F.);
#11311=ORIENTED_EDGE('',*,*,#8200,.T.);
#11312=ORIENTED_EDGE('',*,*,#8055,.F.);
#11313=ORIENTED_EDGE('',*,*,#8200,.F.);
#11314=ORIENTED_EDGE('',*,*,#8201,.F.);
#11315=ORIENTED_EDGE('',*,*,#8202,.F.);
#11316=ORIENTED_EDGE('',*,*,#8056,.F.);
#11317=ORIENTED_EDGE('',*,*,#8202,.T.);
#11318=ORIENTED_EDGE('',*,*,#8203,.F.);
#11319=ORIENTED_EDGE('',*,*,#8204,.F.);
#11320=ORIENTED_EDGE('',*,*,#8057,.F.);
#11321=ORIENTED_EDGE('',*,*,#8204,.T.);
#11322=ORIENTED_EDGE('',*,*,#8205,.F.);
#11323=ORIENTED_EDGE('',*,*,#8206,.F.);
#11324=ORIENTED_EDGE('',*,*,#8058,.F.);
#11325=ORIENTED_EDGE('',*,*,#8206,.T.);
#11326=ORIENTED_EDGE('',*,*,#8207,.F.);
#11327=ORIENTED_EDGE('',*,*,#8208,.T.);
#11328=ORIENTED_EDGE('',*,*,#8059,.F.);
#11329=ORIENTED_EDGE('',*,*,#8208,.F.);
#11330=ORIENTED_EDGE('',*,*,#8209,.F.);
#11331=ORIENTED_EDGE('',*,*,#8210,.F.);
#11332=ORIENTED_EDGE('',*,*,#8060,.F.);
#11333=ORIENTED_EDGE('',*,*,#8210,.T.);
#11334=ORIENTED_EDGE('',*,*,#8211,.F.);
#11335=ORIENTED_EDGE('',*,*,#8212,.F.);
#11336=ORIENTED_EDGE('',*,*,#8061,.F.);
#11337=ORIENTED_EDGE('',*,*,#8212,.T.);
#11338=ORIENTED_EDGE('',*,*,#8213,.F.);
#11339=ORIENTED_EDGE('',*,*,#8214,.F.);
#11340=ORIENTED_EDGE('',*,*,#8062,.F.);
#11341=ORIENTED_EDGE('',*,*,#8214,.T.);
#11342=ORIENTED_EDGE('',*,*,#8215,.F.);
#11343=ORIENTED_EDGE('',*,*,#8216,.T.);
#11344=ORIENTED_EDGE('',*,*,#8063,.F.);
#11345=ORIENTED_EDGE('',*,*,#8216,.F.);
#11346=ORIENTED_EDGE('',*,*,#8217,.F.);
#11347=ORIENTED_EDGE('',*,*,#8218,.F.);
#11348=ORIENTED_EDGE('',*,*,#8064,.F.);
#11349=ORIENTED_EDGE('',*,*,#8218,.T.);
#11350=ORIENTED_EDGE('',*,*,#8219,.F.);
#11351=ORIENTED_EDGE('',*,*,#8220,.F.);
#11352=ORIENTED_EDGE('',*,*,#8065,.F.);
#11353=ORIENTED_EDGE('',*,*,#8220,.T.);
#11354=ORIENTED_EDGE('',*,*,#8221,.F.);
#11355=ORIENTED_EDGE('',*,*,#8222,.F.);
#11356=ORIENTED_EDGE('',*,*,#8066,.F.);
#11357=ORIENTED_EDGE('',*,*,#8222,.T.);
#11358=ORIENTED_EDGE('',*,*,#8223,.F.);
#11359=ORIENTED_EDGE('',*,*,#8224,.T.);
#11360=ORIENTED_EDGE('',*,*,#8067,.F.);
#11361=ORIENTED_EDGE('',*,*,#8224,.F.);
#11362=ORIENTED_EDGE('',*,*,#8225,.F.);
#11363=ORIENTED_EDGE('',*,*,#8226,.F.);
#11364=ORIENTED_EDGE('',*,*,#8068,.F.);
#11365=ORIENTED_EDGE('',*,*,#8226,.T.);
#11366=ORIENTED_EDGE('',*,*,#8227,.F.);
#11367=ORIENTED_EDGE('',*,*,#8228,.F.);
#11368=ORIENTED_EDGE('',*,*,#8069,.F.);
#11369=ORIENTED_EDGE('',*,*,#8228,.T.);
#11370=ORIENTED_EDGE('',*,*,#8229,.F.);
#11371=ORIENTED_EDGE('',*,*,#8230,.F.);
#11372=ORIENTED_EDGE('',*,*,#8070,.F.);
#11373=ORIENTED_EDGE('',*,*,#8230,.T.);
#11374=ORIENTED_EDGE('',*,*,#8231,.F.);
#11375=ORIENTED_EDGE('',*,*,#8232,.T.);
#11376=ORIENTED_EDGE('',*,*,#8071,.F.);
#11377=ORIENTED_EDGE('',*,*,#8232,.F.);
#11378=ORIENTED_EDGE('',*,*,#8233,.F.);
#11379=ORIENTED_EDGE('',*,*,#8234,.F.);
#11380=ORIENTED_EDGE('',*,*,#8072,.F.);
#11381=ORIENTED_EDGE('',*,*,#8234,.T.);
#11382=ORIENTED_EDGE('',*,*,#8235,.F.);
#11383=ORIENTED_EDGE('',*,*,#8236,.F.);
#11384=ORIENTED_EDGE('',*,*,#8073,.F.);
#11385=ORIENTED_EDGE('',*,*,#8236,.T.);
#11386=ORIENTED_EDGE('',*,*,#8237,.F.);
#11387=ORIENTED_EDGE('',*,*,#8238,.F.);
#11388=ORIENTED_EDGE('',*,*,#8074,.F.);
#11389=ORIENTED_EDGE('',*,*,#8238,.T.);
#11390=ORIENTED_EDGE('',*,*,#8239,.F.);
#11391=ORIENTED_EDGE('',*,*,#8240,.T.);
#11392=ORIENTED_EDGE('',*,*,#8075,.F.);
#11393=ORIENTED_EDGE('',*,*,#8240,.F.);
#11394=ORIENTED_EDGE('',*,*,#8241,.F.);
#11395=ORIENTED_EDGE('',*,*,#8242,.F.);
#11396=ORIENTED_EDGE('',*,*,#8076,.F.);
#11397=ORIENTED_EDGE('',*,*,#8242,.T.);
#11398=ORIENTED_EDGE('',*,*,#8243,.F.);
#11399=ORIENTED_EDGE('',*,*,#8244,.F.);
#11400=ORIENTED_EDGE('',*,*,#8077,.F.);
#11401=ORIENTED_EDGE('',*,*,#8244,.T.);
#11402=ORIENTED_EDGE('',*,*,#8245,.F.);
#11403=ORIENTED_EDGE('',*,*,#8246,.F.);
#11404=ORIENTED_EDGE('',*,*,#8078,.F.);
#11405=ORIENTED_EDGE('',*,*,#8247,.T.);
#11406=ORIENTED_EDGE('',*,*,#8245,.T.);
#11407=ORIENTED_EDGE('',*,*,#8243,.T.);
#11408=ORIENTED_EDGE('',*,*,#8241,.T.);
#11409=ORIENTED_EDGE('',*,*,#8239,.T.);
#11410=ORIENTED_EDGE('',*,*,#8237,.T.);
#11411=ORIENTED_EDGE('',*,*,#8235,.T.);
#11412=ORIENTED_EDGE('',*,*,#8233,.T.);
#11413=ORIENTED_EDGE('',*,*,#8231,.T.);
#11414=ORIENTED_EDGE('',*,*,#8229,.T.);
#11415=ORIENTED_EDGE('',*,*,#8227,.T.);
#11416=ORIENTED_EDGE('',*,*,#8225,.T.);
#11417=ORIENTED_EDGE('',*,*,#8223,.T.);
#11418=ORIENTED_EDGE('',*,*,#8221,.T.);
#11419=ORIENTED_EDGE('',*,*,#8219,.T.);
#11420=ORIENTED_EDGE('',*,*,#8217,.T.);
#11421=ORIENTED_EDGE('',*,*,#8215,.T.);
#11422=ORIENTED_EDGE('',*,*,#8213,.T.);
#11423=ORIENTED_EDGE('',*,*,#8211,.T.);
#11424=ORIENTED_EDGE('',*,*,#8209,.T.);
#11425=ORIENTED_EDGE('',*,*,#8207,.T.);
#11426=ORIENTED_EDGE('',*,*,#8205,.T.);
#11427=ORIENTED_EDGE('',*,*,#8203,.T.);
#11428=ORIENTED_EDGE('',*,*,#8201,.T.);
#11429=ORIENTED_EDGE('',*,*,#8199,.T.);
#11430=ORIENTED_EDGE('',*,*,#8197,.T.);
#11431=ORIENTED_EDGE('',*,*,#8195,.T.);
#11432=ORIENTED_EDGE('',*,*,#8193,.T.);
#11433=ORIENTED_EDGE('',*,*,#8191,.T.);
#11434=ORIENTED_EDGE('',*,*,#8189,.T.);
#11435=ORIENTED_EDGE('',*,*,#8187,.T.);
#11436=ORIENTED_EDGE('',*,*,#8185,.T.);
#11437=ORIENTED_EDGE('',*,*,#8183,.T.);
#11438=ORIENTED_EDGE('',*,*,#8181,.T.);
#11439=ORIENTED_EDGE('',*,*,#8179,.T.);
#11440=ORIENTED_EDGE('',*,*,#8177,.T.);
#11441=ORIENTED_EDGE('',*,*,#8175,.T.);
#11442=ORIENTED_EDGE('',*,*,#8173,.T.);
#11443=ORIENTED_EDGE('',*,*,#8171,.T.);
#11444=ORIENTED_EDGE('',*,*,#8169,.T.);
#11445=ORIENTED_EDGE('',*,*,#8167,.T.);
#11446=ORIENTED_EDGE('',*,*,#8165,.T.);
#11447=ORIENTED_EDGE('',*,*,#8163,.T.);
#11448=ORIENTED_EDGE('',*,*,#8161,.T.);
#11449=ORIENTED_EDGE('',*,*,#8159,.T.);
#11450=ORIENTED_EDGE('',*,*,#8157,.T.);
#11451=ORIENTED_EDGE('',*,*,#8155,.T.);
#11452=ORIENTED_EDGE('',*,*,#8153,.T.);
#11453=ORIENTED_EDGE('',*,*,#8151,.T.);
#11454=ORIENTED_EDGE('',*,*,#8149,.T.);
#11455=ORIENTED_EDGE('',*,*,#8147,.T.);
#11456=ORIENTED_EDGE('',*,*,#8145,.T.);
#11457=ORIENTED_EDGE('',*,*,#8143,.T.);
#11458=ORIENTED_EDGE('',*,*,#8141,.T.);
#11459=ORIENTED_EDGE('',*,*,#8139,.T.);
#11460=ORIENTED_EDGE('',*,*,#8137,.T.);
#11461=ORIENTED_EDGE('',*,*,#8135,.T.);
#11462=ORIENTED_EDGE('',*,*,#8133,.T.);
#11463=ORIENTED_EDGE('',*,*,#8131,.T.);
#11464=ORIENTED_EDGE('',*,*,#8129,.T.);
#11465=ORIENTED_EDGE('',*,*,#8127,.T.);
#11466=ORIENTED_EDGE('',*,*,#8125,.T.);
#11467=ORIENTED_EDGE('',*,*,#8123,.T.);
#11468=ORIENTED_EDGE('',*,*,#8121,.T.);
#11469=ORIENTED_EDGE('',*,*,#8119,.T.);
#11470=ORIENTED_EDGE('',*,*,#8117,.T.);
#11471=ORIENTED_EDGE('',*,*,#8115,.T.);
#11472=ORIENTED_EDGE('',*,*,#8113,.T.);
#11473=ORIENTED_EDGE('',*,*,#8111,.T.);
#11474=ORIENTED_EDGE('',*,*,#8109,.T.);
#11475=ORIENTED_EDGE('',*,*,#8107,.T.);
#11476=ORIENTED_EDGE('',*,*,#8105,.T.);
#11477=ORIENTED_EDGE('',*,*,#8103,.T.);
#11478=ORIENTED_EDGE('',*,*,#8101,.T.);
#11479=ORIENTED_EDGE('',*,*,#8099,.T.);
#11480=ORIENTED_EDGE('',*,*,#8097,.T.);
#11481=ORIENTED_EDGE('',*,*,#8095,.T.);
#11482=ORIENTED_EDGE('',*,*,#8093,.T.);
#11483=ORIENTED_EDGE('',*,*,#8091,.T.);
#11484=ORIENTED_EDGE('',*,*,#8089,.T.);
#11485=ORIENTED_EDGE('',*,*,#8087,.T.);
#11486=ORIENTED_EDGE('',*,*,#8088,.T.);
#11487=ORIENTED_EDGE('',*,*,#8079,.F.);
#11488=ORIENTED_EDGE('',*,*,#8246,.T.);
#11489=ORIENTED_EDGE('',*,*,#8247,.F.);
#11772=CYLINDRICAL_SURFACE('',#13949,0.6);
#11773=CYLINDRICAL_SURFACE('',#13951,1.4);
#11774=CYLINDRICAL_SURFACE('',#13956,1.75);
#11775=CYLINDRICAL_SURFACE('',#13959,1.75);
#11776=CYLINDRICAL_SURFACE('',#13962,1.75);
#11777=CYLINDRICAL_SURFACE('',#13965,1.75);
#11778=CYLINDRICAL_SURFACE('',#13968,1.75);
#11779=CYLINDRICAL_SURFACE('',#13971,1.75);
#11780=CYLINDRICAL_SURFACE('',#13974,1.75);
#11781=CYLINDRICAL_SURFACE('',#13977,1.75);
#11782=CYLINDRICAL_SURFACE('',#13980,1.75);
#11783=CYLINDRICAL_SURFACE('',#13983,1.75);
#11784=CYLINDRICAL_SURFACE('',#13986,1.75);
#11785=CYLINDRICAL_SURFACE('',#13989,1.75);
#11786=CYLINDRICAL_SURFACE('',#13992,1.75);
#11787=CYLINDRICAL_SURFACE('',#13995,1.75);
#11788=CYLINDRICAL_SURFACE('',#13998,1.75);
#11789=CYLINDRICAL_SURFACE('',#14001,1.75);
#11790=CYLINDRICAL_SURFACE('',#14004,1.75);
#11791=CYLINDRICAL_SURFACE('',#14007,1.75);
#11792=CYLINDRICAL_SURFACE('',#14010,1.75);
#11793=CYLINDRICAL_SURFACE('',#14015,1.75);
#12353=ADVANCED_FACE('',(#1844),#1241,.F.);
#12354=ADVANCED_FACE('',(#1845),#1242,.F.);
#12355=ADVANCED_FACE('',(#1846),#1243,.F.);
#12356=ADVANCED_FACE('',(#1847,#840),#1244,.F.);
#12357=ADVANCED_FACE('',(#1848),#11772,.F.);
#12358=ADVANCED_FACE('',(#1849),#11773,.T.);
#12359=ADVANCED_FACE('',(#1850,#841),#1245,.T.);
#12360=ADVANCED_FACE('',(#1851),#11,.T.);
#12361=ADVANCED_FACE('',(#1852),#1246,.T.);
#12362=ADVANCED_FACE('',(#1853),#12,.T.);
#12363=ADVANCED_FACE('',(#1854),#11774,.T.);
#12364=ADVANCED_FACE('',(#1855),#13,.T.);
#12365=ADVANCED_FACE('',(#1856),#1247,.T.);
#12366=ADVANCED_FACE('',(#1857),#14,.T.);
#12367=ADVANCED_FACE('',(#1858),#11775,.T.);
#12368=ADVANCED_FACE('',(#1859),#15,.T.);
#12369=ADVANCED_FACE('',(#1860),#1248,.T.);
#12370=ADVANCED_FACE('',(#1861),#16,.T.);
#12371=ADVANCED_FACE('',(#1862),#11776,.T.);
#12372=ADVANCED_FACE('',(#1863),#17,.T.);
#12373=ADVANCED_FACE('',(#1864),#1249,.T.);
#12374=ADVANCED_FACE('',(#1865),#18,.T.);
#12375=ADVANCED_FACE('',(#1866),#11777,.T.);
#12376=ADVANCED_FACE('',(#1867),#19,.T.);
#12377=ADVANCED_FACE('',(#1868),#1250,.T.);
#12378=ADVANCED_FACE('',(#1869),#20,.T.);
#12379=ADVANCED_FACE('',(#1870),#11778,.T.);
#12380=ADVANCED_FACE('',(#1871),#21,.T.);
#12381=ADVANCED_FACE('',(#1872),#1251,.T.);
#12382=ADVANCED_FACE('',(#1873),#22,.T.);
#12383=ADVANCED_FACE('',(#1874),#11779,.T.);
#12384=ADVANCED_FACE('',(#1875),#23,.T.);
#12385=ADVANCED_FACE('',(#1876),#1252,.T.);
#12386=ADVANCED_FACE('',(#1877),#24,.T.);
#12387=ADVANCED_FACE('',(#1878),#11780,.T.);
#12388=ADVANCED_FACE('',(#1879),#25,.T.);
#12389=ADVANCED_FACE('',(#1880),#1253,.T.);
#12390=ADVANCED_FACE('',(#1881),#26,.T.);
#12391=ADVANCED_FACE('',(#1882),#11781,.T.);
#12392=ADVANCED_FACE('',(#1883),#27,.T.);
#12393=ADVANCED_FACE('',(#1884),#1254,.T.);
#12394=ADVANCED_FACE('',(#1885),#28,.T.);
#12395=ADVANCED_FACE('',(#1886),#11782,.T.);
#12396=ADVANCED_FACE('',(#1887),#29,.T.);
#12397=ADVANCED_FACE('',(#1888),#1255,.T.);
#12398=ADVANCED_FACE('',(#1889),#30,.T.);
#12399=ADVANCED_FACE('',(#1890),#11783,.T.);
#12400=ADVANCED_FACE('',(#1891),#31,.T.);
#12401=ADVANCED_FACE('',(#1892),#1256,.T.);
#12402=ADVANCED_FACE('',(#1893),#32,.T.);
#12403=ADVANCED_FACE('',(#1894),#11784,.T.);
#12404=ADVANCED_FACE('',(#1895),#33,.T.);
#12405=ADVANCED_FACE('',(#1896),#1257,.T.);
#12406=ADVANCED_FACE('',(#1897),#34,.T.);
#12407=ADVANCED_FACE('',(#1898),#11785,.T.);
#12408=ADVANCED_FACE('',(#1899),#35,.T.);
#12409=ADVANCED_FACE('',(#1900),#1258,.T.);
#12410=ADVANCED_FACE('',(#1901),#36,.T.);
#12411=ADVANCED_FACE('',(#1902),#11786,.T.);
#12412=ADVANCED_FACE('',(#1903),#37,.T.);
#12413=ADVANCED_FACE('',(#1904),#1259,.T.);
#12414=ADVANCED_FACE('',(#1905),#38,.T.);
#12415=ADVANCED_FACE('',(#1906),#11787,.T.);
#12416=ADVANCED_FACE('',(#1907),#39,.T.);
#12417=ADVANCED_FACE('',(#1908),#1260,.T.);
#12418=ADVANCED_FACE('',(#1909),#40,.T.);
#12419=ADVANCED_FACE('',(#1910),#11788,.T.);
#12420=ADVANCED_FACE('',(#1911),#41,.T.);
#12421=ADVANCED_FACE('',(#1912),#1261,.T.);
#12422=ADVANCED_FACE('',(#1913),#42,.T.);
#12423=ADVANCED_FACE('',(#1914),#11789,.T.);
#12424=ADVANCED_FACE('',(#1915),#43,.T.);
#12425=ADVANCED_FACE('',(#1916),#1262,.T.);
#12426=ADVANCED_FACE('',(#1917),#44,.T.);
#12427=ADVANCED_FACE('',(#1918),#11790,.T.);
#12428=ADVANCED_FACE('',(#1919),#45,.T.);
#12429=ADVANCED_FACE('',(#1920),#1263,.T.);
#12430=ADVANCED_FACE('',(#1921),#46,.T.);
#12431=ADVANCED_FACE('',(#1922),#11791,.T.);
#12432=ADVANCED_FACE('',(#1923),#47,.T.);
#12433=ADVANCED_FACE('',(#1924),#1264,.T.);
#12434=ADVANCED_FACE('',(#1925),#48,.T.);
#12435=ADVANCED_FACE('',(#1926),#11792,.T.);
#12436=ADVANCED_FACE('',(#1927),#49,.T.);
#12437=ADVANCED_FACE('',(#1928),#1265,.T.);
#12438=ADVANCED_FACE('',(#1929),#50,.T.);
#12439=ADVANCED_FACE('',(#1930,#842),#1266,.T.);
#12440=ADVANCED_FACE('',(#1931),#11793,.T.);
#12529=CLOSED_SHELL('',(#12353,#12354,#12355,#12356,#12357,#12358,#12359,
#12360,#12361,#12362,#12363,#12364,#12365,#12366,#12367,#12368,#12369,#12370,
#12371,#12372,#12373,#12374,#12375,#12376,#12377,#12378,#12379,#12380,#12381,
#12382,#12383,#12384,#12385,#12386,#12387,#12388,#12389,#12390,#12391,#12392,
#12393,#12394,#12395,#12396,#12397,#12398,#12399,#12400,#12401,#12402,#12403,
#12404,#12405,#12406,#12407,#12408,#12409,#12410,#12411,#12412,#12413,#12414,
#12415,#12416,#12417,#12418,#12419,#12420,#12421,#12422,#12423,#12424,#12425,
#12426,#12427,#12428,#12429,#12430,#12431,#12432,#12433,#12434,#12435,#12436,
#12437,#12438,#12439,#12440));
#13923=AXIS2_PLACEMENT_3D('',#20821,#16991,#16992);
#13924=AXIS2_PLACEMENT_3D('',#20822,#16993,#16994);
#13925=AXIS2_PLACEMENT_3D('',#20831,#16999,#17000);
#13926=AXIS2_PLACEMENT_3D('',#20837,#17004,#17005);
#13927=AXIS2_PLACEMENT_3D('',#20843,#17009,#17010);
#13928=AXIS2_PLACEMENT_3D('',#20846,#17011,#17012);
#13929=AXIS2_PLACEMENT_3D('',#20992,#17014,#17015);
#13930=AXIS2_PLACEMENT_3D('',#21138,#17017,#17018);
#13931=AXIS2_PLACEMENT_3D('',#21284,#17020,#17021);
#13932=AXIS2_PLACEMENT_3D('',#21430,#17023,#17024);
#13933=AXIS2_PLACEMENT_3D('',#21576,#17026,#17027);
#13934=AXIS2_PLACEMENT_3D('',#21722,#17029,#17030);
#13935=AXIS2_PLACEMENT_3D('',#21868,#17032,#17033);
#13936=AXIS2_PLACEMENT_3D('',#22014,#17035,#17036);
#13937=AXIS2_PLACEMENT_3D('',#22160,#17038,#17039);
#13938=AXIS2_PLACEMENT_3D('',#22306,#17041,#17042);
#13939=AXIS2_PLACEMENT_3D('',#22452,#17044,#17045);
#13940=AXIS2_PLACEMENT_3D('',#22598,#17047,#17048);
#13941=AXIS2_PLACEMENT_3D('',#22744,#17050,#17051);
#13942=AXIS2_PLACEMENT_3D('',#22890,#17053,#17054);
#13943=AXIS2_PLACEMENT_3D('',#23036,#17056,#17057);
#13944=AXIS2_PLACEMENT_3D('',#23182,#17059,#17060);
#13945=AXIS2_PLACEMENT_3D('',#23328,#17062,#17063);
#13946=AXIS2_PLACEMENT_3D('',#23474,#17065,#17066);
#13947=AXIS2_PLACEMENT_3D('',#23620,#17068,#17069);
#13948=AXIS2_PLACEMENT_3D('',#23764,#17071,#17072);
#13949=AXIS2_PLACEMENT_3D('',#23765,#17073,#17074);
#13950=AXIS2_PLACEMENT_3D('',#23766,#17075,#17076);
#13951=AXIS2_PLACEMENT_3D('',#23767,#17077,#17078);
#13952=AXIS2_PLACEMENT_3D('',#23769,#17079,#17080);
#13953=AXIS2_PLACEMENT_3D('',#23772,#17082,#17083);
#13954=AXIS2_PLACEMENT_3D('',#23773,#17084,#17085);
#13955=AXIS2_PLACEMENT_3D('',#23988,#17088,#17089);
#13956=AXIS2_PLACEMENT_3D('',#24204,#17093,#17094);
#13957=AXIS2_PLACEMENT_3D('',#24206,#17095,#17096);
#13958=AXIS2_PLACEMENT_3D('',#24420,#17099,#17100);
#13959=AXIS2_PLACEMENT_3D('',#24636,#17104,#17105);
#13960=AXIS2_PLACEMENT_3D('',#24638,#17106,#17107);
#13961=AXIS2_PLACEMENT_3D('',#24852,#17110,#17111);
#13962=AXIS2_PLACEMENT_3D('',#25068,#17115,#17116);
#13963=AXIS2_PLACEMENT_3D('',#25070,#17117,#17118);
#13964=AXIS2_PLACEMENT_3D('',#25284,#17121,#17122);
#13965=AXIS2_PLACEMENT_3D('',#25500,#17126,#17127);
#13966=AXIS2_PLACEMENT_3D('',#25502,#17128,#17129);
#13967=AXIS2_PLACEMENT_3D('',#25716,#17132,#17133);
#13968=AXIS2_PLACEMENT_3D('',#25932,#17137,#17138);
#13969=AXIS2_PLACEMENT_3D('',#25934,#17139,#17140);
#13970=AXIS2_PLACEMENT_3D('',#26148,#17143,#17144);
#13971=AXIS2_PLACEMENT_3D('',#26364,#17148,#17149);
#13972=AXIS2_PLACEMENT_3D('',#26366,#17150,#17151);
#13973=AXIS2_PLACEMENT_3D('',#26580,#17154,#17155);
#13974=AXIS2_PLACEMENT_3D('',#26796,#17159,#17160);
#13975=AXIS2_PLACEMENT_3D('',#26798,#17161,#17162);
#13976=AXIS2_PLACEMENT_3D('',#27012,#17165,#17166);
#13977=AXIS2_PLACEMENT_3D('',#27228,#17170,#17171);
#13978=AXIS2_PLACEMENT_3D('',#27230,#17172,#17173);
#13979=AXIS2_PLACEMENT_3D('',#27444,#17176,#17177);
#13980=AXIS2_PLACEMENT_3D('',#27660,#17181,#17182);
#13981=AXIS2_PLACEMENT_3D('',#27662,#17183,#17184);
#13982=AXIS2_PLACEMENT_3D('',#27876,#17187,#17188);
#13983=AXIS2_PLACEMENT_3D('',#28092,#17192,#17193);
#13984=AXIS2_PLACEMENT_3D('',#28094,#17194,#17195);
#13985=AXIS2_PLACEMENT_3D('',#28308,#17198,#17199);
#13986=AXIS2_PLACEMENT_3D('',#28524,#17203,#17204);
#13987=AXIS2_PLACEMENT_3D('',#28526,#17205,#17206);
#13988=AXIS2_PLACEMENT_3D('',#28740,#17209,#17210);
#13989=AXIS2_PLACEMENT_3D('',#28956,#17214,#17215);
#13990=AXIS2_PLACEMENT_3D('',#28958,#17216,#17217);
#13991=AXIS2_PLACEMENT_3D('',#29172,#17220,#17221);
#13992=AXIS2_PLACEMENT_3D('',#29388,#17225,#17226);
#13993=AXIS2_PLACEMENT_3D('',#29390,#17227,#17228);
#13994=AXIS2_PLACEMENT_3D('',#29604,#17231,#17232);
#13995=AXIS2_PLACEMENT_3D('',#29820,#17236,#17237);
#13996=AXIS2_PLACEMENT_3D('',#29822,#17238,#17239);
#13997=AXIS2_PLACEMENT_3D('',#30036,#17242,#17243);
#13998=AXIS2_PLACEMENT_3D('',#30252,#17247,#17248);
#13999=AXIS2_PLACEMENT_3D('',#30254,#17249,#17250);
#14000=AXIS2_PLACEMENT_3D('',#30468,#17253,#17254);
#14001=AXIS2_PLACEMENT_3D('',#30684,#17258,#17259);
#14002=AXIS2_PLACEMENT_3D('',#30686,#17260,#17261);
#14003=AXIS2_PLACEMENT_3D('',#30900,#17264,#17265);
#14004=AXIS2_PLACEMENT_3D('',#31116,#17269,#17270);
#14005=AXIS2_PLACEMENT_3D('',#31118,#17271,#17272);
#14006=AXIS2_PLACEMENT_3D('',#31332,#17275,#17276);
#14007=AXIS2_PLACEMENT_3D('',#31548,#17280,#17281);
#14008=AXIS2_PLACEMENT_3D('',#31550,#17282,#17283);
#14009=AXIS2_PLACEMENT_3D('',#31764,#17286,#17287);
#14010=AXIS2_PLACEMENT_3D('',#31980,#17291,#17292);
#14011=AXIS2_PLACEMENT_3D('',#31982,#17293,#17294);
#14012=AXIS2_PLACEMENT_3D('',#32196,#17297,#17298);
#14013=AXIS2_PLACEMENT_3D('',#32412,#17302,#17303);
#14014=AXIS2_PLACEMENT_3D('',#32413,#17304,#17305);
#14015=AXIS2_PLACEMENT_3D('',#32414,#17306,#17307);
#16991=DIRECTION('axis',(0.,0.,1.));
#16992=DIRECTION('refdir',(1.,0.,0.));
#16993=DIRECTION('center_axis',(1.,0.,0.));
#16994=DIRECTION('ref_axis',(0.,0.,-1.));
#16995=DIRECTION('',(0.,0.,1.));
#16996=DIRECTION('',(0.,1.,0.));
#16997=DIRECTION('',(0.,0.,-1.));
#16998=DIRECTION('',(0.,-1.,0.));
#16999=DIRECTION('center_axis',(0.,0.,-1.));
#17000=DIRECTION('ref_axis',(-1.,0.,0.));
#17001=DIRECTION('',(1.,0.,0.));
#17002=DIRECTION('',(0.,-1.,0.));
#17003=DIRECTION('',(-1.,0.,0.));
#17004=DIRECTION('center_axis',(-1.,0.,0.));
#17005=DIRECTION('ref_axis',(0.,0.,1.));
#17006=DIRECTION('',(0.,0.,-1.));
#17007=DIRECTION('',(0.,1.,0.));
#17008=DIRECTION('',(0.,0.,1.));
#17009=DIRECTION('center_axis',(0.,1.,0.));
#17010=DIRECTION('ref_axis',(1.,0.,0.));
#17011=DIRECTION('center_axis',(0.,-1.,0.));
#17012=DIRECTION('ref_axis',(1.,0.,0.));
#17013=DIRECTION('',(-0.587785252292473,0.,0.809016994374947));
#17014=DIRECTION('center_axis',(0.,-1.,0.));
#17015=DIRECTION('ref_axis',(1.,0.,0.));
#17016=DIRECTION('',(-0.809016994374948,0.,0.587785252292473));
#17017=DIRECTION('center_axis',(0.,-1.,0.));
#17018=DIRECTION('ref_axis',(1.,0.,0.));
#17019=DIRECTION('',(-0.951056516295154,0.,0.309016994374947));
#17020=DIRECTION('center_axis',(0.,-1.,0.));
#17021=DIRECTION('ref_axis',(1.,0.,0.));
#17022=DIRECTION('',(-1.,0.,-1.83697019872103E-16));
#17023=DIRECTION('center_axis',(0.,-1.,0.));
#17024=DIRECTION('ref_axis',(1.,0.,0.));
#17025=DIRECTION('',(-0.951056516295154,0.,-0.309016994374948));
#17026=DIRECTION('center_axis',(0.,-1.,0.));
#17027=DIRECTION('ref_axis',(1.,0.,0.));
#17028=DIRECTION('',(-0.809016994374947,0.,-0.587785252292473));
#17029=DIRECTION('center_axis',(0.,-1.,0.));
#17030=DIRECTION('ref_axis',(1.,0.,0.));
#17031=DIRECTION('',(-0.587785252292473,0.,-0.809016994374948));
#17032=DIRECTION('center_axis',(0.,-1.,0.));
#17033=DIRECTION('ref_axis',(1.,0.,0.));
#17034=DIRECTION('',(-0.309016994374947,0.,-0.951056516295154));
#17035=DIRECTION('center_axis',(0.,-1.,0.));
#17036=DIRECTION('ref_axis',(1.,0.,0.));
#17037=DIRECTION('',(1.22464679914735E-16,0.,-1.));
#17038=DIRECTION('center_axis',(0.,-1.,0.));
#17039=DIRECTION('ref_axis',(1.,0.,0.));
#17040=DIRECTION('',(0.309016994374948,0.,-0.951056516295154));
#17041=DIRECTION('center_axis',(0.,-1.,0.));
#17042=DIRECTION('ref_axis',(1.,0.,0.));
#17043=DIRECTION('',(0.587785252292473,0.,-0.809016994374947));
#17044=DIRECTION('center_axis',(0.,-1.,0.));
#17045=DIRECTION('ref_axis',(1.,0.,0.));
#17046=DIRECTION('',(0.809016994374948,0.,-0.587785252292473));
#17047=DIRECTION('center_axis',(0.,-1.,0.));
#17048=DIRECTION('ref_axis',(1.,0.,0.));
#17049=DIRECTION('',(0.951056516295154,0.,-0.309016994374947));
#17050=DIRECTION('center_axis',(0.,-1.,0.));
#17051=DIRECTION('ref_axis',(1.,0.,0.));
#17052=DIRECTION('',(1.,0.,6.12323399573677E-17));
#17053=DIRECTION('center_axis',(0.,-1.,0.));
#17054=DIRECTION('ref_axis',(1.,0.,0.));
#17055=DIRECTION('',(0.951056516295154,0.,0.309016994374948));
#17056=DIRECTION('center_axis',(0.,-1.,0.));
#17057=DIRECTION('ref_axis',(1.,0.,0.));
#17058=DIRECTION('',(0.809016994374947,0.,0.587785252292473));
#17059=DIRECTION('center_axis',(0.,-1.,0.));
#17060=DIRECTION('ref_axis',(1.,0.,0.));
#17061=DIRECTION('',(0.587785252292473,0.,0.809016994374947));
#17062=DIRECTION('center_axis',(0.,-1.,0.));
#17063=DIRECTION('ref_axis',(1.,0.,0.));
#17064=DIRECTION('',(0.309016994374947,0.,0.951056516295154));
#17065=DIRECTION('center_axis',(0.,-1.,0.));
#17066=DIRECTION('ref_axis',(1.,0.,0.));
#17067=DIRECTION('',(0.,0.,1.));
#17068=DIRECTION('center_axis',(0.,-1.,0.));
#17069=DIRECTION('ref_axis',(1.,0.,0.));
#17070=DIRECTION('',(-0.309016994374948,0.,0.951056516295154));
#17071=DIRECTION('center_axis',(0.,1.,0.));
#17072=DIRECTION('ref_axis',(1.,0.,0.));
#17073=DIRECTION('center_axis',(0.,1.,0.));
#17074=DIRECTION('ref_axis',(6.12323399573677E-17,0.,1.));
#17075=DIRECTION('center_axis',(0.,-1.,0.));
#17076=DIRECTION('ref_axis',(1.,0.,0.));
#17077=DIRECTION('center_axis',(0.,1.,0.));
#17078=DIRECTION('ref_axis',(1.,0.,0.));
#17079=DIRECTION('center_axis',(0.,1.,0.));
#17080=DIRECTION('ref_axis',(1.,0.,0.));
#17081=DIRECTION('',(0.,-1.,0.));
#17082=DIRECTION('center_axis',(0.,-1.,0.));
#17083=DIRECTION('ref_axis',(1.,0.,0.));
#17084=DIRECTION('center_axis',(0.,1.,0.));
#17085=DIRECTION('ref_axis',(1.,0.,0.));
#17086=DIRECTION('',(0.,-1.,0.));
#17087=DIRECTION('',(0.,1.,0.));
#17088=DIRECTION('center_axis',(0.951056516295154,0.,0.309016994374948));
#17089=DIRECTION('ref_axis',(0.309016994374948,0.,-0.951056516295154));
#17090=DIRECTION('',(0.309016994374948,0.,-0.951056516295154));
#17091=DIRECTION('',(0.,1.,0.));
#17092=DIRECTION('',(0.,1.,0.));
#17093=DIRECTION('center_axis',(0.,1.,0.));
#17094=DIRECTION('ref_axis',(1.,0.,0.));
#17095=DIRECTION('center_axis',(0.,1.,0.));
#17096=DIRECTION('ref_axis',(1.,0.,0.));
#17097=DIRECTION('',(0.,-1.,0.));
#17098=DIRECTION('',(0.,1.,0.));
#17099=DIRECTION('center_axis',(0.809016994374947,0.,0.587785252292473));
#17100=DIRECTION('ref_axis',(0.587785252292473,0.,-0.809016994374947));
#17101=DIRECTION('',(0.587785252292473,0.,-0.809016994374947));
#17102=DIRECTION('',(0.,1.,0.));
#17103=DIRECTION('',(0.,1.,0.));
#17104=DIRECTION('center_axis',(0.,1.,0.));
#17105=DIRECTION('ref_axis',(1.,0.,0.));
#17106=DIRECTION('center_axis',(0.,1.,0.));
#17107=DIRECTION('ref_axis',(1.,0.,0.));
#17108=DIRECTION('',(0.,-1.,0.));
#17109=DIRECTION('',(0.,1.,0.));
#17110=DIRECTION('center_axis',(0.587785252292473,0.,0.809016994374948));
#17111=DIRECTION('ref_axis',(0.809016994374948,0.,-0.587785252292473));
#17112=DIRECTION('',(0.809016994374948,0.,-0.587785252292473));
#17113=DIRECTION('',(0.,1.,0.));
#17114=DIRECTION('',(0.,1.,0.));
#17115=DIRECTION('center_axis',(0.,1.,0.));
#17116=DIRECTION('ref_axis',(1.,0.,0.));
#17117=DIRECTION('center_axis',(0.,1.,0.));
#17118=DIRECTION('ref_axis',(1.,0.,0.));
#17119=DIRECTION('',(0.,-1.,0.));
#17120=DIRECTION('',(0.,1.,0.));
#17121=DIRECTION('center_axis',(0.309016994374947,0.,0.951056516295154));
#17122=DIRECTION('ref_axis',(0.951056516295154,0.,-0.309016994374947));
#17123=DIRECTION('',(0.951056516295154,0.,-0.309016994374947));
#17124=DIRECTION('',(0.,1.,0.));
#17125=DIRECTION('',(0.,1.,0.));
#17126=DIRECTION('center_axis',(0.,1.,0.));
#17127=DIRECTION('ref_axis',(1.,0.,0.));
#17128=DIRECTION('center_axis',(0.,1.,0.));
#17129=DIRECTION('ref_axis',(1.,0.,0.));
#17130=DIRECTION('',(0.,-1.,0.));
#17131=DIRECTION('',(0.,1.,0.));
#17132=DIRECTION('center_axis',(-1.83697019872103E-16,0.,1.));
#17133=DIRECTION('ref_axis',(1.,0.,1.83697019872103E-16));
#17134=DIRECTION('',(1.,0.,1.83697019872103E-16));
#17135=DIRECTION('',(0.,1.,0.));
#17136=DIRECTION('',(0.,1.,0.));
#17137=DIRECTION('center_axis',(0.,1.,0.));
#17138=DIRECTION('ref_axis',(1.,0.,0.));
#17139=DIRECTION('center_axis',(0.,1.,0.));
#17140=DIRECTION('ref_axis',(1.,0.,0.));
#17141=DIRECTION('',(0.,-1.,0.));
#17142=DIRECTION('',(0.,1.,0.));
#17143=DIRECTION('center_axis',(-0.309016994374948,0.,0.951056516295154));
#17144=DIRECTION('ref_axis',(0.951056516295154,0.,0.309016994374948));
#17145=DIRECTION('',(0.951056516295154,0.,0.309016994374948));
#17146=DIRECTION('',(0.,1.,0.));
#17147=DIRECTION('',(0.,1.,0.));
#17148=DIRECTION('center_axis',(0.,1.,0.));
#17149=DIRECTION('ref_axis',(1.,0.,0.));
#17150=DIRECTION('center_axis',(0.,1.,0.));
#17151=DIRECTION('ref_axis',(1.,0.,0.));
#17152=DIRECTION('',(0.,-1.,0.));
#17153=DIRECTION('',(0.,1.,0.));
#17154=DIRECTION('center_axis',(-0.587785252292473,0.,0.809016994374947));
#17155=DIRECTION('ref_axis',(0.809016994374947,0.,0.587785252292473));
#17156=DIRECTION('',(0.809016994374947,0.,0.587785252292473));
#17157=DIRECTION('',(0.,1.,0.));
#17158=DIRECTION('',(0.,1.,0.));
#17159=DIRECTION('center_axis',(0.,1.,0.));
#17160=DIRECTION('ref_axis',(1.,0.,0.));
#17161=DIRECTION('center_axis',(0.,1.,0.));
#17162=DIRECTION('ref_axis',(1.,0.,0.));
#17163=DIRECTION('',(0.,-1.,0.));
#17164=DIRECTION('',(0.,1.,0.));
#17165=DIRECTION('center_axis',(-0.809016994374948,0.,0.587785252292473));
#17166=DIRECTION('ref_axis',(0.587785252292473,0.,0.809016994374948));
#17167=DIRECTION('',(0.587785252292473,0.,0.809016994374948));
#17168=DIRECTION('',(0.,1.,0.));
#17169=DIRECTION('',(0.,1.,0.));
#17170=DIRECTION('center_axis',(0.,1.,0.));
#17171=DIRECTION('ref_axis',(1.,0.,0.));
#17172=DIRECTION('center_axis',(0.,1.,0.));
#17173=DIRECTION('ref_axis',(1.,0.,0.));
#17174=DIRECTION('',(0.,-1.,0.));
#17175=DIRECTION('',(0.,1.,0.));
#17176=DIRECTION('center_axis',(-0.951056516295154,0.,0.309016994374947));
#17177=DIRECTION('ref_axis',(0.309016994374947,0.,0.951056516295154));
#17178=DIRECTION('',(0.309016994374947,0.,0.951056516295154));
#17179=DIRECTION('',(0.,1.,0.));
#17180=DIRECTION('',(0.,1.,0.));
#17181=DIRECTION('center_axis',(0.,1.,0.));
#17182=DIRECTION('ref_axis',(1.,0.,0.));
#17183=DIRECTION('center_axis',(0.,1.,0.));
#17184=DIRECTION('ref_axis',(1.,0.,0.));
#17185=DIRECTION('',(0.,-1.,0.));
#17186=DIRECTION('',(0.,1.,0.));
#17187=DIRECTION('center_axis',(-1.,0.,-1.22464679914735E-16));
#17188=DIRECTION('ref_axis',(-1.22464679914735E-16,0.,1.));
#17189=DIRECTION('',(-1.22464679914735E-16,0.,1.));
#17190=DIRECTION('',(0.,1.,0.));
#17191=DIRECTION('',(0.,1.,0.));
#17192=DIRECTION('center_axis',(0.,1.,0.));
#17193=DIRECTION('ref_axis',(1.,0.,0.));
#17194=DIRECTION('center_axis',(0.,1.,0.));
#17195=DIRECTION('ref_axis',(1.,0.,0.));
#17196=DIRECTION('',(0.,-1.,0.));
#17197=DIRECTION('',(0.,1.,0.));
#17198=DIRECTION('center_axis',(-0.951056516295154,0.,-0.309016994374948));
#17199=DIRECTION('ref_axis',(-0.309016994374948,0.,0.951056516295154));
#17200=DIRECTION('',(-0.309016994374948,0.,0.951056516295154));
#17201=DIRECTION('',(0.,1.,0.));
#17202=DIRECTION('',(0.,1.,0.));
#17203=DIRECTION('center_axis',(0.,1.,0.));
#17204=DIRECTION('ref_axis',(1.,0.,0.));
#17205=DIRECTION('center_axis',(0.,1.,0.));
#17206=DIRECTION('ref_axis',(1.,0.,0.));
#17207=DIRECTION('',(0.,-1.,0.));
#17208=DIRECTION('',(0.,1.,0.));
#17209=DIRECTION('center_axis',(-0.809016994374947,0.,-0.587785252292473));
#17210=DIRECTION('ref_axis',(-0.587785252292473,0.,0.809016994374947));
#17211=DIRECTION('',(-0.587785252292473,0.,0.809016994374947));
#17212=DIRECTION('',(0.,1.,0.));
#17213=DIRECTION('',(0.,1.,0.));
#17214=DIRECTION('center_axis',(0.,1.,0.));
#17215=DIRECTION('ref_axis',(1.,0.,0.));
#17216=DIRECTION('center_axis',(0.,1.,0.));
#17217=DIRECTION('ref_axis',(1.,0.,0.));
#17218=DIRECTION('',(0.,-1.,0.));
#17219=DIRECTION('',(0.,1.,0.));
#17220=DIRECTION('center_axis',(-0.587785252292473,0.,-0.809016994374948));
#17221=DIRECTION('ref_axis',(-0.809016994374948,0.,0.587785252292473));
#17222=DIRECTION('',(-0.809016994374948,0.,0.587785252292473));
#17223=DIRECTION('',(0.,1.,0.));
#17224=DIRECTION('',(0.,1.,0.));
#17225=DIRECTION('center_axis',(0.,1.,0.));
#17226=DIRECTION('ref_axis',(1.,0.,0.));
#17227=DIRECTION('center_axis',(0.,1.,0.));
#17228=DIRECTION('ref_axis',(1.,0.,0.));
#17229=DIRECTION('',(0.,-1.,0.));
#17230=DIRECTION('',(0.,1.,0.));
#17231=DIRECTION('center_axis',(-0.309016994374947,0.,-0.951056516295154));
#17232=DIRECTION('ref_axis',(-0.951056516295154,0.,0.309016994374947));
#17233=DIRECTION('',(-0.951056516295154,0.,0.309016994374947));
#17234=DIRECTION('',(0.,1.,0.));
#17235=DIRECTION('',(0.,1.,0.));
#17236=DIRECTION('center_axis',(0.,1.,0.));
#17237=DIRECTION('ref_axis',(1.,0.,0.));
#17238=DIRECTION('center_axis',(0.,1.,0.));
#17239=DIRECTION('ref_axis',(1.,0.,0.));
#17240=DIRECTION('',(0.,-1.,0.));
#17241=DIRECTION('',(0.,1.,0.));
#17242=DIRECTION('center_axis',(6.12323399573677E-17,0.,-1.));
#17243=DIRECTION('ref_axis',(-1.,0.,-6.12323399573677E-17));
#17244=DIRECTION('',(-1.,0.,-6.12323399573677E-17));
#17245=DIRECTION('',(0.,1.,0.));
#17246=DIRECTION('',(0.,1.,0.));
#17247=DIRECTION('center_axis',(0.,1.,0.));
#17248=DIRECTION('ref_axis',(1.,0.,0.));
#17249=DIRECTION('center_axis',(0.,1.,0.));
#17250=DIRECTION('ref_axis',(1.,0.,0.));
#17251=DIRECTION('',(0.,-1.,0.));
#17252=DIRECTION('',(0.,1.,0.));
#17253=DIRECTION('center_axis',(0.309016994374948,0.,-0.951056516295154));
#17254=DIRECTION('ref_axis',(-0.951056516295154,0.,-0.309016994374948));
#17255=DIRECTION('',(-0.951056516295154,0.,-0.309016994374948));
#17256=DIRECTION('',(0.,1.,0.));
#17257=DIRECTION('',(0.,1.,0.));
#17258=DIRECTION('center_axis',(0.,1.,0.));
#17259=DIRECTION('ref_axis',(1.,0.,0.));
#17260=DIRECTION('center_axis',(0.,1.,0.));
#17261=DIRECTION('ref_axis',(1.,0.,0.));
#17262=DIRECTION('',(0.,-1.,0.));
#17263=DIRECTION('',(0.,1.,0.));
#17264=DIRECTION('center_axis',(0.587785252292473,0.,-0.809016994374947));
#17265=DIRECTION('ref_axis',(-0.809016994374947,0.,-0.587785252292473));
#17266=DIRECTION('',(-0.809016994374947,0.,-0.587785252292473));
#17267=DIRECTION('',(0.,1.,0.));
#17268=DIRECTION('',(0.,1.,0.));
#17269=DIRECTION('center_axis',(0.,1.,0.));
#17270=DIRECTION('ref_axis',(1.,0.,0.));
#17271=DIRECTION('center_axis',(0.,1.,0.));
#17272=DIRECTION('ref_axis',(1.,0.,0.));
#17273=DIRECTION('',(0.,-1.,0.));
#17274=DIRECTION('',(0.,1.,0.));
#17275=DIRECTION('center_axis',(0.809016994374947,0.,-0.587785252292473));
#17276=DIRECTION('ref_axis',(-0.587785252292473,0.,-0.809016994374947));
#17277=DIRECTION('',(-0.587785252292473,0.,-0.809016994374947));
#17278=DIRECTION('',(0.,1.,0.));
#17279=DIRECTION('',(0.,1.,0.));
#17280=DIRECTION('center_axis',(0.,1.,0.));
#17281=DIRECTION('ref_axis',(1.,0.,0.));
#17282=DIRECTION('center_axis',(0.,1.,0.));
#17283=DIRECTION('ref_axis',(1.,0.,0.));
#17284=DIRECTION('',(0.,-1.,0.));
#17285=DIRECTION('',(0.,1.,0.));
#17286=DIRECTION('center_axis',(0.951056516295154,0.,-0.309016994374947));
#17287=DIRECTION('ref_axis',(-0.309016994374947,0.,-0.951056516295154));
#17288=DIRECTION('',(-0.309016994374947,0.,-0.951056516295154));
#17289=DIRECTION('',(0.,1.,0.));
#17290=DIRECTION('',(0.,1.,0.));
#17291=DIRECTION('center_axis',(0.,1.,0.));
#17292=DIRECTION('ref_axis',(1.,0.,0.));
#17293=DIRECTION('center_axis',(0.,1.,0.));
#17294=DIRECTION('ref_axis',(1.,0.,0.));
#17295=DIRECTION('',(0.,-1.,0.));
#17296=DIRECTION('',(0.,1.,0.));
#17297=DIRECTION('center_axis',(1.,0.,0.));
#17298=DIRECTION('ref_axis',(0.,0.,-1.));
#17299=DIRECTION('',(0.,0.,-1.));
#17300=DIRECTION('',(0.,1.,0.));
#17301=DIRECTION('',(0.,1.,0.));
#17302=DIRECTION('center_axis',(0.,1.,0.));
#17303=DIRECTION('ref_axis',(1.,0.,0.));
#17304=DIRECTION('center_axis',(0.,1.,0.));
#17305=DIRECTION('ref_axis',(1.,0.,0.));
#17306=DIRECTION('center_axis',(0.,1.,0.));
#17307=DIRECTION('ref_axis',(1.,0.,0.));
#20821=CARTESIAN_POINT('',(0.,0.,0.));
#20822=CARTESIAN_POINT('Origin',(0.2,0.,0.));
#20823=CARTESIAN_POINT('',(0.2,2.2,-0.78));
#20824=CARTESIAN_POINT('',(0.2,2.2,-0.565685424949238));
#20825=CARTESIAN_POINT('',(0.2,2.2,0.));
#20826=CARTESIAN_POINT('',(0.2,-1.,-0.78));
#20827=CARTESIAN_POINT('',(0.2,0.,-0.78));
#20828=CARTESIAN_POINT('',(0.2,-1.,-0.565685424949238));
#20829=CARTESIAN_POINT('',(0.2,-1.,0.));
#20830=CARTESIAN_POINT('',(0.2,0.,-0.565685424949238));
#20831=CARTESIAN_POINT('Origin',(0.2,0.,-0.78));
#20832=CARTESIAN_POINT('',(-0.2,2.2,-0.78));
#20833=CARTESIAN_POINT('',(0.1,2.2,-0.78));
#20834=CARTESIAN_POINT('',(-0.2,-1.,-0.78));
#20835=CARTESIAN_POINT('',(-0.2,0.,-0.78));
#20836=CARTESIAN_POINT('',(0.1,-1.,-0.78));
#20837=CARTESIAN_POINT('Origin',(-0.2,0.,-0.78));
#20838=CARTESIAN_POINT('',(-0.2,2.2,-0.565685424949238));
#20839=CARTESIAN_POINT('',(-0.2,2.2,-0.39));
#20840=CARTESIAN_POINT('',(-0.2,-1.,-0.565685424949238));
#20841=CARTESIAN_POINT('',(-0.2,0.,-0.565685424949238));
#20842=CARTESIAN_POINT('',(-0.2,-1.,-0.39));
#20843=CARTESIAN_POINT('Origin',(0.,-1.,0.));
#20844=CARTESIAN_POINT('',(1.60662857109684,-1.,0.693717979106306));
#20845=CARTESIAN_POINT('',(1.5055822144029,-1.,0.892032620296856));
#20846=CARTESIAN_POINT('Origin',(0.,-1.,0.));
#20847=CARTESIAN_POINT('',(1.81978687191668,-1.,1.23627494547115));
#20848=CARTESIAN_POINT('Ctrl Pts',(1.5055822144029,-1.,0.892032620296856));
#20849=CARTESIAN_POINT('Ctrl Pts',(1.50980486806688,-1.,0.894452006964544));
#20850=CARTESIAN_POINT('Ctrl Pts',(1.51805569590094,-1.,0.899185047483511));
#20851=CARTESIAN_POINT('Ctrl Pts',(1.52984849887993,-1.,0.905967409625651));
#20852=CARTESIAN_POINT('Ctrl Pts',(1.54440491149498,-1.,0.914375919026456));
#20853=CARTESIAN_POINT('Ctrl Pts',(1.56065988578893,-1.,0.923832188944341));
#20854=CARTESIAN_POINT('Ctrl Pts',(1.57499388382243,-1.,0.932246680108685));
#20855=CARTESIAN_POINT('Ctrl Pts',(1.58744937487176,-1.,0.939646377893399));
#20856=CARTESIAN_POINT('Ctrl Pts',(1.59810042043673,-1.,0.946078063315257));
#20857=CARTESIAN_POINT('Ctrl Pts',(1.60706069896936,-1.,0.951613284356035));
#20858=CARTESIAN_POINT('Ctrl Pts',(1.61449324337085,-1.,0.956354422920671));
#20859=CARTESIAN_POINT('Ctrl Pts',(1.62061638140221,-1.,0.960438326101729));
#20860=CARTESIAN_POINT('Ctrl Pts',(1.62571930670187,-1.,0.964046107040536));
#20861=CARTESIAN_POINT('Ctrl Pts',(1.63013849959461,-1.,0.967387853230345));
#20862=CARTESIAN_POINT('Ctrl Pts',(1.63420665729798,-1.,0.970669715997509));
#20863=CARTESIAN_POINT('Ctrl Pts',(1.63820952658144,-1.,0.974066058287419));
#20864=CARTESIAN_POINT('Ctrl Pts',(1.64233990826687,-1.,0.977689794119417));
#20865=CARTESIAN_POINT('Ctrl Pts',(1.64665139190656,-1.,0.981562530939489));
#20866=CARTESIAN_POINT('Ctrl Pts',(1.65110016612638,-1.,0.985642622920821));
#20867=CARTESIAN_POINT('Ctrl Pts',(1.65559044289699,-1.,0.989855627854165));
#20868=CARTESIAN_POINT('Ctrl Pts',(1.66001553809947,-1.,0.994121836661306));
#20869=CARTESIAN_POINT('Ctrl Pts',(1.66430758030376,-1.,0.998389654952758));
#20870=CARTESIAN_POINT('Ctrl Pts',(1.66846059277303,-1.,1.00265091003727));
#20871=CARTESIAN_POINT('Ctrl Pts',(1.67250335383293,-1.,1.00692206696414));
#20872=CARTESIAN_POINT('Ctrl Pts',(1.67648246776464,-1.,1.01123236493511));
#20873=CARTESIAN_POINT('Ctrl Pts',(1.68044289894798,-1.,1.01561026162773));
#20874=CARTESIAN_POINT('Ctrl Pts',(1.68440578021706,-1.,1.02006795074201));
#20875=CARTESIAN_POINT('Ctrl Pts',(1.68836910178447,-1.,1.02460180535255));
#20876=CARTESIAN_POINT('Ctrl Pts',(1.69231840863458,-1.,1.02919977579147));
#20877=CARTESIAN_POINT('Ctrl Pts',(1.69623414782771,-1.,1.03384646003588));
#20878=CARTESIAN_POINT('Ctrl Pts',(1.70010052930962,-1.,1.03852922490789));
#20879=CARTESIAN_POINT('Ctrl Pts',(1.70391338707982,-1.,1.04324363334554));
#20880=CARTESIAN_POINT('Ctrl Pts',(1.70767646263649,-1.,1.04799085404995));
#20881=CARTESIAN_POINT('Ctrl Pts',(1.71139783543989,-1.,1.05277517202855));
#20882=CARTESIAN_POINT('Ctrl Pts',(1.7150865442702,-1.,1.05760163192479));
#20883=CARTESIAN_POINT('Ctrl Pts',(1.71874858456904,-1.,1.06247324680647));
#20884=CARTESIAN_POINT('Ctrl Pts',(1.72238500928453,-1.,1.06738966975462));
#20885=CARTESIAN_POINT('Ctrl Pts',(1.72599406198488,-1.,1.07234866990252));
#20886=CARTESIAN_POINT('Ctrl Pts',(1.72957248977424,-1.,1.0773470373727));
#20887=CARTESIAN_POINT('Ctrl Pts',(1.73311705663407,-1.,1.08238162784749));
#20888=CARTESIAN_POINT('Ctrl Pts',(1.73662628326091,-1.,1.08745056285427));
#20889=CARTESIAN_POINT('Ctrl Pts',(1.74010053962247,-1.,1.09255329056493));
#20890=CARTESIAN_POINT('Ctrl Pts',(1.74354119236208,-1.,1.09768999241226));
#20891=CARTESIAN_POINT('Ctrl Pts',(1.74695004214923,-1.,1.10286118991143));
#20892=CARTESIAN_POINT('Ctrl Pts',(1.7503286607592,-1.,1.10806728183007));
#20893=CARTESIAN_POINT('Ctrl Pts',(1.7536777209463,-1.,1.11330807582551));
#20894=CARTESIAN_POINT('Ctrl Pts',(1.75699720772105,-1.,1.11858293216763));
#20895=CARTESIAN_POINT('Ctrl Pts',(1.76028671825096,-1.,1.12389096855086));
#20896=CARTESIAN_POINT('Ctrl Pts',(1.7635457196617,-1.,1.12923123555075));
#20897=CARTESIAN_POINT('Ctrl Pts',(1.76677384551862,-1.,1.1346029180462));
#20898=CARTESIAN_POINT('Ctrl Pts',(1.76997111386769,-1.,1.14000548336975));
#20899=CARTESIAN_POINT('Ctrl Pts',(1.77313777896194,-1.,1.1454385822692));
#20900=CARTESIAN_POINT('Ctrl Pts',(1.7762742255701,-1.,1.15090197841515));
#20901=CARTESIAN_POINT('Ctrl Pts',(1.77938085564275,-1.,1.15639547194698));
#20902=CARTESIAN_POINT('Ctrl Pts',(1.78245795881009,-1.,1.16191881298499));
#20903=CARTESIAN_POINT('Ctrl Pts',(1.78550566040443,-1.,1.16747166312303));
#20904=CARTESIAN_POINT('Ctrl Pts',(1.78852398877616,-1.,1.17305363177328));
#20905=CARTESIAN_POINT('Ctrl Pts',(1.79151291552689,-1.,1.17866429440809));
#20906=CARTESIAN_POINT('Ctrl Pts',(1.79447240321515,-1.,1.18430321697432));
#20907=CARTESIAN_POINT('Ctrl Pts',(1.79740245923478,-1.,1.18996997934445));
#20908=CARTESIAN_POINT('Ctrl Pts',(1.80030314369879,-1.,1.19566418930242));
#20909=CARTESIAN_POINT('Ctrl Pts',(1.80317454838603,-1.,1.20138548938974));
#20910=CARTESIAN_POINT('Ctrl Pts',(1.80601678480707,-1.,1.20713356605475));
#20911=CARTESIAN_POINT('Ctrl Pts',(1.80882996917129,-1.,1.21290815708314));
#20912=CARTESIAN_POINT('Ctrl Pts',(1.81161420806656,-1.,1.21870906103557));
#20913=CARTESIAN_POINT('Ctrl Pts',(1.81436959210434,-1.,1.2245361330495));
#20914=CARTESIAN_POINT('Ctrl Pts',(1.8165508718364,-1.,1.2292186489137));
#20915=CARTESIAN_POINT('Ctrl Pts',(1.81817389921279,-1.,1.2327422452705));
#20916=CARTESIAN_POINT('Ctrl Pts',(1.81925017193666,-1.,1.23509651170476));
#20917=CARTESIAN_POINT('Ctrl Pts',(1.81978687191668,-1.,1.23627494547115));
#20918=CARTESIAN_POINT('',(1.73811241238545,-1.,1.34869019493419));
#20919=CARTESIAN_POINT('',(1.81978687191668,-1.,1.23627494547115));
#20920=CARTESIAN_POINT('',(1.31362392696032,-1.,1.15624053661742));
#20921=CARTESIAN_POINT('Ctrl Pts',(1.73811241238545,-1.,1.34869019493419));
#20922=CARTESIAN_POINT('Ctrl Pts',(1.73682580585691,-1.,1.34854391898045));
#20923=CARTESIAN_POINT('Ctrl Pts',(1.73425417885907,-1.,1.34824783112887));
#20924=CARTESIAN_POINT('Ctrl Pts',(1.7304014965394,-1.,1.34779309152035));
#20925=CARTESIAN_POINT('Ctrl Pts',(1.72527410680674,-1.,1.34716554819527));
#20926=CARTESIAN_POINT('Ctrl Pts',(1.7188807715049,-1.,1.34634568653227));
#20927=CARTESIAN_POINT('Ctrl Pts',(1.71250340686822,-1.,1.34549029589416));
#20928=CARTESIAN_POINT('Ctrl Pts',(1.70614212266738,-1.,1.34459924533831));
#20929=CARTESIAN_POINT('Ctrl Pts',(1.69979707754427,-1.,1.34367237124483));
#20930=CARTESIAN_POINT('Ctrl Pts',(1.6934684849687,-1.,1.34270948206319));
#20931=CARTESIAN_POINT('Ctrl Pts',(1.68715660868764,-1.,1.341710374848));
#20932=CARTESIAN_POINT('Ctrl Pts',(1.68086176030362,-1.,1.34067485185203));
#20933=CARTESIAN_POINT('Ctrl Pts',(1.67458429426086,-1.,1.3396027347034));
#20934=CARTESIAN_POINT('Ctrl Pts',(1.66832460783989,-1.,1.33849388654388));
#20935=CARTESIAN_POINT('Ctrl Pts',(1.66208312541983,-1.,1.33734820885262));
#20936=CARTESIAN_POINT('Ctrl Pts',(1.65586025952593,-1.,1.33616559745172));
#20937=CARTESIAN_POINT('Ctrl Pts',(1.6496563728683,-1.,1.33494590467993));
#20938=CARTESIAN_POINT('Ctrl Pts',(1.6434717485603,-1.,1.33368890676572));
#20939=CARTESIAN_POINT('Ctrl Pts',(1.63730653475089,-1.,1.33239425103724));
#20940=CARTESIAN_POINT('Ctrl Pts',(1.63116079730923,-1.,1.33106149345645));
#20941=CARTESIAN_POINT('Ctrl Pts',(1.62503464209797,-1.,1.3296901950568));
#20942=CARTESIAN_POINT('Ctrl Pts',(1.61892832270724,-1.,1.32828000610449));
#20943=CARTESIAN_POINT('Ctrl Pts',(1.6128423401575,-1.,1.32683074483356));
#20944=CARTESIAN_POINT('Ctrl Pts',(1.60677758290954,-1.,1.32534250785782));
#20945=CARTESIAN_POINT('Ctrl Pts',(1.60073511858687,-1.,1.32381550858256));
#20946=CARTESIAN_POINT('Ctrl Pts',(1.59471591079403,-1.,1.32224985747682));
#20947=CARTESIAN_POINT('Ctrl Pts',(1.58872057258245,-1.,1.32064537110892));
#20948=CARTESIAN_POINT('Ctrl Pts',(1.58274907898834,-1.,1.31900135021432));
#20949=CARTESIAN_POINT('Ctrl Pts',(1.5768005650559,-1.,1.31731642317187));
#20950=CARTESIAN_POINT('Ctrl Pts',(1.57087397835723,-1.,1.31558903860016));
#20951=CARTESIAN_POINT('Ctrl Pts',(1.56496872402353,-1.,1.31381795281002));
#20952=CARTESIAN_POINT('Ctrl Pts',(1.55908521254821,-1.,1.31200264341696));
#20953=CARTESIAN_POINT('Ctrl Pts',(1.55322568759481,-1.,1.31014393684222));
#20954=CARTESIAN_POINT('Ctrl Pts',(1.54739413957185,-1.,1.30824393907473));
#20955=CARTESIAN_POINT('Ctrl Pts',(1.54159462645432,-1.,1.30630475189556));
#20956=CARTESIAN_POINT('Ctrl Pts',(1.53582981268977,-1.,1.30432735639489));
#20957=CARTESIAN_POINT('Ctrl Pts',(1.53009970283891,-1.,1.30231064395568));
#20958=CARTESIAN_POINT('Ctrl Pts',(1.52439957861062,-1.,1.30024984366328));
#20959=CARTESIAN_POINT('Ctrl Pts',(1.51872184912724,-1.,1.29813791800747));
#20960=CARTESIAN_POINT('Ctrl Pts',(1.51305994241402,-1.,1.29596850710509));
#20961=CARTESIAN_POINT('Ctrl Pts',(1.50741159078365,-1.,1.29373841372842));
#20962=CARTESIAN_POINT('Ctrl Pts',(1.50178230149776,-1.,1.29145022885181));
#20963=CARTESIAN_POINT('Ctrl Pts',(1.49618896881754,-1.,1.28911506584254));
#20964=CARTESIAN_POINT('Ctrl Pts',(1.4906522831278,-1.,1.2867467611644));
#20965=CARTESIAN_POINT('Ctrl Pts',(1.4851881711891,-1.,1.28435533880201));
#20966=CARTESIAN_POINT('Ctrl Pts',(1.47980070347095,-1.,1.28194158939517));
#20967=CARTESIAN_POINT('Ctrl Pts',(1.4744717526707,-1.,1.2794891824849));
#20968=CARTESIAN_POINT('Ctrl Pts',(1.46916035917133,-1.,1.2769641483109));
#20969=CARTESIAN_POINT('Ctrl Pts',(1.46382431332476,-1.,1.27433119897822));
#20970=CARTESIAN_POINT('Ctrl Pts',(1.45843906294697,-1.,1.27156805265289));
#20971=CARTESIAN_POINT('Ctrl Pts',(1.45301422764247,-1.,1.2686778680489));
#20972=CARTESIAN_POINT('Ctrl Pts',(1.44761985001662,-1.,1.26570925118868));
#20973=CARTESIAN_POINT('Ctrl Pts',(1.44236470511303,-1.,1.26273903323859));
#20974=CARTESIAN_POINT('Ctrl Pts',(1.43734919180847,-1.,1.25983531012005));
#20975=CARTESIAN_POINT('Ctrl Pts',(1.43262645609691,-1.,1.25702687965755));
#20976=CARTESIAN_POINT('Ctrl Pts',(1.42815938799387,-1.,1.25426945222639));
#20977=CARTESIAN_POINT('Ctrl Pts',(1.42378102115575,-1.,1.2514145557001));
#20978=CARTESIAN_POINT('Ctrl Pts',(1.41923722596025,-1.,1.24824430986571));
#20979=CARTESIAN_POINT('Ctrl Pts',(1.41422913175179,-1.,1.24450600513056));
#20980=CARTESIAN_POINT('Ctrl Pts',(1.40845295531283,-1.,1.23994455029534));
#20981=CARTESIAN_POINT('Ctrl Pts',(1.40164708206106,-1.,1.23434087290423));
#20982=CARTESIAN_POINT('Ctrl Pts',(1.39361389568796,-1.,1.22752961899387));
#20983=CARTESIAN_POINT('Ctrl Pts',(1.38420564527715,-1.,1.21938737280852));
#20984=CARTESIAN_POINT('Ctrl Pts',(1.37331915607905,-1.,1.20982812925645));
#20985=CARTESIAN_POINT('Ctrl Pts',(1.36088705043885,-1.,1.1987959077932));
#20986=CARTESIAN_POINT('Ctrl Pts',(1.34687054001093,-1.,1.18625865667441));
#20987=CARTESIAN_POINT('Ctrl Pts',(1.33437539347008,-1.,1.17501305789857));
#20988=CARTESIAN_POINT('Ctrl Pts',(1.32428080721772,-1.,1.16589330093588));
#20989=CARTESIAN_POINT('Ctrl Pts',(1.31722977216397,-1.,1.15950888730809));
#20990=CARTESIAN_POINT('Ctrl Pts',(1.31362392696032,-1.,1.15624053661742));
#20991=CARTESIAN_POINT('',(1.15624053661742,-1.,1.31362392696033));
#20992=CARTESIAN_POINT('Origin',(0.,-1.,0.));
#20993=CARTESIAN_POINT('',(1.34869019493419,-1.,1.73811241238545));
#20994=CARTESIAN_POINT('Ctrl Pts',(1.15624053661742,-1.,1.31362392696033));
#20995=CARTESIAN_POINT('Ctrl Pts',(1.15950888730433,-1.,1.3172297721596));
#20996=CARTESIAN_POINT('Ctrl Pts',(1.16589330092532,-1.,1.32428080720544));
#20997=CARTESIAN_POINT('Ctrl Pts',(1.17501305787994,-1.,1.33437539344842));
#20998=CARTESIAN_POINT('Ctrl Pts',(1.18625865664915,-1.,1.34687053998157));
#20999=CARTESIAN_POINT('Ctrl Pts',(1.1987959077656,-1.,1.36088705040677));
#21000=CARTESIAN_POINT('Ctrl Pts',(1.20982812923113,-1.,1.37331915604962));
#21001=CARTESIAN_POINT('Ctrl Pts',(1.21938737278853,-1.,1.38420564525391));
#21002=CARTESIAN_POINT('Ctrl Pts',(1.22752961898063,-1.,1.39361389567257));
#21003=CARTESIAN_POINT('Ctrl Pts',(1.23434087289768,-1.,1.40164708205345));
#21004=CARTESIAN_POINT('Ctrl Pts',(1.23994455029421,-1.,1.40845295531151));
#21005=CARTESIAN_POINT('Ctrl Pts',(1.24450600513278,-1.,1.41422913175437));
#21006=CARTESIAN_POINT('Ctrl Pts',(1.24824430986911,-1.,1.41923722596421));
#21007=CARTESIAN_POINT('Ctrl Pts',(1.25141455570299,-1.,1.42378102115911));
#21008=CARTESIAN_POINT('Ctrl Pts',(1.25426945222783,-1.,1.42815938799555));
#21009=CARTESIAN_POINT('Ctrl Pts',(1.25702687965744,-1.,1.43262645609679));
#21010=CARTESIAN_POINT('Ctrl Pts',(1.25983531011894,-1.,1.43734919180719));
#21011=CARTESIAN_POINT('Ctrl Pts',(1.26273903323723,-1.,1.44236470511145));
#21012=CARTESIAN_POINT('Ctrl Pts',(1.26570925118767,-1.,1.44761985001544));
#21013=CARTESIAN_POINT('Ctrl Pts',(1.26867786804854,-1.,1.45301422764205));
#21014=CARTESIAN_POINT('Ctrl Pts',(1.27156805265312,-1.,1.45843906294725));
#21015=CARTESIAN_POINT('Ctrl Pts',(1.27433119897877,-1.,1.4638243133254));
#21016=CARTESIAN_POINT('Ctrl Pts',(1.27696414831144,-1.,1.46916035917197));
#21017=CARTESIAN_POINT('Ctrl Pts',(1.27948918248524,-1.,1.4744717526711));
#21018=CARTESIAN_POINT('Ctrl Pts',(1.28194158939522,-1.,1.47980070347102));
#21019=CARTESIAN_POINT('Ctrl Pts',(1.28435533880184,-1.,1.48518817118891));
#21020=CARTESIAN_POINT('Ctrl Pts',(1.28674676116415,-1.,1.4906522831275));
#21021=CARTESIAN_POINT('Ctrl Pts',(1.28911506584232,-1.,1.49618896881729));
#21022=CARTESIAN_POINT('Ctrl Pts',(1.29145022885171,-1.,1.50178230149764));
#21023=CARTESIAN_POINT('Ctrl Pts',(1.29373841372843,-1.,1.50741159078367));
#21024=CARTESIAN_POINT('Ctrl Pts',(1.29596850710518,-1.,1.51305994241412));
#21025=CARTESIAN_POINT('Ctrl Pts',(1.29813791800757,-1.,1.51872184912735));
#21026=CARTESIAN_POINT('Ctrl Pts',(1.30024984366334,-1.,1.5243995786107));
#21027=CARTESIAN_POINT('Ctrl Pts',(1.3023106439557,-1.,1.53009970283893));
#21028=CARTESIAN_POINT('Ctrl Pts',(1.30432735639487,-1.,1.53582981268976));
#21029=CARTESIAN_POINT('Ctrl Pts',(1.30630475189553,-1.,1.54159462645428));
#21030=CARTESIAN_POINT('Ctrl Pts',(1.30824393907471,-1.,1.54739413957183));
#21031=CARTESIAN_POINT('Ctrl Pts',(1.31014393684221,-1.,1.55322568759481));
#21032=CARTESIAN_POINT('Ctrl Pts',(1.31200264341696,-1.,1.55908521254822));
#21033=CARTESIAN_POINT('Ctrl Pts',(1.31381795281002,-1.,1.56496872402352));
#21034=CARTESIAN_POINT('Ctrl Pts',(1.31558903860015,-1.,1.57087397835721));
#21035=CARTESIAN_POINT('Ctrl Pts',(1.31731642317183,-1.,1.57680056505585));
#21036=CARTESIAN_POINT('Ctrl Pts',(1.31900135021428,-1.,1.58274907898829));
#21037=CARTESIAN_POINT('Ctrl Pts',(1.32064537110891,-1.,1.58872057258244));
#21038=CARTESIAN_POINT('Ctrl Pts',(1.32224985747686,-1.,1.59471591079408));
#21039=CARTESIAN_POINT('Ctrl Pts',(1.32381550858266,-1.,1.600735118587));
#21040=CARTESIAN_POINT('Ctrl Pts',(1.32534250785794,-1.,1.6067775829097));
#21041=CARTESIAN_POINT('Ctrl Pts',(1.32683074483365,-1.,1.61284234015762));
#21042=CARTESIAN_POINT('Ctrl Pts',(1.32828000610448,-1.,1.61892832270723));
#21043=CARTESIAN_POINT('Ctrl Pts',(1.32969019505665,-1.,1.62503464209777));
#21044=CARTESIAN_POINT('Ctrl Pts',(1.33106149345618,-1.,1.63116079730887));
#21045=CARTESIAN_POINT('Ctrl Pts',(1.33239425103694,-1.,1.6373065347505));
#21046=CARTESIAN_POINT('Ctrl Pts',(1.33368890676554,-1.,1.64347174856007));
#21047=CARTESIAN_POINT('Ctrl Pts',(1.33494590468003,-1.,1.64965637286843));
#21048=CARTESIAN_POINT('Ctrl Pts',(1.33616559745217,-1.,1.65586025952651));
#21049=CARTESIAN_POINT('Ctrl Pts',(1.33734820885331,-1.,1.66208312542073));
#21050=CARTESIAN_POINT('Ctrl Pts',(1.33849388654458,-1.,1.66832460784078));
#21051=CARTESIAN_POINT('Ctrl Pts',(1.33960273470372,-1.,1.67458429426126));
#21052=CARTESIAN_POINT('Ctrl Pts',(1.3406748518516,-1.,1.68086176030308));
#21053=CARTESIAN_POINT('Ctrl Pts',(1.34171037484673,-1.,1.68715660868602));
#21054=CARTESIAN_POINT('Ctrl Pts',(1.34270948206139,-1.,1.6934684849664));
#21055=CARTESIAN_POINT('Ctrl Pts',(1.34367237124322,-1.,1.69979707754221));
#21056=CARTESIAN_POINT('Ctrl Pts',(1.34459924533783,-1.,1.70614212266676));
#21057=CARTESIAN_POINT('Ctrl Pts',(1.34549029589563,-1.,1.71250340687011));
#21058=CARTESIAN_POINT('Ctrl Pts',(1.34634568653586,-1.,1.7188807715095));
#21059=CARTESIAN_POINT('Ctrl Pts',(1.34716554820013,-1.,1.72527410681298));
#21060=CARTESIAN_POINT('Ctrl Pts',(1.3477930915247,-1.,1.73040149654497));
#21061=CARTESIAN_POINT('Ctrl Pts',(1.34824783113158,-1.,1.73425417886255));
#21062=CARTESIAN_POINT('Ctrl Pts',(1.34854391898145,-1.,1.73682580585819));
#21063=CARTESIAN_POINT('Ctrl Pts',(1.34869019493419,-1.,1.73811241238545));
#21064=CARTESIAN_POINT('',(1.23627494547115,-1.,1.81978687191668));
#21065=CARTESIAN_POINT('',(1.34869019493419,-1.,1.73811241238545));
#21066=CARTESIAN_POINT('',(0.892032620296855,-1.,1.5055822144029));
#21067=CARTESIAN_POINT('Ctrl Pts',(1.23627494547115,-1.,1.81978687191668));
#21068=CARTESIAN_POINT('Ctrl Pts',(1.23509651170384,-1.,1.81925017193531));
#21069=CARTESIAN_POINT('Ctrl Pts',(1.23274224526804,-1.,1.81817389920914));
#21070=CARTESIAN_POINT('Ctrl Pts',(1.22921864890975,-1.,1.81655087183054));
#21071=CARTESIAN_POINT('Ctrl Pts',(1.22453613304507,-1.,1.81436959209778));
#21072=CARTESIAN_POINT('Ctrl Pts',(1.2187090610323,-1.,1.81161420806172));
#21073=CARTESIAN_POINT('Ctrl Pts',(1.2129081570818,-1.,1.80882996916931));
#21074=CARTESIAN_POINT('Ctrl Pts',(1.20713356605519,-1.,1.80601678480772));
#21075=CARTESIAN_POINT('Ctrl Pts',(1.2013854893912,-1.,1.8031745483882));
#21076=CARTESIAN_POINT('Ctrl Pts',(1.19566418930405,-1.,1.80030314370121));
#21077=CARTESIAN_POINT('Ctrl Pts',(1.1899699793456,-1.,1.79740245923649));
#21078=CARTESIAN_POINT('Ctrl Pts',(1.18430321697471,-1.,1.79447240321572));
#21079=CARTESIAN_POINT('Ctrl Pts',(1.17866429440781,-1.,1.79151291552646));
#21080=CARTESIAN_POINT('Ctrl Pts',(1.17305363177265,-1.,1.78852398877523));
#21081=CARTESIAN_POINT('Ctrl Pts',(1.16747166312239,-1.,1.78550566040349));
#21082=CARTESIAN_POINT('Ctrl Pts',(1.16191881298458,-1.,1.78245795880949));
#21083=CARTESIAN_POINT('Ctrl Pts',(1.15639547194689,-1.,1.77938085564261));
#21084=CARTESIAN_POINT('Ctrl Pts',(1.15090197841531,-1.,1.77627422557034));
#21085=CARTESIAN_POINT('Ctrl Pts',(1.14543858226948,-1.,1.77313777896234));
#21086=CARTESIAN_POINT('Ctrl Pts',(1.14000548337,-1.,1.76997111386806));
#21087=CARTESIAN_POINT('Ctrl Pts',(1.13460291804634,-1.,1.76677384551883));
#21088=CARTESIAN_POINT('Ctrl Pts',(1.12923123555076,-1.,1.76354571966171));
#21089=CARTESIAN_POINT('Ctrl Pts',(1.12389096855078,-1.,1.76028671825084));
#21090=CARTESIAN_POINT('Ctrl Pts',(1.11858293216752,-1.,1.75699720772089));
#21091=CARTESIAN_POINT('Ctrl Pts',(1.11330807582542,-1.,1.75367772094617));
#21092=CARTESIAN_POINT('Ctrl Pts',(1.10806728183003,-1.,1.75032866075914));
#21093=CARTESIAN_POINT('Ctrl Pts',(1.10286118991144,-1.,1.74695004214924));
#21094=CARTESIAN_POINT('Ctrl Pts',(1.09768999241229,-1.,1.74354119236212));
#21095=CARTESIAN_POINT('Ctrl Pts',(1.09255329056496,-1.,1.74010053962252));
#21096=CARTESIAN_POINT('Ctrl Pts',(1.08745056285429,-1.,1.73662628326093));
#21097=CARTESIAN_POINT('Ctrl Pts',(1.08238162784749,-1.,1.73311705663407));
#21098=CARTESIAN_POINT('Ctrl Pts',(1.0773470373727,-1.,1.72957248977424));
#21099=CARTESIAN_POINT('Ctrl Pts',(1.07234866990252,-1.,1.72599406198489));
#21100=CARTESIAN_POINT('Ctrl Pts',(1.06738966975463,-1.,1.72238500928456));
#21101=CARTESIAN_POINT('Ctrl Pts',(1.06247324680649,-1.,1.71874858456908));
#21102=CARTESIAN_POINT('Ctrl Pts',(1.05760163192481,-1.,1.71508654427022));
#21103=CARTESIAN_POINT('Ctrl Pts',(1.05277517202853,-1.,1.71139783543986));
#21104=CARTESIAN_POINT('Ctrl Pts',(1.0479908540499,-1.,1.70767646263641));
#21105=CARTESIAN_POINT('Ctrl Pts',(1.04324363334546,-1.,1.70391338707969));
#21106=CARTESIAN_POINT('Ctrl Pts',(1.03852922490782,-1.,1.70010052930951));
#21107=CARTESIAN_POINT('Ctrl Pts',(1.03384646003587,-1.,1.69623414782769));
#21108=CARTESIAN_POINT('Ctrl Pts',(1.02919977579155,-1.,1.69231840863471));
#21109=CARTESIAN_POINT('Ctrl Pts',(1.02460180535272,-1.,1.68836910178475));
#21110=CARTESIAN_POINT('Ctrl Pts',(1.02006795074222,-1.,1.68440578021739));
#21111=CARTESIAN_POINT('Ctrl Pts',(1.01561026162786,-1.,1.6804428989482));
#21112=CARTESIAN_POINT('Ctrl Pts',(1.01123236493507,-1.,1.67648246776457));
#21113=CARTESIAN_POINT('Ctrl Pts',(1.00692206696387,-1.,1.67250335383248));
#21114=CARTESIAN_POINT('Ctrl Pts',(1.00265091003682,-1.,1.66846059277231));
#21115=CARTESIAN_POINT('Ctrl Pts',(0.998389654952317,-1.,1.66430758030304));
#21116=CARTESIAN_POINT('Ctrl Pts',(0.994121836661115,-1.,1.66001553809916));
#21117=CARTESIAN_POINT('Ctrl Pts',(0.98985562785445,-1.,1.65559044289746));
#21118=CARTESIAN_POINT('Ctrl Pts',(0.985642622921626,-1.,1.6511001661277));
#21119=CARTESIAN_POINT('Ctrl Pts',(0.981562530940574,-1.,1.64665139190834));
#21120=CARTESIAN_POINT('Ctrl Pts',(0.977689794120296,-1.,1.64233990826831));
#21121=CARTESIAN_POINT('Ctrl Pts',(0.974066058287501,-1.,1.63820952658157));
#21122=CARTESIAN_POINT('Ctrl Pts',(0.970669715996356,-1.,1.63420665729609));
#21123=CARTESIAN_POINT('Ctrl Pts',(0.967387853228041,-1.,1.63013849959083));
#21124=CARTESIAN_POINT('Ctrl Pts',(0.964046107037821,-1.,1.6257193066974));
#21125=CARTESIAN_POINT('Ctrl Pts',(0.960438326099958,-1.,1.62061638139929));
#21126=CARTESIAN_POINT('Ctrl Pts',(0.956354422921572,-1.,1.61449324337233));
#21127=CARTESIAN_POINT('Ctrl Pts',(0.951613284361247,-1.,1.60706069897794));
#21128=CARTESIAN_POINT('Ctrl Pts',(0.946078063325795,-1.,1.59810042045408));
#21129=CARTESIAN_POINT('Ctrl Pts',(0.939646377909319,-1.,1.58744937489796));
#21130=CARTESIAN_POINT('Ctrl Pts',(0.932246680128848,-1.,1.57499388385561));
#21131=CARTESIAN_POINT('Ctrl Pts',(0.923832188966322,-1.,1.56065988582509));
#21132=CARTESIAN_POINT('Ctrl Pts',(0.914375919046579,-1.,1.54440491152808));
#21133=CARTESIAN_POINT('Ctrl Pts',(0.905967409640498,-1.,1.52984849890434));
#21134=CARTESIAN_POINT('Ctrl Pts',(0.89918504749193,-1.,1.51805569591479));
#21135=CARTESIAN_POINT('Ctrl Pts',(0.894452006967538,-1.,1.50980486807181));
#21136=CARTESIAN_POINT('Ctrl Pts',(0.892032620296855,-1.,1.5055822144029));
#21137=CARTESIAN_POINT('',(0.693717979106305,-1.,1.60662857109684));
#21138=CARTESIAN_POINT('Origin',(0.,-1.,0.));
#21139=CARTESIAN_POINT('',(0.7455743247944,-1.,2.0698113262342));
#21140=CARTESIAN_POINT('Ctrl Pts',(0.693717979106305,-1.,1.60662857109684));
#21141=CARTESIAN_POINT('Ctrl Pts',(0.69571209787897,-1.,1.61106790957619));
#21142=CARTESIAN_POINT('Ctrl Pts',(0.699605146398836,-1.,1.61974673471117));
#21143=CARTESIAN_POINT('Ctrl Pts',(0.705159151977294,-1.,1.6321654166204));
#21144=CARTESIAN_POINT('Ctrl Pts',(0.711993139340447,-1.,1.64752408828442));
#21145=CARTESIAN_POINT('Ctrl Pts',(0.719585433787949,-1.,1.66472880551777));
#21146=CARTESIAN_POINT('Ctrl Pts',(0.726235967982445,-1.,1.67996158451922));
#21147=CARTESIAN_POINT('Ctrl Pts',(0.731963238685357,-1.,1.69326921972915));
#21148=CARTESIAN_POINT('Ctrl Pts',(0.736799665716932,-1.,1.70473309004249));
#21149=CARTESIAN_POINT('Ctrl Pts',(0.74079516202821,-1.,1.71447789751001));
#21150=CARTESIAN_POINT('Ctrl Pts',(0.744021445433093,-1.,1.72268229916769));
#21151=CARTESIAN_POINT('Ctrl Pts',(0.746574710097752,-1.,1.72958533647714));
#21152=CARTESIAN_POINT('Ctrl Pts',(0.74858246295687,-1.,1.7355035168033));
#21153=CARTESIAN_POINT('Ctrl Pts',(0.750193435981249,-1.,1.74080458267114));
#21154=CARTESIAN_POINT('Ctrl Pts',(0.751555614164482,-1.,1.74585086852502));
#21155=CARTESIAN_POINT('Ctrl Pts',(0.752797683531314,-1.,1.75095139468794));
#21156=CARTESIAN_POINT('Ctrl Pts',(0.754009254027828,-1.,1.75631083600019));
#21157=CARTESIAN_POINT('Ctrl Pts',(0.755220979974461,-1.,1.76197817240128));
#21158=CARTESIAN_POINT('Ctrl Pts',(0.75642189602781,-1.,1.76789396002998));
#21159=CARTESIAN_POINT('Ctrl Pts',(0.757578264077028,-1.,1.77394167108292));
#21160=CARTESIAN_POINT('Ctrl Pts',(0.758650626677518,-1.,1.77999411220945));
#21161=CARTESIAN_POINT('Ctrl Pts',(0.759614401110189,-1.,1.78596964884604));
#21162=CARTESIAN_POINT('Ctrl Pts',(0.760469555880749,-1.,1.7918581561088));
#21163=CARTESIAN_POINT('Ctrl Pts',(0.761229695230558,-1.,1.79768986997783));
#21164=CARTESIAN_POINT('Ctrl Pts',(0.761915336443547,-1.,1.80351583877342));
#21165=CARTESIAN_POINT('Ctrl Pts',(0.762546129463938,-1.,1.80938551463965));
#21166=CARTESIAN_POINT('Ctrl Pts',(0.763132003836634,-1.,1.8153211840553));
#21167=CARTESIAN_POINT('Ctrl Pts',(0.763673465462726,-1.,1.82131873145266));
#21168=CARTESIAN_POINT('Ctrl Pts',(0.764165902605995,-1.,1.82735991200065));
#21169=CARTESIAN_POINT('Ctrl Pts',(0.764602549687853,-1.,1.83342077227142));
#21170=CARTESIAN_POINT('Ctrl Pts',(0.764978057881737,-1.,1.83948181064835));
#21171=CARTESIAN_POINT('Ctrl Pts',(0.765291664862029,-1.,1.84553698875924));
#21172=CARTESIAN_POINT('Ctrl Pts',(0.765545710619062,-1.,1.85158945130063));
#21173=CARTESIAN_POINT('Ctrl Pts',(0.765744212909318,-1.,1.85764741390394));
#21174=CARTESIAN_POINT('Ctrl Pts',(0.765891519092547,-1.,1.86372027063312));
#21175=CARTESIAN_POINT('Ctrl Pts',(0.765990708546091,-1.,1.86981398314341));
#21176=CARTESIAN_POINT('Ctrl Pts',(0.766042837036744,-1.,1.87592888967883));
#21177=CARTESIAN_POINT('Ctrl Pts',(0.766047794851864,-1.,1.88206215302561));
#21178=CARTESIAN_POINT('Ctrl Pts',(0.766004837062091,-1.,1.88820926433409));
#21179=CARTESIAN_POINT('Ctrl Pts',(0.765913193856978,-1.,1.89436577771388));
#21180=CARTESIAN_POINT('Ctrl Pts',(0.765772772593386,-1.,1.90052930393596));
#21181=CARTESIAN_POINT('Ctrl Pts',(0.765584196937919,-1.,1.90669961402356));
#21182=CARTESIAN_POINT('Ctrl Pts',(0.765348465884722,-1.,1.91287765805169));
#21183=CARTESIAN_POINT('Ctrl Pts',(0.765066729667088,-1.,1.91906491634196));
#21184=CARTESIAN_POINT('Ctrl Pts',(0.764740025488211,-1.,1.92526263537048));
#21185=CARTESIAN_POINT('Ctrl Pts',(0.76436901067394,-1.,1.93147105496382));
#21186=CARTESIAN_POINT('Ctrl Pts',(0.763954049121458,-1.,1.93768964875886));
#21187=CARTESIAN_POINT('Ctrl Pts',(0.763495333538629,-1.,1.9439174661764));
#21188=CARTESIAN_POINT('Ctrl Pts',(0.762992990878769,-1.,1.95015342590024));
#21189=CARTESIAN_POINT('Ctrl Pts',(0.762447203806178,-1.,1.95639665309869));
#21190=CARTESIAN_POINT('Ctrl Pts',(0.761858300014423,-1.,1.96264672744186));
#21191=CARTESIAN_POINT('Ctrl Pts',(0.76122669048382,-1.,1.96890351582499));
#21192=CARTESIAN_POINT('Ctrl Pts',(0.760552825409757,-1.,1.97516705321494));
#21193=CARTESIAN_POINT('Ctrl Pts',(0.75983714745219,-1.,1.98143741418172));
#21194=CARTESIAN_POINT('Ctrl Pts',(0.759080037802488,-1.,1.98771456680874));
#21195=CARTESIAN_POINT('Ctrl Pts',(0.758281796766761,-1.,1.99399831098817));
#21196=CARTESIAN_POINT('Ctrl Pts',(0.757442676862724,-1.,2.00028834739178));
#21197=CARTESIAN_POINT('Ctrl Pts',(0.75656290464667,-1.,2.0065843158773));
#21198=CARTESIAN_POINT('Ctrl Pts',(0.755642704957865,-1.,2.01288584328084));
#21199=CARTESIAN_POINT('Ctrl Pts',(0.754682330722816,-1.,2.01919259405809));
#21200=CARTESIAN_POINT('Ctrl Pts',(0.753682061112768,-1.,2.02550428623313));
#21201=CARTESIAN_POINT('Ctrl Pts',(0.75264218048721,-1.,2.03182068456221));
#21202=CARTESIAN_POINT('Ctrl Pts',(0.751562963361115,-1.,2.03814160092099));
#21203=CARTESIAN_POINT('Ctrl Pts',(0.750444657875575,-1.,2.04446689147979));
#21204=CARTESIAN_POINT('Ctrl Pts',(0.749287468665046,-1.,2.05079645592154));
#21205=CARTESIAN_POINT('Ctrl Pts',(0.748091554183802,-1.,2.05713023031007));
#21206=CARTESIAN_POINT('Ctrl Pts',(0.747103932787919,-1.,2.06220058927826));
#21207=CARTESIAN_POINT('Ctrl Pts',(0.7463458715442,-1.,2.06600523016815));
#21208=CARTESIAN_POINT('Ctrl Pts',(0.745832791378367,-1.,2.06854248895728));
#21209=CARTESIAN_POINT('Ctrl Pts',(0.7455743247944,-1.,2.0698113262342));
#21210=CARTESIAN_POINT('',(0.61342227326009,-1.,2.11275013067528));
#21211=CARTESIAN_POINT('',(0.7455743247944,-1.,2.0698113262342));
#21212=CARTESIAN_POINT('',(0.383122945602004,-1.,1.7075470150345));
#21213=CARTESIAN_POINT('Ctrl Pts',(0.61342227326009,-1.,2.11275013067528));
#21214=CARTESIAN_POINT('Ctrl Pts',(0.6124673655618,-1.,2.11187554259986));
#21215=CARTESIAN_POINT('Ctrl Pts',(0.610560911689898,-1.,2.11012443807238));
#21216=CARTESIAN_POINT('Ctrl Pts',(0.607711315454876,-1.,2.1074919961518));
#21217=CARTESIAN_POINT('Ctrl Pts',(0.60393203073603,-1.,2.10397049886949));
#21218=CARTESIAN_POINT('Ctrl Pts',(0.599241616420533,-1.,2.0995493086477));
#21219=CARTESIAN_POINT('Ctrl Pts',(0.594585006052162,-1.,2.0951087622027));
#21220=CARTESIAN_POINT('Ctrl Pts',(0.589962365403406,-1.,2.09064881812129));
#21221=CARTESIAN_POINT('Ctrl Pts',(0.585373918991617,-1.,2.08616943727951));
#21222=CARTESIAN_POINT('Ctrl Pts',(0.580819952108063,-1.,2.08167059018418));
#21223=CARTESIAN_POINT('Ctrl Pts',(0.576300797416844,-1.,2.07715226767559));
#21224=CARTESIAN_POINT('Ctrl Pts',(0.571816823242602,-1.,2.07261449292824));
#21225=CARTESIAN_POINT('Ctrl Pts',(0.567368421181087,-1.,2.06805732997334));
#21226=CARTESIAN_POINT('Ctrl Pts',(0.562955993082261,-1.,2.06348090160589));
#21227=CARTESIAN_POINT('Ctrl Pts',(0.558579940185151,-1.,2.05888537756462));
#21228=CARTESIAN_POINT('Ctrl Pts',(0.554240657463906,-1.,2.05427091604413));
#21229=CARTESIAN_POINT('Ctrl Pts',(0.549938525150295,-1.,2.04963761077958));
#21230=CARTESIAN_POINT('Ctrl Pts',(0.54567390381743,-1.,2.04498544714588));
#21231=CARTESIAN_POINT('Ctrl Pts',(0.541447120615659,-1.,2.04031422690527));
#21232=CARTESIAN_POINT('Ctrl Pts',(0.537258489833262,-1.,2.03562362954037));
#21233=CARTESIAN_POINT('Ctrl Pts',(0.533108355132976,-1.,2.03091336214426));
#21234=CARTESIAN_POINT('Ctrl Pts',(0.528997127241914,-1.,2.0261832908329));
#21235=CARTESIAN_POINT('Ctrl Pts',(0.524925318333476,-1.,2.02143356304698));
#21236=CARTESIAN_POINT('Ctrl Pts',(0.52089359039937,-1.,2.01666477917286));
#21237=CARTESIAN_POINT('Ctrl Pts',(0.516902681728687,-1.,2.01187773939242));
#21238=CARTESIAN_POINT('Ctrl Pts',(0.512953306961792,-1.,2.00707309946949));
#21239=CARTESIAN_POINT('Ctrl Pts',(0.509046069886157,-1.,2.00225107134734));
#21240=CARTESIAN_POINT('Ctrl Pts',(0.505181361323026,-1.,1.99741107463572));
#21241=CARTESIAN_POINT('Ctrl Pts',(0.501359287727146,-1.,1.99255149126155));
#21242=CARTESIAN_POINT('Ctrl Pts',(0.497579909545574,-1.,1.98767044752932));
#21243=CARTESIAN_POINT('Ctrl Pts',(0.493843476541494,-1.,1.98276658761821));
#21244=CARTESIAN_POINT('Ctrl Pts',(0.490150627860952,-1.,1.97783973019229));
#21245=CARTESIAN_POINT('Ctrl Pts',(0.486502692907658,-1.,1.97289186263272));
#21246=CARTESIAN_POINT('Ctrl Pts',(0.48290166212069,-1.,1.96792703422362));
#21247=CARTESIAN_POINT('Ctrl Pts',(0.479349583074855,-1.,1.96294933055943));
#21248=CARTESIAN_POINT('Ctrl Pts',(0.475848034683176,-1.,1.95796111148177));
#21249=CARTESIAN_POINT('Ctrl Pts',(0.472397672264072,-1.,1.95296148278133));
#21250=CARTESIAN_POINT('Ctrl Pts',(0.468997482913135,-1.,1.94794381136514));
#21251=CARTESIAN_POINT('Ctrl Pts',(0.46564546202603,-1.,1.9428979419619));
#21252=CARTESIAN_POINT('Ctrl Pts',(0.462340031009056,-1.,1.93781486640821));
#21253=CARTESIAN_POINT('Ctrl Pts',(0.459081234547926,-1.,1.93269066517934));
#21254=CARTESIAN_POINT('Ctrl Pts',(0.45587200517437,-1.,1.92753067150476));
#21255=CARTESIAN_POINT('Ctrl Pts',(0.452719478359432,-1.,1.92235380648502));
#21256=CARTESIAN_POINT('Ctrl Pts',(0.449632260106662,-1.,1.91718342555755));
#21257=CARTESIAN_POINT('Ctrl Pts',(0.446617343485711,-1.,1.9120369998112));
#21258=CARTESIAN_POINT('Ctrl Pts',(0.44367755684915,-1.,1.90691756144898));
#21259=CARTESIAN_POINT('Ctrl Pts',(0.440807833704038,-1.,1.90180124389086));
#21260=CARTESIAN_POINT('Ctrl Pts',(0.437995003948244,-1.,1.89663648956466));
#21261=CARTESIAN_POINT('Ctrl Pts',(0.435225660963383,-1.,1.89136993975504));
#21262=CARTESIAN_POINT('Ctrl Pts',(0.432493038548748,-1.,1.88596913666793));
#21263=CARTESIAN_POINT('Ctrl Pts',(0.429803062482344,-1.,1.88044229001832));
#21264=CARTESIAN_POINT('Ctrl Pts',(0.427183828519102,-1.,1.87486989291484));
#21265=CARTESIAN_POINT('Ctrl Pts',(0.424678177291358,-1.,1.86937803944323));
#21266=CARTESIAN_POINT('Ctrl Pts',(0.422327307418275,-1.,1.86408083334028));
#21267=CARTESIAN_POINT('Ctrl Pts',(0.420157287975619,-1.,1.85903281096686));
#21268=CARTESIAN_POINT('Ctrl Pts',(0.418164129143534,-1.,1.85417632856234));
#21269=CARTESIAN_POINT('Ctrl Pts',(0.416300022038864,-1.,1.84929312929882));
#21270=CARTESIAN_POINT('Ctrl Pts',(0.41448743825434,-1.,1.8440575707371));
#21271=CARTESIAN_POINT('Ctrl Pts',(0.412633125322161,-1.,1.83808953475839));
#21272=CARTESIAN_POINT('Ctrl Pts',(0.410641256301674,-1.,1.83100408895216));
#21273=CARTESIAN_POINT('Ctrl Pts',(0.408428948108533,-1.,1.8224702267854));
#21274=CARTESIAN_POINT('Ctrl Pts',(0.405933518411838,-1.,1.81223801813988));
#21275=CARTESIAN_POINT('Ctrl Pts',(0.403107976170441,-1.,1.80012077176221));
#21276=CARTESIAN_POINT('Ctrl Pts',(0.39991940378308,-1.,1.78598826347533));
#21277=CARTESIAN_POINT('Ctrl Pts',(0.39634619612042,-1.,1.7697556004756));
#21278=CARTESIAN_POINT('Ctrl Pts',(0.392375812294307,-1.,1.75137405313962));
#21279=CARTESIAN_POINT('Ctrl Pts',(0.388877023509191,-1.,1.7349317097561));
#21280=CARTESIAN_POINT('Ctrl Pts',(0.38607079032701,-1.,1.72162022246158));
#21281=CARTESIAN_POINT('Ctrl Pts',(0.384119047315541,-1.,1.71231062891958));
#21282=CARTESIAN_POINT('Ctrl Pts',(0.383122945602004,-1.,1.7075470150345));
#21283=CARTESIAN_POINT('',(0.163289472382896,-1.,1.74236521665491));
#21284=CARTESIAN_POINT('Origin',(0.,-1.,0.));
#21285=CARTESIAN_POINT('',(0.0694764450219578,-1.,2.19890268624765));
#21286=CARTESIAN_POINT('Ctrl Pts',(0.163289472382896,-1.,1.74236521665491));
#21287=CARTESIAN_POINT('Ctrl Pts',(0.163814161002002,-1.,1.7472034950333));
#21288=CARTESIAN_POINT('Ctrl Pts',(0.164834765707158,-1.,1.75666056638427));
#21289=CARTESIAN_POINT('Ctrl Pts',(0.1662793551464,-1.,1.77018771684844));
#21290=CARTESIAN_POINT('Ctrl Pts',(0.168032772805197,-1.,1.7869064998507));
#21291=CARTESIAN_POINT('Ctrl Pts',(0.169936923904608,-1.,1.80561530629706));
#21292=CARTESIAN_POINT('Ctrl Pts',(0.171554770204119,-1.,1.82215766811545));
#21293=CARTESIAN_POINT('Ctrl Pts',(0.1728894428919,-1.,1.83658380527692));
#21294=CARTESIAN_POINT('Ctrl Pts',(0.173946627587731,-1.,1.8489811319852));
#21295=CARTESIAN_POINT('Ctrl Pts',(0.17473525927603,-1.,1.85948367088837));
#21296=CARTESIAN_POINT('Ctrl Pts',(0.175268337590757,-1.,1.86828349694799));
#21297=CARTESIAN_POINT('Ctrl Pts',(0.175563480746485,-1.,1.87563767773588));
#21298=CARTESIAN_POINT('Ctrl Pts',(0.175644148889698,-1.,1.88188663145367));
#21299=CARTESIAN_POINT('Ctrl Pts',(0.175538155840648,-1.,1.88742606273259));
#21300=CARTESIAN_POINT('Ctrl Pts',(0.175274276190844,-1.,1.892646301985));
#21301=CARTESIAN_POINT('Ctrl Pts',(0.174879405091263,-1.,1.89788101117132));
#21302=CARTESIAN_POINT('Ctrl Pts',(0.174375518661085,-1.,1.90335253862834));
#21303=CARTESIAN_POINT('Ctrl Pts',(0.173776635257816,-1.,1.90911693975267));
#21304=CARTESIAN_POINT('Ctrl Pts',(0.173090695383496,-1.,1.91511429159527));
#21305=CARTESIAN_POINT('Ctrl Pts',(0.172321621259513,-1.,1.9212233439798));
#21306=CARTESIAN_POINT('Ctrl Pts',(0.171471191532988,-1.,1.92731093582036));
#21307=CARTESIAN_POINT('Ctrl Pts',(0.170541253116201,-1.,1.93329183155539));
#21308=CARTESIAN_POINT('Ctrl Pts',(0.16953490481749,-1.,1.93915639211581));
#21309=CARTESIAN_POINT('Ctrl Pts',(0.168455741607556,-1.,1.94493757756931));
#21310=CARTESIAN_POINT('Ctrl Pts',(0.167307501784475,-1.,1.95069027794294));
#21311=CARTESIAN_POINT('Ctrl Pts',(0.166093592002812,-1.,1.9564675971873));
#21312=CARTESIAN_POINT('Ctrl Pts',(0.164816568920269,-1.,1.96229379940136));
#21313=CARTESIAN_POINT('Ctrl Pts',(0.163478185457734,-1.,1.96816512677967));
#21314=CARTESIAN_POINT('Ctrl Pts',(0.162079693556288,-1.,1.97406280235188));
#21315=CARTESIAN_POINT('Ctrl Pts',(0.160622060784611,-1.,1.97996195437559));
#21316=CARTESIAN_POINT('Ctrl Pts',(0.159106226437299,-1.,1.98584238283292));
#21317=CARTESIAN_POINT('Ctrl Pts',(0.157533331459227,-1.,1.99169810931908));
#21318=CARTESIAN_POINT('Ctrl Pts',(0.155904629548783,-1.,1.99753284771497));
#21319=CARTESIAN_POINT('Ctrl Pts',(0.154221403049722,-1.,2.00335565310543));
#21320=CARTESIAN_POINT('Ctrl Pts',(0.152484883621449,-1.,2.00917680318424));
#21321=CARTESIAN_POINT('Ctrl Pts',(0.150696157673078,-1.,2.01500291940238));
#21322=CARTESIAN_POINT('Ctrl Pts',(0.148856124775337,-1.,2.02083464969894));
#21323=CARTESIAN_POINT('Ctrl Pts',(0.146965557332583,-1.,2.02666926182017));
#21324=CARTESIAN_POINT('Ctrl Pts',(0.145025140186057,-1.,2.03250223739942));
#21325=CARTESIAN_POINT('Ctrl Pts',(0.143035515058208,-1.,2.03832911025912));
#21326=CARTESIAN_POINT('Ctrl Pts',(0.140997332152546,-1.,2.04414757947916));
#21327=CARTESIAN_POINT('Ctrl Pts',(0.138911255368966,-1.,2.04995762001328));
#21328=CARTESIAN_POINT('Ctrl Pts',(0.136777941218043,-1.,2.05576044414264));
#21329=CARTESIAN_POINT('Ctrl Pts',(0.134598026192106,-1.,2.06155781517842));
#21330=CARTESIAN_POINT('Ctrl Pts',(0.13237211154771,-1.,2.06735123910326));
#21331=CARTESIAN_POINT('Ctrl Pts',(0.130100748328403,-1.,2.07314114713063));
#21332=CARTESIAN_POINT('Ctrl Pts',(0.12778444527612,-1.,2.07892715110987));
#21333=CARTESIAN_POINT('Ctrl Pts',(0.125423679412061,-1.,2.08470840653643));
#21334=CARTESIAN_POINT('Ctrl Pts',(0.123018905621083,-1.,2.09048392424825));
#21335=CARTESIAN_POINT('Ctrl Pts',(0.120570567965122,-1.,2.0962529286773));
#21336=CARTESIAN_POINT('Ctrl Pts',(0.118079107988355,-1.,2.102015121329));
#21337=CARTESIAN_POINT('Ctrl Pts',(0.115544957687926,-1.,2.10777050261309));
#21338=CARTESIAN_POINT('Ctrl Pts',(0.112968534419737,-1.,2.11351924490306));
#21339=CARTESIAN_POINT('Ctrl Pts',(0.110350236135025,-1.,2.11926155590865));
#21340=CARTESIAN_POINT('Ctrl Pts',(0.10769043523109,-1.,2.12499752307));
#21341=CARTESIAN_POINT('Ctrl Pts',(0.104989479152739,-1.,2.13072704887293));
#21342=CARTESIAN_POINT('Ctrl Pts',(0.1022477005561,-1.,2.13644992667165));
#21343=CARTESIAN_POINT('Ctrl Pts',(0.0994654261990913,-1.,2.14216588396025));
#21344=CARTESIAN_POINT('Ctrl Pts',(0.0966429852305456,-1.,2.14787463531795));
#21345=CARTESIAN_POINT('Ctrl Pts',(0.0937807218867641,-1.,2.1535759397817));
#21346=CARTESIAN_POINT('Ctrl Pts',(0.0908789888107263,-1.,2.15926961544516));
#21347=CARTESIAN_POINT('Ctrl Pts',(0.087938129138692,-1.,2.16495552645014));
#21348=CARTESIAN_POINT('Ctrl Pts',(0.084958462083537,-1.,2.17063357870952));
#21349=CARTESIAN_POINT('Ctrl Pts',(0.0819402680872763,-1.,2.176303712113));
#21350=CARTESIAN_POINT('Ctrl Pts',(0.078883772768524,-1.,2.18196589448887));
#21351=CARTESIAN_POINT('Ctrl Pts',(0.0757891465836145,-1.,2.1876201139953));
#21352=CARTESIAN_POINT('Ctrl Pts',(0.0732830357306722,-1.,2.19213712013662));
#21353=CARTESIAN_POINT('Ctrl Pts',(0.0713863779526151,-1.,2.19552129484002));
#21354=CARTESIAN_POINT('Ctrl Pts',(0.0701143536325487,-1.,2.19777582085423));
#21355=CARTESIAN_POINT('Ctrl Pts',(0.0694764450219578,-1.,2.19890268624765));
#21356=CARTESIAN_POINT('',(-0.0694764450219586,-1.,2.19890268624765));
#21357=CARTESIAN_POINT('',(0.0694764450219578,-1.,2.19890268624765));
#21358=CARTESIAN_POINT('',(-0.163289472382896,-1.,1.74236521665491));
#21359=CARTESIAN_POINT('Ctrl Pts',(-0.0694764450219586,-1.,2.19890268624765));
#21360=CARTESIAN_POINT('Ctrl Pts',(-0.0701143536324929,-1.,2.19777582085261));
#21361=CARTESIAN_POINT('Ctrl Pts',(-0.071386377952463,-1.,2.19552129483562));
#21362=CARTESIAN_POINT('Ctrl Pts',(-0.0732830357304279,-1.,2.19213712012956));
#21363=CARTESIAN_POINT('Ctrl Pts',(-0.0757891465833414,-1.,2.1876201139874));
#21364=CARTESIAN_POINT('Ctrl Pts',(-0.078883772768323,-1.,2.18196589448304));
#21365=CARTESIAN_POINT('Ctrl Pts',(-0.0819402680871942,-1.,2.1763037121106));
#21366=CARTESIAN_POINT('Ctrl Pts',(-0.0849584620835646,-1.,2.17063357871031));
#21367=CARTESIAN_POINT('Ctrl Pts',(-0.0879381291387825,-1.,2.16495552645275));
#21368=CARTESIAN_POINT('Ctrl Pts',(-0.0908789888108269,-1.,2.15926961544808));
#21369=CARTESIAN_POINT('Ctrl Pts',(-0.0937807218868348,-1.,2.15357593978377));
#21370=CARTESIAN_POINT('Ctrl Pts',(-0.0966429852305691,-1.,2.14787463531864));
#21371=CARTESIAN_POINT('Ctrl Pts',(-0.0994654261990745,-1.,2.14216588395974));
#21372=CARTESIAN_POINT('Ctrl Pts',(-0.102247700556064,-1.,2.13644992667052));
#21373=CARTESIAN_POINT('Ctrl Pts',(-0.104989479152703,-1.,2.1307270488718));
#21374=CARTESIAN_POINT('Ctrl Pts',(-0.107690435231068,-1.,2.12499752306927));
#21375=CARTESIAN_POINT('Ctrl Pts',(-0.11035023613502,-1.,2.11926155590849));
#21376=CARTESIAN_POINT('Ctrl Pts',(-0.112968534419746,-1.,2.11351924490335));
#21377=CARTESIAN_POINT('Ctrl Pts',(-0.115544957687941,-1.,2.10777050261359));
#21378=CARTESIAN_POINT('Ctrl Pts',(-0.118079107988368,-1.,2.10201512132945));
#21379=CARTESIAN_POINT('Ctrl Pts',(-0.120570567965129,-1.,2.09625292867756));
#21380=CARTESIAN_POINT('Ctrl Pts',(-0.123018905621083,-1.,2.09048392424826));
#21381=CARTESIAN_POINT('Ctrl Pts',(-0.125423679412058,-1.,2.08470840653628));
#21382=CARTESIAN_POINT('Ctrl Pts',(-0.127784445276116,-1.,2.07892715110967));
#21383=CARTESIAN_POINT('Ctrl Pts',(-0.130100748328401,-1.,2.07314114713047));
#21384=CARTESIAN_POINT('Ctrl Pts',(-0.13237211154771,-1.,2.06735123910319));
#21385=CARTESIAN_POINT('Ctrl Pts',(-0.134598026192107,-1.,2.06155781517844));
#21386=CARTESIAN_POINT('Ctrl Pts',(-0.136777941218044,-1.,2.0557604441427));
#21387=CARTESIAN_POINT('Ctrl Pts',(-0.138911255368966,-1.,2.04995762001333));
#21388=CARTESIAN_POINT('Ctrl Pts',(-0.140997332152546,-1.,2.04414757947919));
#21389=CARTESIAN_POINT('Ctrl Pts',(-0.143035515058208,-1.,2.03832911025913));
#21390=CARTESIAN_POINT('Ctrl Pts',(-0.145025140186058,-1.,2.03250223739941));
#21391=CARTESIAN_POINT('Ctrl Pts',(-0.146965557332586,-1.,2.02666926182017));
#21392=CARTESIAN_POINT('Ctrl Pts',(-0.148856124775343,-1.,2.02083464969897));
#21393=CARTESIAN_POINT('Ctrl Pts',(-0.150696157673084,-1.,2.01500291940243));
#21394=CARTESIAN_POINT('Ctrl Pts',(-0.152484883621452,-1.,2.00917680318426));
#21395=CARTESIAN_POINT('Ctrl Pts',(-0.154221403049719,-1.,2.00335565310539));
#21396=CARTESIAN_POINT('Ctrl Pts',(-0.155904629548775,-1.,1.99753284771487));
#21397=CARTESIAN_POINT('Ctrl Pts',(-0.157533331459215,-1.,1.99169810931893));
#21398=CARTESIAN_POINT('Ctrl Pts',(-0.159106226437289,-1.,1.98584238283279));
#21399=CARTESIAN_POINT('Ctrl Pts',(-0.16062206078461,-1.,1.97996195437557));
#21400=CARTESIAN_POINT('Ctrl Pts',(-0.162079693556302,-1.,1.97406280235204));
#21401=CARTESIAN_POINT('Ctrl Pts',(-0.16347818545776,-1.,1.96816512678));
#21402=CARTESIAN_POINT('Ctrl Pts',(-0.1648165689203,-1.,1.96229379940174));
#21403=CARTESIAN_POINT('Ctrl Pts',(-0.166093592002833,-1.,1.95646759718755));
#21404=CARTESIAN_POINT('Ctrl Pts',(-0.167307501784469,-1.,1.95069027794286));
#21405=CARTESIAN_POINT('Ctrl Pts',(-0.168455741607516,-1.,1.94493757756879));
#21406=CARTESIAN_POINT('Ctrl Pts',(-0.169534904817425,-1.,1.93915639211497));
#21407=CARTESIAN_POINT('Ctrl Pts',(-0.170541253116136,-1.,1.93329183155455));
#21408=CARTESIAN_POINT('Ctrl Pts',(-0.17147119153296,-1.,1.92731093582));
#21409=CARTESIAN_POINT('Ctrl Pts',(-0.172321621259557,-1.,1.92122334398034));
#21410=CARTESIAN_POINT('Ctrl Pts',(-0.173090695383619,-1.,1.91511429159681));
#21411=CARTESIAN_POINT('Ctrl Pts',(-0.173776635257984,-1.,1.90911693975475));
#21412=CARTESIAN_POINT('Ctrl Pts',(-0.174375518661222,-1.,1.90335253863003));
#21413=CARTESIAN_POINT('Ctrl Pts',(-0.174879405091277,-1.,1.89788101117148));
#21414=CARTESIAN_POINT('Ctrl Pts',(-0.175274276190664,-1.,1.89264630198279));
#21415=CARTESIAN_POINT('Ctrl Pts',(-0.175538155840286,-1.,1.88742606272818));
#21416=CARTESIAN_POINT('Ctrl Pts',(-0.175644148889271,-1.,1.88188663144846));
#21417=CARTESIAN_POINT('Ctrl Pts',(-0.175563480746206,-1.,1.87563767773249));
#21418=CARTESIAN_POINT('Ctrl Pts',(-0.175268337590901,-1.,1.86828349694972));
#21419=CARTESIAN_POINT('Ctrl Pts',(-0.174735259276856,-1.,1.85948367089838));
#21420=CARTESIAN_POINT('Ctrl Pts',(-0.173946627589401,-1.,1.84898113200543));
#21421=CARTESIAN_POINT('Ctrl Pts',(-0.17288944289442,-1.,1.83658380530747));
#21422=CARTESIAN_POINT('Ctrl Pts',(-0.171554770207306,-1.,1.82215766815414));
#21423=CARTESIAN_POINT('Ctrl Pts',(-0.169936923908078,-1.,1.80561530633924));
#21424=CARTESIAN_POINT('Ctrl Pts',(-0.16803277280837,-1.,1.78690649988931));
#21425=CARTESIAN_POINT('Ctrl Pts',(-0.166279355148738,-1.,1.77018771687692));
#21426=CARTESIAN_POINT('Ctrl Pts',(-0.164834765708484,-1.,1.75666056640041));
#21427=CARTESIAN_POINT('Ctrl Pts',(-0.163814161002474,-1.,1.74720349503904));
#21428=CARTESIAN_POINT('Ctrl Pts',(-0.163289472382896,-1.,1.74236521665491));
#21429=CARTESIAN_POINT('',(-0.383122945602004,-1.,1.7075470150345));
#21430=CARTESIAN_POINT('Origin',(0.,-1.,0.));
#21431=CARTESIAN_POINT('',(-0.61342227326009,-1.,2.11275013067528));
#21432=CARTESIAN_POINT('Ctrl Pts',(-0.383122945602004,-1.,1.7075470150345));
#21433=CARTESIAN_POINT('Ctrl Pts',(-0.384119047314215,-1.,1.71231062891398));
#21434=CARTESIAN_POINT('Ctrl Pts',(-0.386070790323281,-1.,1.72162022244582));
#21435=CARTESIAN_POINT('Ctrl Pts',(-0.388877023502615,-1.,1.73493170972829));
#21436=CARTESIAN_POINT('Ctrl Pts',(-0.392375812285395,-1.,1.75137405310193));
#21437=CARTESIAN_POINT('Ctrl Pts',(-0.396346196110688,-1.,1.76975560043442));
#21438=CARTESIAN_POINT('Ctrl Pts',(-0.399919403774155,-1.,1.78598826343754));
#21439=CARTESIAN_POINT('Ctrl Pts',(-0.403107976163396,-1.,1.80012077173238));
#21440=CARTESIAN_POINT('Ctrl Pts',(-0.405933518407175,-1.,1.81223801812013));
#21441=CARTESIAN_POINT('Ctrl Pts',(-0.408428948106227,-1.,1.82247022677562));
#21442=CARTESIAN_POINT('Ctrl Pts',(-0.410641256301276,-1.,1.83100408895047));
#21443=CARTESIAN_POINT('Ctrl Pts',(-0.412633125322945,-1.,1.8380895347617));
#21444=CARTESIAN_POINT('Ctrl Pts',(-0.414487438255542,-1.,1.84405757074218));
#21445=CARTESIAN_POINT('Ctrl Pts',(-0.416300022039885,-1.,1.84929312930314));
#21446=CARTESIAN_POINT('Ctrl Pts',(-0.418164129144045,-1.,1.8541763285645));
#21447=CARTESIAN_POINT('Ctrl Pts',(-0.420157287975583,-1.,1.8590328109667));
#21448=CARTESIAN_POINT('Ctrl Pts',(-0.422327307417885,-1.,1.86408083333863));
#21449=CARTESIAN_POINT('Ctrl Pts',(-0.424678177290876,-1.,1.8693780394412));
#21450=CARTESIAN_POINT('Ctrl Pts',(-0.427183828518743,-1.,1.87486989291333));
#21451=CARTESIAN_POINT('Ctrl Pts',(-0.429803062482217,-1.,1.88044229001778));
#21452=CARTESIAN_POINT('Ctrl Pts',(-0.432493038548833,-1.,1.88596913666828));
#21453=CARTESIAN_POINT('Ctrl Pts',(-0.43522566096358,-1.,1.89136993975585));
#21454=CARTESIAN_POINT('Ctrl Pts',(-0.437995003948443,-1.,1.89663648956549));
#21455=CARTESIAN_POINT('Ctrl Pts',(-0.440807833704161,-1.,1.90180124389137));
#21456=CARTESIAN_POINT('Ctrl Pts',(-0.44367755684917,-1.,1.90691756144906));
#21457=CARTESIAN_POINT('Ctrl Pts',(-0.446617343485651,-1.,1.91203699981095));
#21458=CARTESIAN_POINT('Ctrl Pts',(-0.449632260106572,-1.,1.91718342555717));
#21459=CARTESIAN_POINT('Ctrl Pts',(-0.452719478359356,-1.,1.9223538064847));
#21460=CARTESIAN_POINT('Ctrl Pts',(-0.455872005174335,-1.,1.92753067150461));
#21461=CARTESIAN_POINT('Ctrl Pts',(-0.459081234547931,-1.,1.93269066517936));
#21462=CARTESIAN_POINT('Ctrl Pts',(-0.462340031009087,-1.,1.93781486640834));
#21463=CARTESIAN_POINT('Ctrl Pts',(-0.465645462026065,-1.,1.94289794196205));
#21464=CARTESIAN_POINT('Ctrl Pts',(-0.468997482913158,-1.,1.94794381136524));
#21465=CARTESIAN_POINT('Ctrl Pts',(-0.47239767226408,-1.,1.95296148278136));
#21466=CARTESIAN_POINT('Ctrl Pts',(-0.475848034683172,-1.,1.95796111148175));
#21467=CARTESIAN_POINT('Ctrl Pts',(-0.479349583074846,-1.,1.96294933055938));
#21468=CARTESIAN_POINT('Ctrl Pts',(-0.482901662120687,-1.,1.96792703422358));
#21469=CARTESIAN_POINT('Ctrl Pts',(-0.486502692907661,-1.,1.97289186263272));
#21470=CARTESIAN_POINT('Ctrl Pts',(-0.490150627860955,-1.,1.97783973019229));
#21471=CARTESIAN_POINT('Ctrl Pts',(-0.493843476541492,-1.,1.9827665876182));
#21472=CARTESIAN_POINT('Ctrl Pts',(-0.497579909545564,-1.,1.98767044752929));
#21473=CARTESIAN_POINT('Ctrl Pts',(-0.501359287727129,-1.,1.9925514912615));
#21474=CARTESIAN_POINT('Ctrl Pts',(-0.505181361323011,-1.,1.99741107463567));
#21475=CARTESIAN_POINT('Ctrl Pts',(-0.509046069886152,-1.,2.00225107134733));
#21476=CARTESIAN_POINT('Ctrl Pts',(-0.512953306961814,-1.,2.00707309946955));
#21477=CARTESIAN_POINT('Ctrl Pts',(-0.516902681728733,-1.,2.01187773939257));
#21478=CARTESIAN_POINT('Ctrl Pts',(-0.520893590399428,-1.,2.01666477917305));
#21479=CARTESIAN_POINT('Ctrl Pts',(-0.524925318333518,-1.,2.02143356304712));
#21480=CARTESIAN_POINT('Ctrl Pts',(-0.528997127241911,-1.,2.02618329083289));
#21481=CARTESIAN_POINT('Ctrl Pts',(-0.533108355132905,-1.,2.03091336214401));
#21482=CARTESIAN_POINT('Ctrl Pts',(-0.537258489833134,-1.,2.03562362953993));
#21483=CARTESIAN_POINT('Ctrl Pts',(-0.54144712061552,-1.,2.0403142269048));
#21484=CARTESIAN_POINT('Ctrl Pts',(-0.545673903817348,-1.,2.0449854471456));
#21485=CARTESIAN_POINT('Ctrl Pts',(-0.549938525150342,-1.,2.04963761077974));
#21486=CARTESIAN_POINT('Ctrl Pts',(-0.55424065746411,-1.,2.05427091604482));
#21487=CARTESIAN_POINT('Ctrl Pts',(-0.558579940185467,-1.,2.05888537756571));
#21488=CARTESIAN_POINT('Ctrl Pts',(-0.562955993082574,-1.,2.06348090160697));
#21489=CARTESIAN_POINT('Ctrl Pts',(-0.567368421181229,-1.,2.06805732997383));
#21490=CARTESIAN_POINT('Ctrl Pts',(-0.571816823242411,-1.,2.07261449292757));
#21491=CARTESIAN_POINT('Ctrl Pts',(-0.576300797416275,-1.,2.07715226767361));
#21492=CARTESIAN_POINT('Ctrl Pts',(-0.580819952107257,-1.,2.08167059018138));
#21493=CARTESIAN_POINT('Ctrl Pts',(-0.585373918990895,-1.,2.086169437277));
#21494=CARTESIAN_POINT('Ctrl Pts',(-0.589962365403189,-1.,2.09064881812053));
#21495=CARTESIAN_POINT('Ctrl Pts',(-0.594585006052824,-1.,2.09510876220501));
#21496=CARTESIAN_POINT('Ctrl Pts',(-0.599241616422144,-1.,2.09954930865331));
#21497=CARTESIAN_POINT('Ctrl Pts',(-0.603932030738212,-1.,2.10397049887709));
#21498=CARTESIAN_POINT('Ctrl Pts',(-0.607711315456826,-1.,2.10749199615859));
#21499=CARTESIAN_POINT('Ctrl Pts',(-0.610560911691113,-1.,2.11012443807661));
#21500=CARTESIAN_POINT('Ctrl Pts',(-0.61246736556225,-1.,2.11187554260142));
#21501=CARTESIAN_POINT('Ctrl Pts',(-0.61342227326009,-1.,2.11275013067528));
#21502=CARTESIAN_POINT('',(-0.745574324794401,-1.,2.0698113262342));
#21503=CARTESIAN_POINT('',(-0.61342227326009,-1.,2.11275013067528));
#21504=CARTESIAN_POINT('',(-0.693717979106306,-1.,1.60662857109684));
#21505=CARTESIAN_POINT('Ctrl Pts',(-0.745574324794401,-1.,2.0698113262342));
#21506=CARTESIAN_POINT('Ctrl Pts',(-0.74583279137781,-1.,2.06854248895575));
#21507=CARTESIAN_POINT('Ctrl Pts',(-0.746345871542696,-1.,2.06600523016401));
#21508=CARTESIAN_POINT('Ctrl Pts',(-0.747103932785504,-1.,2.06220058927162));
#21509=CARTESIAN_POINT('Ctrl Pts',(-0.748091554181101,-1.,2.05713023030263));
#21510=CARTESIAN_POINT('Ctrl Pts',(-0.749287468663053,-1.,2.05079645591606));
#21511=CARTESIAN_POINT('Ctrl Pts',(-0.750444657874758,-1.,2.04446689147754));
#21512=CARTESIAN_POINT('Ctrl Pts',(-0.751562963361384,-1.,2.03814160092173));
#21513=CARTESIAN_POINT('Ctrl Pts',(-0.752642180488104,-1.,2.03182068456467));
#21514=CARTESIAN_POINT('Ctrl Pts',(-0.753682061113766,-1.,2.02550428623587));
#21515=CARTESIAN_POINT('Ctrl Pts',(-0.75468233072352,-1.,2.01919259406003));
#21516=CARTESIAN_POINT('Ctrl Pts',(-0.7556427049581,-1.,2.01288584328149));
#21517=CARTESIAN_POINT('Ctrl Pts',(-0.756562904646496,-1.,2.00658431587682));
#21518=CARTESIAN_POINT('Ctrl Pts',(-0.757442676862341,-1.,2.00028834739072));
#21519=CARTESIAN_POINT('Ctrl Pts',(-0.758281796766377,-1.,1.9939983109871));
#21520=CARTESIAN_POINT('Ctrl Pts',(-0.759080037802243,-1.,1.98771456680806));
#21521=CARTESIAN_POINT('Ctrl Pts',(-0.759837147452135,-1.,1.98143741418156));
#21522=CARTESIAN_POINT('Ctrl Pts',(-0.760552825409855,-1.,1.97516705321521));
#21523=CARTESIAN_POINT('Ctrl Pts',(-0.761226690483986,-1.,1.96890351582545));
#21524=CARTESIAN_POINT('Ctrl Pts',(-0.761858300014575,-1.,1.96264672744229));
#21525=CARTESIAN_POINT('Ctrl Pts',(-0.762447203806263,-1.,1.95639665309893));
#21526=CARTESIAN_POINT('Ctrl Pts',(-0.762992990878774,-1.,1.95015342590025));
#21527=CARTESIAN_POINT('Ctrl Pts',(-0.76349533353858,-1.,1.94391746617626));
#21528=CARTESIAN_POINT('Ctrl Pts',(-0.763954049121393,-1.,1.93768964875867));
#21529=CARTESIAN_POINT('Ctrl Pts',(-0.764369010673889,-1.,1.93147105496367));
#21530=CARTESIAN_POINT('Ctrl Pts',(-0.764740025488189,-1.,1.92526263537041));
#21531=CARTESIAN_POINT('Ctrl Pts',(-0.765066729667095,-1.,1.91906491634197));
#21532=CARTESIAN_POINT('Ctrl Pts',(-0.765348465884739,-1.,1.91287765805174));
#21533=CARTESIAN_POINT('Ctrl Pts',(-0.765584196937936,-1.,1.90669961402362));
#21534=CARTESIAN_POINT('Ctrl Pts',(-0.765772772593395,-1.,1.90052930393599));
#21535=CARTESIAN_POINT('Ctrl Pts',(-0.765913193856979,-1.,1.89436577771389));
#21536=CARTESIAN_POINT('Ctrl Pts',(-0.76600483706209,-1.,1.88820926433409));
#21537=CARTESIAN_POINT('Ctrl Pts',(-0.766047794851869,-1.,1.88206215302561));
#21538=CARTESIAN_POINT('Ctrl Pts',(-0.766042837036759,-1.,1.87592888967886));
#21539=CARTESIAN_POINT('Ctrl Pts',(-0.765990708546111,-1.,1.86981398314345));
#21540=CARTESIAN_POINT('Ctrl Pts',(-0.765891519092557,-1.,1.86372027063314));
#21541=CARTESIAN_POINT('Ctrl Pts',(-0.765744212909305,-1.,1.85764741390391));
#21542=CARTESIAN_POINT('Ctrl Pts',(-0.765545710619023,-1.,1.85158945130054));
#21543=CARTESIAN_POINT('Ctrl Pts',(-0.765291664861971,-1.,1.8455369887591));
#21544=CARTESIAN_POINT('Ctrl Pts',(-0.764978057881687,-1.,1.83948181064823));
#21545=CARTESIAN_POINT('Ctrl Pts',(-0.764602549687845,-1.,1.8334207722714));
#21546=CARTESIAN_POINT('Ctrl Pts',(-0.764165902606055,-1.,1.8273599120008));
#21547=CARTESIAN_POINT('Ctrl Pts',(-0.763673465462854,-1.,1.82131873145297));
#21548=CARTESIAN_POINT('Ctrl Pts',(-0.763132003836783,-1.,1.81532118405566));
#21549=CARTESIAN_POINT('Ctrl Pts',(-0.762546129464036,-1.,1.80938551463989));
#21550=CARTESIAN_POINT('Ctrl Pts',(-0.761915336443516,-1.,1.80351583877334));
#21551=CARTESIAN_POINT('Ctrl Pts',(-0.761229695230359,-1.,1.79768986997735));
#21552=CARTESIAN_POINT('Ctrl Pts',(-0.760469555880425,-1.,1.79185815610802));
#21553=CARTESIAN_POINT('Ctrl Pts',(-0.759614401109868,-1.,1.78596964884526));
#21554=CARTESIAN_POINT('Ctrl Pts',(-0.75865062667738,-1.,1.77999411220912));
#21555=CARTESIAN_POINT('Ctrl Pts',(-0.757578264077238,-1.,1.77394167108342));
#21556=CARTESIAN_POINT('Ctrl Pts',(-0.756421896028403,-1.,1.76789396003141));
#21557=CARTESIAN_POINT('Ctrl Pts',(-0.755220979975262,-1.,1.7619781724032));
#21558=CARTESIAN_POINT('Ctrl Pts',(-0.75400925402848,-1.,1.75631083600175));
#21559=CARTESIAN_POINT('Ctrl Pts',(-0.752797683531377,-1.,1.75095139468809));
#21560=CARTESIAN_POINT('Ctrl Pts',(-0.751555614163629,-1.,1.74585086852298));
#21561=CARTESIAN_POINT('Ctrl Pts',(-0.75019343597954,-1.,1.74080458266705));
#21562=CARTESIAN_POINT('Ctrl Pts',(-0.748582462954855,-1.,1.73550351679848));
#21563=CARTESIAN_POINT('Ctrl Pts',(-0.746574710096436,-1.,1.72958533647399));
#21564=CARTESIAN_POINT('Ctrl Pts',(-0.744021445433764,-1.,1.7226822991693));
#21565=CARTESIAN_POINT('Ctrl Pts',(-0.740795162032088,-1.,1.71447789751927));
#21566=CARTESIAN_POINT('Ctrl Pts',(-0.736799665724771,-1.,1.70473309006121));
#21567=CARTESIAN_POINT('Ctrl Pts',(-0.731963238697195,-1.,1.69326921975743));
#21568=CARTESIAN_POINT('Ctrl Pts',(-0.726235967997433,-1.,1.67996158455503));
#21569=CARTESIAN_POINT('Ctrl Pts',(-0.719585433804282,-1.,1.6647288055568));
#21570=CARTESIAN_POINT('Ctrl Pts',(-0.711993139355394,-1.,1.64752408832016));
#21571=CARTESIAN_POINT('Ctrl Pts',(-0.705159151988319,-1.,1.63216541664676));
#21572=CARTESIAN_POINT('Ctrl Pts',(-0.699605146405088,-1.,1.61974673472612));
#21573=CARTESIAN_POINT('Ctrl Pts',(-0.695712097881194,-1.,1.61106790958151));
#21574=CARTESIAN_POINT('Ctrl Pts',(-0.693717979106306,-1.,1.60662857109684));
#21575=CARTESIAN_POINT('',(-0.892032620296855,-1.,1.5055822144029));
#21576=CARTESIAN_POINT('Origin',(0.,-1.,0.));
#21577=CARTESIAN_POINT('',(-1.23627494547115,-1.,1.81978687191668));
#21578=CARTESIAN_POINT('Ctrl Pts',(-0.892032620296855,-1.,1.5055822144029));
#21579=CARTESIAN_POINT('Ctrl Pts',(-0.894452006964543,-1.,1.50980486806688));
#21580=CARTESIAN_POINT('Ctrl Pts',(-0.899185047483511,-1.,1.51805569590094));
#21581=CARTESIAN_POINT('Ctrl Pts',(-0.905967409625651,-1.,1.52984849887993));
#21582=CARTESIAN_POINT('Ctrl Pts',(-0.914375919026456,-1.,1.54440491149498));
#21583=CARTESIAN_POINT('Ctrl Pts',(-0.923832188944341,-1.,1.56065988578893));
#21584=CARTESIAN_POINT('Ctrl Pts',(-0.932246680108685,-1.,1.57499388382243));
#21585=CARTESIAN_POINT('Ctrl Pts',(-0.939646377893399,-1.,1.58744937487176));
#21586=CARTESIAN_POINT('Ctrl Pts',(-0.946078063315257,-1.,1.59810042043673));
#21587=CARTESIAN_POINT('Ctrl Pts',(-0.951613284356035,-1.,1.60706069896936));
#21588=CARTESIAN_POINT('Ctrl Pts',(-0.956354422920671,-1.,1.61449324337085));
#21589=CARTESIAN_POINT('Ctrl Pts',(-0.960438326101729,-1.,1.62061638140221));
#21590=CARTESIAN_POINT('Ctrl Pts',(-0.964046107040536,-1.,1.62571930670187));
#21591=CARTESIAN_POINT('Ctrl Pts',(-0.967387853230345,-1.,1.63013849959461));
#21592=CARTESIAN_POINT('Ctrl Pts',(-0.970669715997509,-1.,1.63420665729798));
#21593=CARTESIAN_POINT('Ctrl Pts',(-0.974066058287418,-1.,1.63820952658144));
#21594=CARTESIAN_POINT('Ctrl Pts',(-0.977689794119416,-1.,1.64233990826687));
#21595=CARTESIAN_POINT('Ctrl Pts',(-0.981562530939489,-1.,1.64665139190656));
#21596=CARTESIAN_POINT('Ctrl Pts',(-0.985642622920821,-1.,1.65110016612638));
#21597=CARTESIAN_POINT('Ctrl Pts',(-0.989855627854165,-1.,1.65559044289699));
#21598=CARTESIAN_POINT('Ctrl Pts',(-0.994121836661306,-1.,1.66001553809947));
#21599=CARTESIAN_POINT('Ctrl Pts',(-0.998389654952758,-1.,1.66430758030376));
#21600=CARTESIAN_POINT('Ctrl Pts',(-1.00265091003727,-1.,1.66846059277303));
#21601=CARTESIAN_POINT('Ctrl Pts',(-1.00692206696414,-1.,1.67250335383293));
#21602=CARTESIAN_POINT('Ctrl Pts',(-1.01123236493511,-1.,1.67648246776464));
#21603=CARTESIAN_POINT('Ctrl Pts',(-1.01561026162773,-1.,1.68044289894798));
#21604=CARTESIAN_POINT('Ctrl Pts',(-1.02006795074201,-1.,1.68440578021706));
#21605=CARTESIAN_POINT('Ctrl Pts',(-1.02460180535255,-1.,1.68836910178447));
#21606=CARTESIAN_POINT('Ctrl Pts',(-1.02919977579147,-1.,1.69231840863458));
#21607=CARTESIAN_POINT('Ctrl Pts',(-1.03384646003588,-1.,1.69623414782771));
#21608=CARTESIAN_POINT('Ctrl Pts',(-1.03852922490789,-1.,1.70010052930962));
#21609=CARTESIAN_POINT('Ctrl Pts',(-1.04324363334554,-1.,1.70391338707982));
#21610=CARTESIAN_POINT('Ctrl Pts',(-1.04799085404995,-1.,1.70767646263649));
#21611=CARTESIAN_POINT('Ctrl Pts',(-1.05277517202855,-1.,1.71139783543989));
#21612=CARTESIAN_POINT('Ctrl Pts',(-1.05760163192479,-1.,1.7150865442702));
#21613=CARTESIAN_POINT('Ctrl Pts',(-1.06247324680647,-1.,1.71874858456904));
#21614=CARTESIAN_POINT('Ctrl Pts',(-1.06738966975462,-1.,1.72238500928453));
#21615=CARTESIAN_POINT('Ctrl Pts',(-1.07234866990252,-1.,1.72599406198488));
#21616=CARTESIAN_POINT('Ctrl Pts',(-1.0773470373727,-1.,1.72957248977424));
#21617=CARTESIAN_POINT('Ctrl Pts',(-1.08238162784749,-1.,1.73311705663407));
#21618=CARTESIAN_POINT('Ctrl Pts',(-1.08745056285427,-1.,1.73662628326091));
#21619=CARTESIAN_POINT('Ctrl Pts',(-1.09255329056493,-1.,1.74010053962247));
#21620=CARTESIAN_POINT('Ctrl Pts',(-1.09768999241225,-1.,1.74354119236208));
#21621=CARTESIAN_POINT('Ctrl Pts',(-1.10286118991143,-1.,1.74695004214923));
#21622=CARTESIAN_POINT('Ctrl Pts',(-1.10806728183007,-1.,1.7503286607592));
#21623=CARTESIAN_POINT('Ctrl Pts',(-1.11330807582551,-1.,1.7536777209463));
#21624=CARTESIAN_POINT('Ctrl Pts',(-1.11858293216763,-1.,1.75699720772105));
#21625=CARTESIAN_POINT('Ctrl Pts',(-1.12389096855086,-1.,1.76028671825096));
#21626=CARTESIAN_POINT('Ctrl Pts',(-1.12923123555075,-1.,1.7635457196617));
#21627=CARTESIAN_POINT('Ctrl Pts',(-1.1346029180462,-1.,1.76677384551862));
#21628=CARTESIAN_POINT('Ctrl Pts',(-1.14000548336975,-1.,1.76997111386769));
#21629=CARTESIAN_POINT('Ctrl Pts',(-1.1454385822692,-1.,1.77313777896194));
#21630=CARTESIAN_POINT('Ctrl Pts',(-1.15090197841515,-1.,1.7762742255701));
#21631=CARTESIAN_POINT('Ctrl Pts',(-1.15639547194698,-1.,1.77938085564275));
#21632=CARTESIAN_POINT('Ctrl Pts',(-1.16191881298499,-1.,1.78245795881009));
#21633=CARTESIAN_POINT('Ctrl Pts',(-1.16747166312303,-1.,1.78550566040443));
#21634=CARTESIAN_POINT('Ctrl Pts',(-1.17305363177328,-1.,1.78852398877616));
#21635=CARTESIAN_POINT('Ctrl Pts',(-1.17866429440809,-1.,1.79151291552689));
#21636=CARTESIAN_POINT('Ctrl Pts',(-1.18430321697432,-1.,1.79447240321515));
#21637=CARTESIAN_POINT('Ctrl Pts',(-1.18996997934445,-1.,1.79740245923478));
#21638=CARTESIAN_POINT('Ctrl Pts',(-1.19566418930242,-1.,1.80030314369879));
#21639=CARTESIAN_POINT('Ctrl Pts',(-1.20138548938974,-1.,1.80317454838603));
#21640=CARTESIAN_POINT('Ctrl Pts',(-1.20713356605475,-1.,1.80601678480707));
#21641=CARTESIAN_POINT('Ctrl Pts',(-1.21290815708314,-1.,1.80882996917129));
#21642=CARTESIAN_POINT('Ctrl Pts',(-1.21870906103557,-1.,1.81161420806656));
#21643=CARTESIAN_POINT('Ctrl Pts',(-1.2245361330495,-1.,1.81436959210434));
#21644=CARTESIAN_POINT('Ctrl Pts',(-1.2292186489137,-1.,1.8165508718364));
#21645=CARTESIAN_POINT('Ctrl Pts',(-1.2327422452705,-1.,1.81817389921279));
#21646=CARTESIAN_POINT('Ctrl Pts',(-1.23509651170476,-1.,1.81925017193666));
#21647=CARTESIAN_POINT('Ctrl Pts',(-1.23627494547115,-1.,1.81978687191668));
#21648=CARTESIAN_POINT('',(-1.34869019493419,-1.,1.73811241238545));
#21649=CARTESIAN_POINT('',(-1.23627494547115,-1.,1.81978687191668));
#21650=CARTESIAN_POINT('',(-1.15624053661742,-1.,1.31362392696032));
#21651=CARTESIAN_POINT('Ctrl Pts',(-1.34869019493419,-1.,1.73811241238545));
#21652=CARTESIAN_POINT('Ctrl Pts',(-1.34854391898045,-1.,1.73682580585691));
#21653=CARTESIAN_POINT('Ctrl Pts',(-1.34824783112887,-1.,1.73425417885907));
#21654=CARTESIAN_POINT('Ctrl Pts',(-1.34779309152035,-1.,1.7304014965394));
#21655=CARTESIAN_POINT('Ctrl Pts',(-1.34716554819527,-1.,1.72527410680674));
#21656=CARTESIAN_POINT('Ctrl Pts',(-1.34634568653227,-1.,1.7188807715049));
#21657=CARTESIAN_POINT('Ctrl Pts',(-1.34549029589416,-1.,1.71250340686822));
#21658=CARTESIAN_POINT('Ctrl Pts',(-1.34459924533831,-1.,1.70614212266738));
#21659=CARTESIAN_POINT('Ctrl Pts',(-1.34367237124483,-1.,1.69979707754427));
#21660=CARTESIAN_POINT('Ctrl Pts',(-1.34270948206319,-1.,1.6934684849687));
#21661=CARTESIAN_POINT('Ctrl Pts',(-1.341710374848,-1.,1.68715660868764));
#21662=CARTESIAN_POINT('Ctrl Pts',(-1.34067485185203,-1.,1.68086176030362));
#21663=CARTESIAN_POINT('Ctrl Pts',(-1.3396027347034,-1.,1.67458429426086));
#21664=CARTESIAN_POINT('Ctrl Pts',(-1.33849388654388,-1.,1.66832460783989));
#21665=CARTESIAN_POINT('Ctrl Pts',(-1.33734820885262,-1.,1.66208312541983));
#21666=CARTESIAN_POINT('Ctrl Pts',(-1.33616559745172,-1.,1.65586025952593));
#21667=CARTESIAN_POINT('Ctrl Pts',(-1.33494590467993,-1.,1.6496563728683));
#21668=CARTESIAN_POINT('Ctrl Pts',(-1.33368890676572,-1.,1.6434717485603));
#21669=CARTESIAN_POINT('Ctrl Pts',(-1.33239425103724,-1.,1.63730653475089));
#21670=CARTESIAN_POINT('Ctrl Pts',(-1.33106149345645,-1.,1.63116079730923));
#21671=CARTESIAN_POINT('Ctrl Pts',(-1.3296901950568,-1.,1.62503464209797));
#21672=CARTESIAN_POINT('Ctrl Pts',(-1.32828000610449,-1.,1.61892832270724));
#21673=CARTESIAN_POINT('Ctrl Pts',(-1.32683074483356,-1.,1.6128423401575));
#21674=CARTESIAN_POINT('Ctrl Pts',(-1.32534250785782,-1.,1.60677758290954));
#21675=CARTESIAN_POINT('Ctrl Pts',(-1.32381550858256,-1.,1.60073511858687));
#21676=CARTESIAN_POINT('Ctrl Pts',(-1.32224985747682,-1.,1.59471591079403));
#21677=CARTESIAN_POINT('Ctrl Pts',(-1.32064537110892,-1.,1.58872057258245));
#21678=CARTESIAN_POINT('Ctrl Pts',(-1.31900135021432,-1.,1.58274907898834));
#21679=CARTESIAN_POINT('Ctrl Pts',(-1.31731642317187,-1.,1.5768005650559));
#21680=CARTESIAN_POINT('Ctrl Pts',(-1.31558903860016,-1.,1.57087397835723));
#21681=CARTESIAN_POINT('Ctrl Pts',(-1.31381795281002,-1.,1.56496872402353));
#21682=CARTESIAN_POINT('Ctrl Pts',(-1.31200264341696,-1.,1.55908521254821));
#21683=CARTESIAN_POINT('Ctrl Pts',(-1.31014393684222,-1.,1.55322568759481));
#21684=CARTESIAN_POINT('Ctrl Pts',(-1.30824393907473,-1.,1.54739413957185));
#21685=CARTESIAN_POINT('Ctrl Pts',(-1.30630475189556,-1.,1.54159462645432));
#21686=CARTESIAN_POINT('Ctrl Pts',(-1.30432735639489,-1.,1.53582981268977));
#21687=CARTESIAN_POINT('Ctrl Pts',(-1.30231064395568,-1.,1.53009970283891));
#21688=CARTESIAN_POINT('Ctrl Pts',(-1.30024984366328,-1.,1.52439957861062));
#21689=CARTESIAN_POINT('Ctrl Pts',(-1.29813791800747,-1.,1.51872184912724));
#21690=CARTESIAN_POINT('Ctrl Pts',(-1.29596850710509,-1.,1.51305994241402));
#21691=CARTESIAN_POINT('Ctrl Pts',(-1.29373841372842,-1.,1.50741159078365));
#21692=CARTESIAN_POINT('Ctrl Pts',(-1.29145022885181,-1.,1.50178230149776));
#21693=CARTESIAN_POINT('Ctrl Pts',(-1.28911506584254,-1.,1.49618896881754));
#21694=CARTESIAN_POINT('Ctrl Pts',(-1.2867467611644,-1.,1.4906522831278));
#21695=CARTESIAN_POINT('Ctrl Pts',(-1.28435533880201,-1.,1.4851881711891));
#21696=CARTESIAN_POINT('Ctrl Pts',(-1.28194158939517,-1.,1.47980070347095));
#21697=CARTESIAN_POINT('Ctrl Pts',(-1.2794891824849,-1.,1.4744717526707));
#21698=CARTESIAN_POINT('Ctrl Pts',(-1.27696414831089,-1.,1.46916035917133));
#21699=CARTESIAN_POINT('Ctrl Pts',(-1.27433119897822,-1.,1.46382431332476));
#21700=CARTESIAN_POINT('Ctrl Pts',(-1.27156805265289,-1.,1.45843906294697));
#21701=CARTESIAN_POINT('Ctrl Pts',(-1.2686778680489,-1.,1.45301422764247));
#21702=CARTESIAN_POINT('Ctrl Pts',(-1.26570925118868,-1.,1.44761985001662));
#21703=CARTESIAN_POINT('Ctrl Pts',(-1.26273903323859,-1.,1.44236470511303));
#21704=CARTESIAN_POINT('Ctrl Pts',(-1.25983531012005,-1.,1.43734919180848));
#21705=CARTESIAN_POINT('Ctrl Pts',(-1.25702687965755,-1.,1.43262645609691));
#21706=CARTESIAN_POINT('Ctrl Pts',(-1.25426945222639,-1.,1.42815938799387));
#21707=CARTESIAN_POINT('Ctrl Pts',(-1.2514145557001,-1.,1.42378102115575));
#21708=CARTESIAN_POINT('Ctrl Pts',(-1.24824430986571,-1.,1.41923722596025));
#21709=CARTESIAN_POINT('Ctrl Pts',(-1.24450600513056,-1.,1.41422913175179));
#21710=CARTESIAN_POINT('Ctrl Pts',(-1.23994455029534,-1.,1.40845295531283));
#21711=CARTESIAN_POINT('Ctrl Pts',(-1.23434087290423,-1.,1.40164708206106));
#21712=CARTESIAN_POINT('Ctrl Pts',(-1.22752961899387,-1.,1.39361389568796));
#21713=CARTESIAN_POINT('Ctrl Pts',(-1.21938737280852,-1.,1.38420564527715));
#21714=CARTESIAN_POINT('Ctrl Pts',(-1.20982812925645,-1.,1.37331915607905));
#21715=CARTESIAN_POINT('Ctrl Pts',(-1.1987959077932,-1.,1.36088705043885));
#21716=CARTESIAN_POINT('Ctrl Pts',(-1.18625865667441,-1.,1.34687054001093));
#21717=CARTESIAN_POINT('Ctrl Pts',(-1.17501305789857,-1.,1.33437539347008));
#21718=CARTESIAN_POINT('Ctrl Pts',(-1.16589330093588,-1.,1.32428080721772));
#21719=CARTESIAN_POINT('Ctrl Pts',(-1.15950888730809,-1.,1.31722977216397));
#21720=CARTESIAN_POINT('Ctrl Pts',(-1.15624053661742,-1.,1.31362392696032));
#21721=CARTESIAN_POINT('',(-1.31362392696033,-1.,1.15624053661742));
#21722=CARTESIAN_POINT('Origin',(0.,-1.,0.));
#21723=CARTESIAN_POINT('',(-1.73811241238545,-1.,1.34869019493419));
#21724=CARTESIAN_POINT('Ctrl Pts',(-1.31362392696033,-1.,1.15624053661742));
#21725=CARTESIAN_POINT('Ctrl Pts',(-1.3172297721596,-1.,1.15950888730433));
#21726=CARTESIAN_POINT('Ctrl Pts',(-1.32428080720544,-1.,1.16589330092532));
#21727=CARTESIAN_POINT('Ctrl Pts',(-1.33437539344842,-1.,1.17501305787994));
#21728=CARTESIAN_POINT('Ctrl Pts',(-1.34687053998157,-1.,1.18625865664915));
#21729=CARTESIAN_POINT('Ctrl Pts',(-1.36088705040677,-1.,1.1987959077656));
#21730=CARTESIAN_POINT('Ctrl Pts',(-1.37331915604962,-1.,1.20982812923113));
#21731=CARTESIAN_POINT('Ctrl Pts',(-1.38420564525391,-1.,1.21938737278853));
#21732=CARTESIAN_POINT('Ctrl Pts',(-1.39361389567257,-1.,1.22752961898063));
#21733=CARTESIAN_POINT('Ctrl Pts',(-1.40164708205345,-1.,1.23434087289768));
#21734=CARTESIAN_POINT('Ctrl Pts',(-1.40845295531151,-1.,1.23994455029421));
#21735=CARTESIAN_POINT('Ctrl Pts',(-1.41422913175437,-1.,1.24450600513278));
#21736=CARTESIAN_POINT('Ctrl Pts',(-1.41923722596421,-1.,1.24824430986911));
#21737=CARTESIAN_POINT('Ctrl Pts',(-1.42378102115911,-1.,1.25141455570299));
#21738=CARTESIAN_POINT('Ctrl Pts',(-1.42815938799555,-1.,1.25426945222783));
#21739=CARTESIAN_POINT('Ctrl Pts',(-1.43262645609679,-1.,1.25702687965744));
#21740=CARTESIAN_POINT('Ctrl Pts',(-1.43734919180719,-1.,1.25983531011894));
#21741=CARTESIAN_POINT('Ctrl Pts',(-1.44236470511145,-1.,1.26273903323723));
#21742=CARTESIAN_POINT('Ctrl Pts',(-1.44761985001544,-1.,1.26570925118767));
#21743=CARTESIAN_POINT('Ctrl Pts',(-1.45301422764205,-1.,1.26867786804854));
#21744=CARTESIAN_POINT('Ctrl Pts',(-1.45843906294725,-1.,1.27156805265312));
#21745=CARTESIAN_POINT('Ctrl Pts',(-1.4638243133254,-1.,1.27433119897877));
#21746=CARTESIAN_POINT('Ctrl Pts',(-1.46916035917197,-1.,1.27696414831144));
#21747=CARTESIAN_POINT('Ctrl Pts',(-1.4744717526711,-1.,1.27948918248524));
#21748=CARTESIAN_POINT('Ctrl Pts',(-1.47980070347102,-1.,1.28194158939522));
#21749=CARTESIAN_POINT('Ctrl Pts',(-1.48518817118891,-1.,1.28435533880184));
#21750=CARTESIAN_POINT('Ctrl Pts',(-1.4906522831275,-1.,1.28674676116415));
#21751=CARTESIAN_POINT('Ctrl Pts',(-1.49618896881729,-1.,1.28911506584232));
#21752=CARTESIAN_POINT('Ctrl Pts',(-1.50178230149764,-1.,1.29145022885171));
#21753=CARTESIAN_POINT('Ctrl Pts',(-1.50741159078367,-1.,1.29373841372843));
#21754=CARTESIAN_POINT('Ctrl Pts',(-1.51305994241412,-1.,1.29596850710518));
#21755=CARTESIAN_POINT('Ctrl Pts',(-1.51872184912735,-1.,1.29813791800757));
#21756=CARTESIAN_POINT('Ctrl Pts',(-1.5243995786107,-1.,1.30024984366334));
#21757=CARTESIAN_POINT('Ctrl Pts',(-1.53009970283893,-1.,1.3023106439557));
#21758=CARTESIAN_POINT('Ctrl Pts',(-1.53582981268976,-1.,1.30432735639487));
#21759=CARTESIAN_POINT('Ctrl Pts',(-1.54159462645428,-1.,1.30630475189553));
#21760=CARTESIAN_POINT('Ctrl Pts',(-1.54739413957183,-1.,1.30824393907471));
#21761=CARTESIAN_POINT('Ctrl Pts',(-1.55322568759481,-1.,1.31014393684221));
#21762=CARTESIAN_POINT('Ctrl Pts',(-1.55908521254822,-1.,1.31200264341696));
#21763=CARTESIAN_POINT('Ctrl Pts',(-1.56496872402352,-1.,1.31381795281002));
#21764=CARTESIAN_POINT('Ctrl Pts',(-1.57087397835721,-1.,1.31558903860015));
#21765=CARTESIAN_POINT('Ctrl Pts',(-1.57680056505585,-1.,1.31731642317183));
#21766=CARTESIAN_POINT('Ctrl Pts',(-1.58274907898829,-1.,1.31900135021428));
#21767=CARTESIAN_POINT('Ctrl Pts',(-1.58872057258244,-1.,1.32064537110891));
#21768=CARTESIAN_POINT('Ctrl Pts',(-1.59471591079408,-1.,1.32224985747686));
#21769=CARTESIAN_POINT('Ctrl Pts',(-1.600735118587,-1.,1.32381550858266));
#21770=CARTESIAN_POINT('Ctrl Pts',(-1.6067775829097,-1.,1.32534250785794));
#21771=CARTESIAN_POINT('Ctrl Pts',(-1.61284234015762,-1.,1.32683074483365));
#21772=CARTESIAN_POINT('Ctrl Pts',(-1.61892832270723,-1.,1.32828000610448));
#21773=CARTESIAN_POINT('Ctrl Pts',(-1.62503464209777,-1.,1.32969019505665));
#21774=CARTESIAN_POINT('Ctrl Pts',(-1.63116079730887,-1.,1.33106149345618));
#21775=CARTESIAN_POINT('Ctrl Pts',(-1.6373065347505,-1.,1.33239425103694));
#21776=CARTESIAN_POINT('Ctrl Pts',(-1.64347174856007,-1.,1.33368890676554));
#21777=CARTESIAN_POINT('Ctrl Pts',(-1.64965637286843,-1.,1.33494590468003));
#21778=CARTESIAN_POINT('Ctrl Pts',(-1.65586025952651,-1.,1.33616559745217));
#21779=CARTESIAN_POINT('Ctrl Pts',(-1.66208312542073,-1.,1.33734820885331));
#21780=CARTESIAN_POINT('Ctrl Pts',(-1.66832460784078,-1.,1.33849388654458));
#21781=CARTESIAN_POINT('Ctrl Pts',(-1.67458429426126,-1.,1.33960273470372));
#21782=CARTESIAN_POINT('Ctrl Pts',(-1.68086176030308,-1.,1.3406748518516));
#21783=CARTESIAN_POINT('Ctrl Pts',(-1.68715660868602,-1.,1.34171037484673));
#21784=CARTESIAN_POINT('Ctrl Pts',(-1.6934684849664,-1.,1.34270948206139));
#21785=CARTESIAN_POINT('Ctrl Pts',(-1.69979707754221,-1.,1.34367237124322));
#21786=CARTESIAN_POINT('Ctrl Pts',(-1.70614212266676,-1.,1.34459924533783));
#21787=CARTESIAN_POINT('Ctrl Pts',(-1.71250340687011,-1.,1.34549029589563));
#21788=CARTESIAN_POINT('Ctrl Pts',(-1.7188807715095,-1.,1.34634568653586));
#21789=CARTESIAN_POINT('Ctrl Pts',(-1.72527410681298,-1.,1.34716554820013));
#21790=CARTESIAN_POINT('Ctrl Pts',(-1.73040149654497,-1.,1.3477930915247));
#21791=CARTESIAN_POINT('Ctrl Pts',(-1.73425417886255,-1.,1.34824783113158));
#21792=CARTESIAN_POINT('Ctrl Pts',(-1.73682580585819,-1.,1.34854391898145));
#21793=CARTESIAN_POINT('Ctrl Pts',(-1.73811241238545,-1.,1.34869019493419));
#21794=CARTESIAN_POINT('',(-1.81978687191668,-1.,1.23627494547115));
#21795=CARTESIAN_POINT('',(-1.73811241238545,-1.,1.34869019493419));
#21796=CARTESIAN_POINT('',(-1.5055822144029,-1.,0.892032620296855));
#21797=CARTESIAN_POINT('Ctrl Pts',(-1.81978687191668,-1.,1.23627494547115));
#21798=CARTESIAN_POINT('Ctrl Pts',(-1.81925017193531,-1.,1.23509651170384));
#21799=CARTESIAN_POINT('Ctrl Pts',(-1.81817389920914,-1.,1.23274224526804));
#21800=CARTESIAN_POINT('Ctrl Pts',(-1.81655087183054,-1.,1.22921864890975));
#21801=CARTESIAN_POINT('Ctrl Pts',(-1.81436959209778,-1.,1.22453613304507));
#21802=CARTESIAN_POINT('Ctrl Pts',(-1.81161420806172,-1.,1.2187090610323));
#21803=CARTESIAN_POINT('Ctrl Pts',(-1.80882996916931,-1.,1.2129081570818));
#21804=CARTESIAN_POINT('Ctrl Pts',(-1.80601678480772,-1.,1.20713356605519));
#21805=CARTESIAN_POINT('Ctrl Pts',(-1.8031745483882,-1.,1.2013854893912));
#21806=CARTESIAN_POINT('Ctrl Pts',(-1.80030314370121,-1.,1.19566418930405));
#21807=CARTESIAN_POINT('Ctrl Pts',(-1.79740245923649,-1.,1.1899699793456));
#21808=CARTESIAN_POINT('Ctrl Pts',(-1.79447240321572,-1.,1.18430321697471));
#21809=CARTESIAN_POINT('Ctrl Pts',(-1.79151291552646,-1.,1.17866429440781));
#21810=CARTESIAN_POINT('Ctrl Pts',(-1.78852398877523,-1.,1.17305363177265));
#21811=CARTESIAN_POINT('Ctrl Pts',(-1.78550566040349,-1.,1.16747166312239));
#21812=CARTESIAN_POINT('Ctrl Pts',(-1.78245795880949,-1.,1.16191881298458));
#21813=CARTESIAN_POINT('Ctrl Pts',(-1.77938085564261,-1.,1.15639547194689));
#21814=CARTESIAN_POINT('Ctrl Pts',(-1.77627422557034,-1.,1.15090197841531));
#21815=CARTESIAN_POINT('Ctrl Pts',(-1.77313777896234,-1.,1.14543858226948));
#21816=CARTESIAN_POINT('Ctrl Pts',(-1.76997111386806,-1.,1.14000548337));
#21817=CARTESIAN_POINT('Ctrl Pts',(-1.76677384551883,-1.,1.13460291804635));
#21818=CARTESIAN_POINT('Ctrl Pts',(-1.76354571966171,-1.,1.12923123555076));
#21819=CARTESIAN_POINT('Ctrl Pts',(-1.76028671825084,-1.,1.12389096855078));
#21820=CARTESIAN_POINT('Ctrl Pts',(-1.75699720772089,-1.,1.11858293216752));
#21821=CARTESIAN_POINT('Ctrl Pts',(-1.75367772094617,-1.,1.11330807582542));
#21822=CARTESIAN_POINT('Ctrl Pts',(-1.75032866075914,-1.,1.10806728183003));
#21823=CARTESIAN_POINT('Ctrl Pts',(-1.74695004214924,-1.,1.10286118991144));
#21824=CARTESIAN_POINT('Ctrl Pts',(-1.74354119236212,-1.,1.09768999241229));
#21825=CARTESIAN_POINT('Ctrl Pts',(-1.74010053962252,-1.,1.09255329056496));
#21826=CARTESIAN_POINT('Ctrl Pts',(-1.73662628326093,-1.,1.08745056285429));
#21827=CARTESIAN_POINT('Ctrl Pts',(-1.73311705663407,-1.,1.08238162784749));
#21828=CARTESIAN_POINT('Ctrl Pts',(-1.72957248977424,-1.,1.0773470373727));
#21829=CARTESIAN_POINT('Ctrl Pts',(-1.72599406198489,-1.,1.07234866990252));
#21830=CARTESIAN_POINT('Ctrl Pts',(-1.72238500928456,-1.,1.06738966975463));
#21831=CARTESIAN_POINT('Ctrl Pts',(-1.71874858456908,-1.,1.0624732468065));
#21832=CARTESIAN_POINT('Ctrl Pts',(-1.71508654427022,-1.,1.05760163192481));
#21833=CARTESIAN_POINT('Ctrl Pts',(-1.71139783543986,-1.,1.05277517202854));
#21834=CARTESIAN_POINT('Ctrl Pts',(-1.70767646263641,-1.,1.0479908540499));
#21835=CARTESIAN_POINT('Ctrl Pts',(-1.70391338707969,-1.,1.04324363334546));
#21836=CARTESIAN_POINT('Ctrl Pts',(-1.70010052930951,-1.,1.03852922490782));
#21837=CARTESIAN_POINT('Ctrl Pts',(-1.69623414782769,-1.,1.03384646003587));
#21838=CARTESIAN_POINT('Ctrl Pts',(-1.69231840863471,-1.,1.02919977579155));
#21839=CARTESIAN_POINT('Ctrl Pts',(-1.68836910178475,-1.,1.02460180535272));
#21840=CARTESIAN_POINT('Ctrl Pts',(-1.68440578021739,-1.,1.02006795074222));
#21841=CARTESIAN_POINT('Ctrl Pts',(-1.6804428989482,-1.,1.01561026162787));
#21842=CARTESIAN_POINT('Ctrl Pts',(-1.67648246776457,-1.,1.01123236493507));
#21843=CARTESIAN_POINT('Ctrl Pts',(-1.67250335383248,-1.,1.00692206696387));
#21844=CARTESIAN_POINT('Ctrl Pts',(-1.66846059277231,-1.,1.00265091003682));
#21845=CARTESIAN_POINT('Ctrl Pts',(-1.66430758030304,-1.,0.998389654952317));
#21846=CARTESIAN_POINT('Ctrl Pts',(-1.66001553809916,-1.,0.994121836661116));
#21847=CARTESIAN_POINT('Ctrl Pts',(-1.65559044289746,-1.,0.98985562785445));
#21848=CARTESIAN_POINT('Ctrl Pts',(-1.6511001661277,-1.,0.985642622921626));
#21849=CARTESIAN_POINT('Ctrl Pts',(-1.64665139190834,-1.,0.981562530940574));
#21850=CARTESIAN_POINT('Ctrl Pts',(-1.64233990826831,-1.,0.977689794120297));
#21851=CARTESIAN_POINT('Ctrl Pts',(-1.63820952658157,-1.,0.974066058287501));
#21852=CARTESIAN_POINT('Ctrl Pts',(-1.63420665729609,-1.,0.970669715996356));
#21853=CARTESIAN_POINT('Ctrl Pts',(-1.63013849959083,-1.,0.967387853228041));
#21854=CARTESIAN_POINT('Ctrl Pts',(-1.6257193066974,-1.,0.964046107037821));
#21855=CARTESIAN_POINT('Ctrl Pts',(-1.62061638139929,-1.,0.960438326099958));
#21856=CARTESIAN_POINT('Ctrl Pts',(-1.61449324337233,-1.,0.956354422921573));
#21857=CARTESIAN_POINT('Ctrl Pts',(-1.60706069897794,-1.,0.951613284361248));
#21858=CARTESIAN_POINT('Ctrl Pts',(-1.59810042045408,-1.,0.946078063325796));
#21859=CARTESIAN_POINT('Ctrl Pts',(-1.58744937489796,-1.,0.939646377909319));
#21860=CARTESIAN_POINT('Ctrl Pts',(-1.57499388385561,-1.,0.932246680128849));
#21861=CARTESIAN_POINT('Ctrl Pts',(-1.56065988582509,-1.,0.923832188966322));
#21862=CARTESIAN_POINT('Ctrl Pts',(-1.54440491152808,-1.,0.91437591904658));
#21863=CARTESIAN_POINT('Ctrl Pts',(-1.52984849890434,-1.,0.905967409640499));
#21864=CARTESIAN_POINT('Ctrl Pts',(-1.51805569591479,-1.,0.89918504749193));
#21865=CARTESIAN_POINT('Ctrl Pts',(-1.50980486807181,-1.,0.894452006967538));
#21866=CARTESIAN_POINT('Ctrl Pts',(-1.5055822144029,-1.,0.892032620296855));
#21867=CARTESIAN_POINT('',(-1.60662857109684,-1.,0.693717979106305));
#21868=CARTESIAN_POINT('Origin',(0.,-1.,0.));
#21869=CARTESIAN_POINT('',(-2.0698113262342,-1.,0.7455743247944));
#21870=CARTESIAN_POINT('Ctrl Pts',(-1.60662857109684,-1.,0.693717979106305));
#21871=CARTESIAN_POINT('Ctrl Pts',(-1.61106790957619,-1.,0.69571209787897));
#21872=CARTESIAN_POINT('Ctrl Pts',(-1.61974673471117,-1.,0.699605146398837));
#21873=CARTESIAN_POINT('Ctrl Pts',(-1.6321654166204,-1.,0.705159151977294));
#21874=CARTESIAN_POINT('Ctrl Pts',(-1.64752408828442,-1.,0.711993139340447));
#21875=CARTESIAN_POINT('Ctrl Pts',(-1.66472880551777,-1.,0.71958543378795));
#21876=CARTESIAN_POINT('Ctrl Pts',(-1.67996158451922,-1.,0.726235967982445));
#21877=CARTESIAN_POINT('Ctrl Pts',(-1.69326921972915,-1.,0.731963238685357));
#21878=CARTESIAN_POINT('Ctrl Pts',(-1.70473309004249,-1.,0.736799665716932));
#21879=CARTESIAN_POINT('Ctrl Pts',(-1.71447789751001,-1.,0.74079516202821));
#21880=CARTESIAN_POINT('Ctrl Pts',(-1.72268229916769,-1.,0.744021445433093));
#21881=CARTESIAN_POINT('Ctrl Pts',(-1.72958533647714,-1.,0.746574710097752));
#21882=CARTESIAN_POINT('Ctrl Pts',(-1.7355035168033,-1.,0.74858246295687));
#21883=CARTESIAN_POINT('Ctrl Pts',(-1.74080458267114,-1.,0.750193435981249));
#21884=CARTESIAN_POINT('Ctrl Pts',(-1.74585086852502,-1.,0.751555614164482));
#21885=CARTESIAN_POINT('Ctrl Pts',(-1.75095139468794,-1.,0.752797683531314));
#21886=CARTESIAN_POINT('Ctrl Pts',(-1.75631083600019,-1.,0.754009254027829));
#21887=CARTESIAN_POINT('Ctrl Pts',(-1.76197817240128,-1.,0.755220979974461));
#21888=CARTESIAN_POINT('Ctrl Pts',(-1.76789396002998,-1.,0.75642189602781));
#21889=CARTESIAN_POINT('Ctrl Pts',(-1.77394167108292,-1.,0.757578264077029));
#21890=CARTESIAN_POINT('Ctrl Pts',(-1.77999411220945,-1.,0.758650626677518));
#21891=CARTESIAN_POINT('Ctrl Pts',(-1.78596964884604,-1.,0.759614401110189));
#21892=CARTESIAN_POINT('Ctrl Pts',(-1.7918581561088,-1.,0.760469555880749));
#21893=CARTESIAN_POINT('Ctrl Pts',(-1.79768986997783,-1.,0.761229695230558));
#21894=CARTESIAN_POINT('Ctrl Pts',(-1.80351583877342,-1.,0.761915336443547));
#21895=CARTESIAN_POINT('Ctrl Pts',(-1.80938551463965,-1.,0.762546129463938));
#21896=CARTESIAN_POINT('Ctrl Pts',(-1.8153211840553,-1.,0.763132003836634));
#21897=CARTESIAN_POINT('Ctrl Pts',(-1.82131873145266,-1.,0.763673465462726));
#21898=CARTESIAN_POINT('Ctrl Pts',(-1.82735991200065,-1.,0.764165902605995));
#21899=CARTESIAN_POINT('Ctrl Pts',(-1.83342077227142,-1.,0.764602549687853));
#21900=CARTESIAN_POINT('Ctrl Pts',(-1.83948181064835,-1.,0.764978057881737));
#21901=CARTESIAN_POINT('Ctrl Pts',(-1.84553698875924,-1.,0.765291664862029));
#21902=CARTESIAN_POINT('Ctrl Pts',(-1.85158945130063,-1.,0.765545710619062));
#21903=CARTESIAN_POINT('Ctrl Pts',(-1.85764741390394,-1.,0.765744212909318));
#21904=CARTESIAN_POINT('Ctrl Pts',(-1.86372027063312,-1.,0.765891519092547));
#21905=CARTESIAN_POINT('Ctrl Pts',(-1.86981398314341,-1.,0.765990708546091));
#21906=CARTESIAN_POINT('Ctrl Pts',(-1.87592888967883,-1.,0.766042837036744));
#21907=CARTESIAN_POINT('Ctrl Pts',(-1.88206215302561,-1.,0.766047794851864));
#21908=CARTESIAN_POINT('Ctrl Pts',(-1.88820926433409,-1.,0.766004837062091));
#21909=CARTESIAN_POINT('Ctrl Pts',(-1.89436577771388,-1.,0.765913193856978));
#21910=CARTESIAN_POINT('Ctrl Pts',(-1.90052930393596,-1.,0.765772772593386));
#21911=CARTESIAN_POINT('Ctrl Pts',(-1.90669961402356,-1.,0.765584196937919));
#21912=CARTESIAN_POINT('Ctrl Pts',(-1.91287765805169,-1.,0.765348465884722));
#21913=CARTESIAN_POINT('Ctrl Pts',(-1.91906491634196,-1.,0.765066729667088));
#21914=CARTESIAN_POINT('Ctrl Pts',(-1.92526263537048,-1.,0.764740025488211));
#21915=CARTESIAN_POINT('Ctrl Pts',(-1.93147105496382,-1.,0.76436901067394));
#21916=CARTESIAN_POINT('Ctrl Pts',(-1.93768964875886,-1.,0.763954049121458));
#21917=CARTESIAN_POINT('Ctrl Pts',(-1.9439174661764,-1.,0.763495333538629));
#21918=CARTESIAN_POINT('Ctrl Pts',(-1.95015342590024,-1.,0.762992990878769));
#21919=CARTESIAN_POINT('Ctrl Pts',(-1.95639665309869,-1.,0.762447203806179));
#21920=CARTESIAN_POINT('Ctrl Pts',(-1.96264672744186,-1.,0.761858300014423));
#21921=CARTESIAN_POINT('Ctrl Pts',(-1.96890351582499,-1.,0.76122669048382));
#21922=CARTESIAN_POINT('Ctrl Pts',(-1.97516705321494,-1.,0.760552825409757));
#21923=CARTESIAN_POINT('Ctrl Pts',(-1.98143741418172,-1.,0.75983714745219));
#21924=CARTESIAN_POINT('Ctrl Pts',(-1.98771456680874,-1.,0.759080037802488));
#21925=CARTESIAN_POINT('Ctrl Pts',(-1.99399831098817,-1.,0.758281796766761));
#21926=CARTESIAN_POINT('Ctrl Pts',(-2.00028834739178,-1.,0.757442676862724));
#21927=CARTESIAN_POINT('Ctrl Pts',(-2.0065843158773,-1.,0.75656290464667));
#21928=CARTESIAN_POINT('Ctrl Pts',(-2.01288584328084,-1.,0.755642704957865));
#21929=CARTESIAN_POINT('Ctrl Pts',(-2.01919259405809,-1.,0.754682330722816));
#21930=CARTESIAN_POINT('Ctrl Pts',(-2.02550428623313,-1.,0.753682061112768));
#21931=CARTESIAN_POINT('Ctrl Pts',(-2.03182068456221,-1.,0.752642180487211));
#21932=CARTESIAN_POINT('Ctrl Pts',(-2.03814160092099,-1.,0.751562963361115));
#21933=CARTESIAN_POINT('Ctrl Pts',(-2.04446689147979,-1.,0.750444657875576));
#21934=CARTESIAN_POINT('Ctrl Pts',(-2.05079645592154,-1.,0.749287468665046));
#21935=CARTESIAN_POINT('Ctrl Pts',(-2.05713023031006,-1.,0.748091554183802));
#21936=CARTESIAN_POINT('Ctrl Pts',(-2.06220058927826,-1.,0.747103932787919));
#21937=CARTESIAN_POINT('Ctrl Pts',(-2.06600523016815,-1.,0.7463458715442));
#21938=CARTESIAN_POINT('Ctrl Pts',(-2.06854248895728,-1.,0.745832791378367));
#21939=CARTESIAN_POINT('Ctrl Pts',(-2.0698113262342,-1.,0.7455743247944));
#21940=CARTESIAN_POINT('',(-2.11275013067528,-1.,0.61342227326009));
#21941=CARTESIAN_POINT('',(-2.0698113262342,-1.,0.7455743247944));
#21942=CARTESIAN_POINT('',(-1.7075470150345,-1.,0.383122945602004));
#21943=CARTESIAN_POINT('Ctrl Pts',(-2.11275013067528,-1.,0.61342227326009));
#21944=CARTESIAN_POINT('Ctrl Pts',(-2.11187554259986,-1.,0.6124673655618));
#21945=CARTESIAN_POINT('Ctrl Pts',(-2.11012443807238,-1.,0.610560911689899));
#21946=CARTESIAN_POINT('Ctrl Pts',(-2.1074919961518,-1.,0.607711315454876));
#21947=CARTESIAN_POINT('Ctrl Pts',(-2.10397049886949,-1.,0.60393203073603));
#21948=CARTESIAN_POINT('Ctrl Pts',(-2.0995493086477,-1.,0.599241616420533));
#21949=CARTESIAN_POINT('Ctrl Pts',(-2.0951087622027,-1.,0.594585006052162));
#21950=CARTESIAN_POINT('Ctrl Pts',(-2.09064881812129,-1.,0.589962365403406));
#21951=CARTESIAN_POINT('Ctrl Pts',(-2.08616943727951,-1.,0.585373918991617));
#21952=CARTESIAN_POINT('Ctrl Pts',(-2.08167059018418,-1.,0.580819952108063));
#21953=CARTESIAN_POINT('Ctrl Pts',(-2.07715226767559,-1.,0.576300797416844));
#21954=CARTESIAN_POINT('Ctrl Pts',(-2.07261449292824,-1.,0.571816823242603));
#21955=CARTESIAN_POINT('Ctrl Pts',(-2.06805732997334,-1.,0.567368421181087));
#21956=CARTESIAN_POINT('Ctrl Pts',(-2.06348090160589,-1.,0.562955993082261));
#21957=CARTESIAN_POINT('Ctrl Pts',(-2.05888537756462,-1.,0.558579940185151));
#21958=CARTESIAN_POINT('Ctrl Pts',(-2.05427091604413,-1.,0.554240657463906));
#21959=CARTESIAN_POINT('Ctrl Pts',(-2.04963761077958,-1.,0.549938525150295));
#21960=CARTESIAN_POINT('Ctrl Pts',(-2.04498544714588,-1.,0.54567390381743));
#21961=CARTESIAN_POINT('Ctrl Pts',(-2.04031422690527,-1.,0.541447120615659));
#21962=CARTESIAN_POINT('Ctrl Pts',(-2.03562362954037,-1.,0.537258489833262));
#21963=CARTESIAN_POINT('Ctrl Pts',(-2.03091336214426,-1.,0.533108355132976));
#21964=CARTESIAN_POINT('Ctrl Pts',(-2.0261832908329,-1.,0.528997127241914));
#21965=CARTESIAN_POINT('Ctrl Pts',(-2.02143356304698,-1.,0.524925318333476));
#21966=CARTESIAN_POINT('Ctrl Pts',(-2.01666477917286,-1.,0.52089359039937));
#21967=CARTESIAN_POINT('Ctrl Pts',(-2.01187773939242,-1.,0.516902681728687));
#21968=CARTESIAN_POINT('Ctrl Pts',(-2.00707309946949,-1.,0.512953306961792));
#21969=CARTESIAN_POINT('Ctrl Pts',(-2.00225107134734,-1.,0.509046069886157));
#21970=CARTESIAN_POINT('Ctrl Pts',(-1.99741107463572,-1.,0.505181361323026));
#21971=CARTESIAN_POINT('Ctrl Pts',(-1.99255149126155,-1.,0.501359287727146));
#21972=CARTESIAN_POINT('Ctrl Pts',(-1.98767044752932,-1.,0.497579909545574));
#21973=CARTESIAN_POINT('Ctrl Pts',(-1.98276658761821,-1.,0.493843476541494));
#21974=CARTESIAN_POINT('Ctrl Pts',(-1.97783973019229,-1.,0.490150627860952));
#21975=CARTESIAN_POINT('Ctrl Pts',(-1.97289186263272,-1.,0.486502692907659));
#21976=CARTESIAN_POINT('Ctrl Pts',(-1.96792703422362,-1.,0.48290166212069));
#21977=CARTESIAN_POINT('Ctrl Pts',(-1.96294933055943,-1.,0.479349583074855));
#21978=CARTESIAN_POINT('Ctrl Pts',(-1.95796111148177,-1.,0.475848034683176));
#21979=CARTESIAN_POINT('Ctrl Pts',(-1.95296148278133,-1.,0.472397672264072));
#21980=CARTESIAN_POINT('Ctrl Pts',(-1.94794381136514,-1.,0.468997482913135));
#21981=CARTESIAN_POINT('Ctrl Pts',(-1.9428979419619,-1.,0.46564546202603));
#21982=CARTESIAN_POINT('Ctrl Pts',(-1.93781486640821,-1.,0.462340031009056));
#21983=CARTESIAN_POINT('Ctrl Pts',(-1.93269066517934,-1.,0.459081234547926));
#21984=CARTESIAN_POINT('Ctrl Pts',(-1.92753067150476,-1.,0.455872005174371));
#21985=CARTESIAN_POINT('Ctrl Pts',(-1.92235380648502,-1.,0.452719478359432));
#21986=CARTESIAN_POINT('Ctrl Pts',(-1.91718342555755,-1.,0.449632260106662));
#21987=CARTESIAN_POINT('Ctrl Pts',(-1.9120369998112,-1.,0.446617343485711));
#21988=CARTESIAN_POINT('Ctrl Pts',(-1.90691756144898,-1.,0.44367755684915));
#21989=CARTESIAN_POINT('Ctrl Pts',(-1.90180124389086,-1.,0.440807833704038));
#21990=CARTESIAN_POINT('Ctrl Pts',(-1.89663648956466,-1.,0.437995003948244));
#21991=CARTESIAN_POINT('Ctrl Pts',(-1.89136993975504,-1.,0.435225660963383));
#21992=CARTESIAN_POINT('Ctrl Pts',(-1.88596913666793,-1.,0.432493038548748));
#21993=CARTESIAN_POINT('Ctrl Pts',(-1.88044229001832,-1.,0.429803062482344));
#21994=CARTESIAN_POINT('Ctrl Pts',(-1.87486989291484,-1.,0.427183828519102));
#21995=CARTESIAN_POINT('Ctrl Pts',(-1.86937803944323,-1.,0.424678177291359));
#21996=CARTESIAN_POINT('Ctrl Pts',(-1.86408083334028,-1.,0.422327307418275));
#21997=CARTESIAN_POINT('Ctrl Pts',(-1.85903281096686,-1.,0.420157287975619));
#21998=CARTESIAN_POINT('Ctrl Pts',(-1.85417632856234,-1.,0.418164129143534));
#21999=CARTESIAN_POINT('Ctrl Pts',(-1.84929312929882,-1.,0.416300022038864));
#22000=CARTESIAN_POINT('Ctrl Pts',(-1.8440575707371,-1.,0.41448743825434));
#22001=CARTESIAN_POINT('Ctrl Pts',(-1.83808953475839,-1.,0.412633125322161));
#22002=CARTESIAN_POINT('Ctrl Pts',(-1.83100408895216,-1.,0.410641256301675));
#22003=CARTESIAN_POINT('Ctrl Pts',(-1.8224702267854,-1.,0.408428948108533));
#22004=CARTESIAN_POINT('Ctrl Pts',(-1.81223801813988,-1.,0.405933518411838));
#22005=CARTESIAN_POINT('Ctrl Pts',(-1.80012077176221,-1.,0.403107976170441));
#22006=CARTESIAN_POINT('Ctrl Pts',(-1.78598826347533,-1.,0.39991940378308));
#22007=CARTESIAN_POINT('Ctrl Pts',(-1.7697556004756,-1.,0.39634619612042));
#22008=CARTESIAN_POINT('Ctrl Pts',(-1.75137405313962,-1.,0.392375812294307));
#22009=CARTESIAN_POINT('Ctrl Pts',(-1.7349317097561,-1.,0.388877023509191));
#22010=CARTESIAN_POINT('Ctrl Pts',(-1.72162022246158,-1.,0.38607079032701));
#22011=CARTESIAN_POINT('Ctrl Pts',(-1.71231062891958,-1.,0.384119047315542));
#22012=CARTESIAN_POINT('Ctrl Pts',(-1.7075470150345,-1.,0.383122945602004));
#22013=CARTESIAN_POINT('',(-1.74236521665491,-1.,0.163289472382896));
#22014=CARTESIAN_POINT('Origin',(0.,-1.,0.));
#22015=CARTESIAN_POINT('',(-2.19890268624765,-1.,0.069476445021958));
#22016=CARTESIAN_POINT('Ctrl Pts',(-1.74236521665491,-1.,0.163289472382896));
#22017=CARTESIAN_POINT('Ctrl Pts',(-1.7472034950333,-1.,0.163814161002002));
#22018=CARTESIAN_POINT('Ctrl Pts',(-1.75666056638427,-1.,0.164834765707158));
#22019=CARTESIAN_POINT('Ctrl Pts',(-1.77018771684844,-1.,0.1662793551464));
#22020=CARTESIAN_POINT('Ctrl Pts',(-1.7869064998507,-1.,0.168032772805197));
#22021=CARTESIAN_POINT('Ctrl Pts',(-1.80561530629706,-1.,0.169936923904608));
#22022=CARTESIAN_POINT('Ctrl Pts',(-1.82215766811545,-1.,0.171554770204119));
#22023=CARTESIAN_POINT('Ctrl Pts',(-1.83658380527692,-1.,0.1728894428919));
#22024=CARTESIAN_POINT('Ctrl Pts',(-1.8489811319852,-1.,0.173946627587731));
#22025=CARTESIAN_POINT('Ctrl Pts',(-1.85948367088837,-1.,0.17473525927603));
#22026=CARTESIAN_POINT('Ctrl Pts',(-1.86828349694799,-1.,0.175268337590758));
#22027=CARTESIAN_POINT('Ctrl Pts',(-1.87563767773588,-1.,0.175563480746485));
#22028=CARTESIAN_POINT('Ctrl Pts',(-1.88188663145367,-1.,0.175644148889698));
#22029=CARTESIAN_POINT('Ctrl Pts',(-1.88742606273259,-1.,0.175538155840648));
#22030=CARTESIAN_POINT('Ctrl Pts',(-1.892646301985,-1.,0.175274276190844));
#22031=CARTESIAN_POINT('Ctrl Pts',(-1.89788101117132,-1.,0.174879405091263));
#22032=CARTESIAN_POINT('Ctrl Pts',(-1.90335253862834,-1.,0.174375518661085));
#22033=CARTESIAN_POINT('Ctrl Pts',(-1.90911693975267,-1.,0.173776635257817));
#22034=CARTESIAN_POINT('Ctrl Pts',(-1.91511429159527,-1.,0.173090695383496));
#22035=CARTESIAN_POINT('Ctrl Pts',(-1.9212233439798,-1.,0.172321621259514));
#22036=CARTESIAN_POINT('Ctrl Pts',(-1.92731093582036,-1.,0.171471191532988));
#22037=CARTESIAN_POINT('Ctrl Pts',(-1.93329183155539,-1.,0.170541253116201));
#22038=CARTESIAN_POINT('Ctrl Pts',(-1.93915639211581,-1.,0.169534904817491));
#22039=CARTESIAN_POINT('Ctrl Pts',(-1.94493757756931,-1.,0.168455741607556));
#22040=CARTESIAN_POINT('Ctrl Pts',(-1.95069027794294,-1.,0.167307501784475));
#22041=CARTESIAN_POINT('Ctrl Pts',(-1.9564675971873,-1.,0.166093592002812));
#22042=CARTESIAN_POINT('Ctrl Pts',(-1.96229379940136,-1.,0.164816568920269));
#22043=CARTESIAN_POINT('Ctrl Pts',(-1.96816512677967,-1.,0.163478185457734));
#22044=CARTESIAN_POINT('Ctrl Pts',(-1.97406280235188,-1.,0.162079693556288));
#22045=CARTESIAN_POINT('Ctrl Pts',(-1.97996195437559,-1.,0.160622060784611));
#22046=CARTESIAN_POINT('Ctrl Pts',(-1.98584238283292,-1.,0.159106226437299));
#22047=CARTESIAN_POINT('Ctrl Pts',(-1.99169810931908,-1.,0.157533331459227));
#22048=CARTESIAN_POINT('Ctrl Pts',(-1.99753284771497,-1.,0.155904629548783));
#22049=CARTESIAN_POINT('Ctrl Pts',(-2.00335565310543,-1.,0.154221403049722));
#22050=CARTESIAN_POINT('Ctrl Pts',(-2.00917680318424,-1.,0.15248488362145));
#22051=CARTESIAN_POINT('Ctrl Pts',(-2.01500291940238,-1.,0.150696157673078));
#22052=CARTESIAN_POINT('Ctrl Pts',(-2.02083464969894,-1.,0.148856124775337));
#22053=CARTESIAN_POINT('Ctrl Pts',(-2.02666926182017,-1.,0.146965557332583));
#22054=CARTESIAN_POINT('Ctrl Pts',(-2.03250223739942,-1.,0.145025140186057));
#22055=CARTESIAN_POINT('Ctrl Pts',(-2.03832911025912,-1.,0.143035515058209));
#22056=CARTESIAN_POINT('Ctrl Pts',(-2.04414757947916,-1.,0.140997332152546));
#22057=CARTESIAN_POINT('Ctrl Pts',(-2.04995762001328,-1.,0.138911255368966));
#22058=CARTESIAN_POINT('Ctrl Pts',(-2.05576044414264,-1.,0.136777941218043));
#22059=CARTESIAN_POINT('Ctrl Pts',(-2.06155781517842,-1.,0.134598026192106));
#22060=CARTESIAN_POINT('Ctrl Pts',(-2.06735123910326,-1.,0.13237211154771));
#22061=CARTESIAN_POINT('Ctrl Pts',(-2.07314114713063,-1.,0.130100748328403));
#22062=CARTESIAN_POINT('Ctrl Pts',(-2.07892715110987,-1.,0.12778444527612));
#22063=CARTESIAN_POINT('Ctrl Pts',(-2.08470840653643,-1.,0.125423679412061));
#22064=CARTESIAN_POINT('Ctrl Pts',(-2.09048392424825,-1.,0.123018905621083));
#22065=CARTESIAN_POINT('Ctrl Pts',(-2.0962529286773,-1.,0.120570567965122));
#22066=CARTESIAN_POINT('Ctrl Pts',(-2.102015121329,-1.,0.118079107988355));
#22067=CARTESIAN_POINT('Ctrl Pts',(-2.10777050261309,-1.,0.115544957687926));
#22068=CARTESIAN_POINT('Ctrl Pts',(-2.11351924490306,-1.,0.112968534419737));
#22069=CARTESIAN_POINT('Ctrl Pts',(-2.11926155590865,-1.,0.110350236135025));
#22070=CARTESIAN_POINT('Ctrl Pts',(-2.12499752307,-1.,0.10769043523109));
#22071=CARTESIAN_POINT('Ctrl Pts',(-2.13072704887293,-1.,0.104989479152739));
#22072=CARTESIAN_POINT('Ctrl Pts',(-2.13644992667165,-1.,0.1022477005561));
#22073=CARTESIAN_POINT('Ctrl Pts',(-2.14216588396025,-1.,0.0994654261990914));
#22074=CARTESIAN_POINT('Ctrl Pts',(-2.14787463531795,-1.,0.0966429852305457));
#22075=CARTESIAN_POINT('Ctrl Pts',(-2.1535759397817,-1.,0.0937807218867642));
#22076=CARTESIAN_POINT('Ctrl Pts',(-2.15926961544516,-1.,0.0908789888107264));
#22077=CARTESIAN_POINT('Ctrl Pts',(-2.16495552645014,-1.,0.0879381291386921));
#22078=CARTESIAN_POINT('Ctrl Pts',(-2.17063357870952,-1.,0.0849584620835371));
#22079=CARTESIAN_POINT('Ctrl Pts',(-2.176303712113,-1.,0.0819402680872764));
#22080=CARTESIAN_POINT('Ctrl Pts',(-2.18196589448887,-1.,0.0788837727685241));
#22081=CARTESIAN_POINT('Ctrl Pts',(-2.1876201139953,-1.,0.0757891465836146));
#22082=CARTESIAN_POINT('Ctrl Pts',(-2.19213712013662,-1.,0.0732830357306724));
#22083=CARTESIAN_POINT('Ctrl Pts',(-2.19552129484002,-1.,0.0713863779526153));
#22084=CARTESIAN_POINT('Ctrl Pts',(-2.19777582085423,-1.,0.0701143536325489));
#22085=CARTESIAN_POINT('Ctrl Pts',(-2.19890268624765,-1.,0.069476445021958));
#22086=CARTESIAN_POINT('',(-2.19890268624765,-1.,-0.0694764450219585));
#22087=CARTESIAN_POINT('',(-2.19890268624765,-1.,0.069476445021958));
#22088=CARTESIAN_POINT('',(-1.74236521665491,-1.,-0.163289472382896));
#22089=CARTESIAN_POINT('Ctrl Pts',(-2.19890268624765,-1.,-0.0694764450219585));
#22090=CARTESIAN_POINT('Ctrl Pts',(-2.19777582085261,-1.,-0.0701143536324927));
#22091=CARTESIAN_POINT('Ctrl Pts',(-2.19552129483562,-1.,-0.0713863779524629));
#22092=CARTESIAN_POINT('Ctrl Pts',(-2.19213712012956,-1.,-0.0732830357304277));
#22093=CARTESIAN_POINT('Ctrl Pts',(-2.1876201139874,-1.,-0.0757891465833413));
#22094=CARTESIAN_POINT('Ctrl Pts',(-2.18196589448304,-1.,-0.0788837727683229));
#22095=CARTESIAN_POINT('Ctrl Pts',(-2.1763037121106,-1.,-0.0819402680871941));
#22096=CARTESIAN_POINT('Ctrl Pts',(-2.17063357871031,-1.,-0.0849584620835644));
#22097=CARTESIAN_POINT('Ctrl Pts',(-2.16495552645275,-1.,-0.0879381291387824));
#22098=CARTESIAN_POINT('Ctrl Pts',(-2.15926961544808,-1.,-0.0908789888108267));
#22099=CARTESIAN_POINT('Ctrl Pts',(-2.15357593978377,-1.,-0.0937807218868346));
#22100=CARTESIAN_POINT('Ctrl Pts',(-2.14787463531864,-1.,-0.096642985230569));
#22101=CARTESIAN_POINT('Ctrl Pts',(-2.14216588395974,-1.,-0.0994654261990744));
#22102=CARTESIAN_POINT('Ctrl Pts',(-2.13644992667052,-1.,-0.102247700556064));
#22103=CARTESIAN_POINT('Ctrl Pts',(-2.1307270488718,-1.,-0.104989479152703));
#22104=CARTESIAN_POINT('Ctrl Pts',(-2.12499752306927,-1.,-0.107690435231068));
#22105=CARTESIAN_POINT('Ctrl Pts',(-2.11926155590849,-1.,-0.11035023613502));
#22106=CARTESIAN_POINT('Ctrl Pts',(-2.11351924490335,-1.,-0.112968534419746));
#22107=CARTESIAN_POINT('Ctrl Pts',(-2.10777050261359,-1.,-0.11554495768794));
#22108=CARTESIAN_POINT('Ctrl Pts',(-2.10201512132945,-1.,-0.118079107988368));
#22109=CARTESIAN_POINT('Ctrl Pts',(-2.09625292867756,-1.,-0.120570567965129));
#22110=CARTESIAN_POINT('Ctrl Pts',(-2.09048392424826,-1.,-0.123018905621083));
#22111=CARTESIAN_POINT('Ctrl Pts',(-2.08470840653628,-1.,-0.125423679412058));
#22112=CARTESIAN_POINT('Ctrl Pts',(-2.07892715110967,-1.,-0.127784445276116));
#22113=CARTESIAN_POINT('Ctrl Pts',(-2.07314114713047,-1.,-0.130100748328401));
#22114=CARTESIAN_POINT('Ctrl Pts',(-2.06735123910319,-1.,-0.13237211154771));
#22115=CARTESIAN_POINT('Ctrl Pts',(-2.06155781517844,-1.,-0.134598026192107));
#22116=CARTESIAN_POINT('Ctrl Pts',(-2.0557604441427,-1.,-0.136777941218044));
#22117=CARTESIAN_POINT('Ctrl Pts',(-2.04995762001333,-1.,-0.138911255368966));
#22118=CARTESIAN_POINT('Ctrl Pts',(-2.04414757947919,-1.,-0.140997332152545));
#22119=CARTESIAN_POINT('Ctrl Pts',(-2.03832911025913,-1.,-0.143035515058208));
#22120=CARTESIAN_POINT('Ctrl Pts',(-2.03250223739941,-1.,-0.145025140186058));
#22121=CARTESIAN_POINT('Ctrl Pts',(-2.02666926182017,-1.,-0.146965557332586));
#22122=CARTESIAN_POINT('Ctrl Pts',(-2.02083464969897,-1.,-0.148856124775343));
#22123=CARTESIAN_POINT('Ctrl Pts',(-2.01500291940243,-1.,-0.150696157673084));
#22124=CARTESIAN_POINT('Ctrl Pts',(-2.00917680318426,-1.,-0.152484883621452));
#22125=CARTESIAN_POINT('Ctrl Pts',(-2.00335565310539,-1.,-0.154221403049719));
#22126=CARTESIAN_POINT('Ctrl Pts',(-1.99753284771487,-1.,-0.155904629548775));
#22127=CARTESIAN_POINT('Ctrl Pts',(-1.99169810931893,-1.,-0.157533331459215));
#22128=CARTESIAN_POINT('Ctrl Pts',(-1.98584238283279,-1.,-0.159106226437289));
#22129=CARTESIAN_POINT('Ctrl Pts',(-1.97996195437557,-1.,-0.16062206078461));
#22130=CARTESIAN_POINT('Ctrl Pts',(-1.97406280235204,-1.,-0.162079693556302));
#22131=CARTESIAN_POINT('Ctrl Pts',(-1.96816512678,-1.,-0.16347818545776));
#22132=CARTESIAN_POINT('Ctrl Pts',(-1.96229379940174,-1.,-0.1648165689203));
#22133=CARTESIAN_POINT('Ctrl Pts',(-1.95646759718755,-1.,-0.166093592002833));
#22134=CARTESIAN_POINT('Ctrl Pts',(-1.95069027794286,-1.,-0.167307501784469));
#22135=CARTESIAN_POINT('Ctrl Pts',(-1.94493757756879,-1.,-0.168455741607516));
#22136=CARTESIAN_POINT('Ctrl Pts',(-1.93915639211497,-1.,-0.169534904817425));
#22137=CARTESIAN_POINT('Ctrl Pts',(-1.93329183155455,-1.,-0.170541253116136));
#22138=CARTESIAN_POINT('Ctrl Pts',(-1.92731093582,-1.,-0.17147119153296));
#22139=CARTESIAN_POINT('Ctrl Pts',(-1.92122334398034,-1.,-0.172321621259557));
#22140=CARTESIAN_POINT('Ctrl Pts',(-1.91511429159681,-1.,-0.173090695383619));
#22141=CARTESIAN_POINT('Ctrl Pts',(-1.90911693975475,-1.,-0.173776635257984));
#22142=CARTESIAN_POINT('Ctrl Pts',(-1.90335253863003,-1.,-0.174375518661222));
#22143=CARTESIAN_POINT('Ctrl Pts',(-1.89788101117148,-1.,-0.174879405091277));
#22144=CARTESIAN_POINT('Ctrl Pts',(-1.89264630198279,-1.,-0.175274276190664));
#22145=CARTESIAN_POINT('Ctrl Pts',(-1.88742606272818,-1.,-0.175538155840286));
#22146=CARTESIAN_POINT('Ctrl Pts',(-1.88188663144846,-1.,-0.175644148889271));
#22147=CARTESIAN_POINT('Ctrl Pts',(-1.87563767773249,-1.,-0.175563480746205));
#22148=CARTESIAN_POINT('Ctrl Pts',(-1.86828349694972,-1.,-0.175268337590901));
#22149=CARTESIAN_POINT('Ctrl Pts',(-1.85948367089838,-1.,-0.174735259276856));
#22150=CARTESIAN_POINT('Ctrl Pts',(-1.84898113200543,-1.,-0.173946627589401));
#22151=CARTESIAN_POINT('Ctrl Pts',(-1.83658380530747,-1.,-0.17288944289442));
#22152=CARTESIAN_POINT('Ctrl Pts',(-1.82215766815414,-1.,-0.171554770207306));
#22153=CARTESIAN_POINT('Ctrl Pts',(-1.80561530633924,-1.,-0.169936923908078));
#22154=CARTESIAN_POINT('Ctrl Pts',(-1.78690649988931,-1.,-0.16803277280837));
#22155=CARTESIAN_POINT('Ctrl Pts',(-1.77018771687692,-1.,-0.166279355148738));
#22156=CARTESIAN_POINT('Ctrl Pts',(-1.75666056640041,-1.,-0.164834765708484));
#22157=CARTESIAN_POINT('Ctrl Pts',(-1.74720349503904,-1.,-0.163814161002474));
#22158=CARTESIAN_POINT('Ctrl Pts',(-1.74236521665491,-1.,-0.163289472382896));
#22159=CARTESIAN_POINT('',(-1.7075470150345,-1.,-0.383122945602004));
#22160=CARTESIAN_POINT('Origin',(0.,-1.,0.));
#22161=CARTESIAN_POINT('',(-2.11275013067528,-1.,-0.61342227326009));
#22162=CARTESIAN_POINT('Ctrl Pts',(-1.7075470150345,-1.,-0.383122945602004));
#22163=CARTESIAN_POINT('Ctrl Pts',(-1.71231062891398,-1.,-0.384119047314215));
#22164=CARTESIAN_POINT('Ctrl Pts',(-1.72162022244582,-1.,-0.386070790323281));
#22165=CARTESIAN_POINT('Ctrl Pts',(-1.73493170972829,-1.,-0.388877023502615));
#22166=CARTESIAN_POINT('Ctrl Pts',(-1.75137405310193,-1.,-0.392375812285395));
#22167=CARTESIAN_POINT('Ctrl Pts',(-1.76975560043442,-1.,-0.396346196110688));
#22168=CARTESIAN_POINT('Ctrl Pts',(-1.78598826343754,-1.,-0.399919403774155));
#22169=CARTESIAN_POINT('Ctrl Pts',(-1.80012077173238,-1.,-0.403107976163396));
#22170=CARTESIAN_POINT('Ctrl Pts',(-1.81223801812013,-1.,-0.405933518407175));
#22171=CARTESIAN_POINT('Ctrl Pts',(-1.82247022677562,-1.,-0.408428948106227));
#22172=CARTESIAN_POINT('Ctrl Pts',(-1.83100408895047,-1.,-0.410641256301276));
#22173=CARTESIAN_POINT('Ctrl Pts',(-1.8380895347617,-1.,-0.412633125322945));
#22174=CARTESIAN_POINT('Ctrl Pts',(-1.84405757074218,-1.,-0.414487438255542));
#22175=CARTESIAN_POINT('Ctrl Pts',(-1.84929312930314,-1.,-0.416300022039885));
#22176=CARTESIAN_POINT('Ctrl Pts',(-1.8541763285645,-1.,-0.418164129144045));
#22177=CARTESIAN_POINT('Ctrl Pts',(-1.8590328109667,-1.,-0.420157287975583));
#22178=CARTESIAN_POINT('Ctrl Pts',(-1.86408083333863,-1.,-0.422327307417884));
#22179=CARTESIAN_POINT('Ctrl Pts',(-1.8693780394412,-1.,-0.424678177290876));
#22180=CARTESIAN_POINT('Ctrl Pts',(-1.87486989291333,-1.,-0.427183828518743));
#22181=CARTESIAN_POINT('Ctrl Pts',(-1.88044229001778,-1.,-0.429803062482217));
#22182=CARTESIAN_POINT('Ctrl Pts',(-1.88596913666828,-1.,-0.432493038548833));
#22183=CARTESIAN_POINT('Ctrl Pts',(-1.89136993975585,-1.,-0.43522566096358));
#22184=CARTESIAN_POINT('Ctrl Pts',(-1.89663648956549,-1.,-0.437995003948443));
#22185=CARTESIAN_POINT('Ctrl Pts',(-1.90180124389137,-1.,-0.44080783370416));
#22186=CARTESIAN_POINT('Ctrl Pts',(-1.90691756144906,-1.,-0.44367755684917));
#22187=CARTESIAN_POINT('Ctrl Pts',(-1.91203699981095,-1.,-0.446617343485651));
#22188=CARTESIAN_POINT('Ctrl Pts',(-1.91718342555717,-1.,-0.449632260106572));
#22189=CARTESIAN_POINT('Ctrl Pts',(-1.9223538064847,-1.,-0.452719478359356));
#22190=CARTESIAN_POINT('Ctrl Pts',(-1.92753067150461,-1.,-0.455872005174335));
#22191=CARTESIAN_POINT('Ctrl Pts',(-1.93269066517936,-1.,-0.459081234547931));
#22192=CARTESIAN_POINT('Ctrl Pts',(-1.93781486640834,-1.,-0.462340031009087));
#22193=CARTESIAN_POINT('Ctrl Pts',(-1.94289794196205,-1.,-0.465645462026064));
#22194=CARTESIAN_POINT('Ctrl Pts',(-1.94794381136524,-1.,-0.468997482913158));
#22195=CARTESIAN_POINT('Ctrl Pts',(-1.95296148278136,-1.,-0.472397672264079));
#22196=CARTESIAN_POINT('Ctrl Pts',(-1.95796111148175,-1.,-0.475848034683171));
#22197=CARTESIAN_POINT('Ctrl Pts',(-1.96294933055938,-1.,-0.479349583074846));
#22198=CARTESIAN_POINT('Ctrl Pts',(-1.96792703422358,-1.,-0.482901662120686));
#22199=CARTESIAN_POINT('Ctrl Pts',(-1.97289186263272,-1.,-0.486502692907661));
#22200=CARTESIAN_POINT('Ctrl Pts',(-1.97783973019229,-1.,-0.490150627860955));
#22201=CARTESIAN_POINT('Ctrl Pts',(-1.9827665876182,-1.,-0.493843476541492));
#22202=CARTESIAN_POINT('Ctrl Pts',(-1.98767044752929,-1.,-0.497579909545564));
#22203=CARTESIAN_POINT('Ctrl Pts',(-1.9925514912615,-1.,-0.501359287727129));
#22204=CARTESIAN_POINT('Ctrl Pts',(-1.99741107463567,-1.,-0.505181361323011));
#22205=CARTESIAN_POINT('Ctrl Pts',(-2.00225107134733,-1.,-0.509046069886152));
#22206=CARTESIAN_POINT('Ctrl Pts',(-2.00707309946955,-1.,-0.512953306961813));
#22207=CARTESIAN_POINT('Ctrl Pts',(-2.01187773939257,-1.,-0.516902681728733));
#22208=CARTESIAN_POINT('Ctrl Pts',(-2.01666477917305,-1.,-0.520893590399428));
#22209=CARTESIAN_POINT('Ctrl Pts',(-2.02143356304712,-1.,-0.524925318333518));
#22210=CARTESIAN_POINT('Ctrl Pts',(-2.02618329083289,-1.,-0.52899712724191));
#22211=CARTESIAN_POINT('Ctrl Pts',(-2.03091336214401,-1.,-0.533108355132905));
#22212=CARTESIAN_POINT('Ctrl Pts',(-2.03562362953993,-1.,-0.537258489833134));
#22213=CARTESIAN_POINT('Ctrl Pts',(-2.0403142269048,-1.,-0.54144712061552));
#22214=CARTESIAN_POINT('Ctrl Pts',(-2.0449854471456,-1.,-0.545673903817348));
#22215=CARTESIAN_POINT('Ctrl Pts',(-2.04963761077974,-1.,-0.549938525150342));
#22216=CARTESIAN_POINT('Ctrl Pts',(-2.05427091604482,-1.,-0.554240657464109));
#22217=CARTESIAN_POINT('Ctrl Pts',(-2.05888537756571,-1.,-0.558579940185467));
#22218=CARTESIAN_POINT('Ctrl Pts',(-2.06348090160697,-1.,-0.562955993082574));
#22219=CARTESIAN_POINT('Ctrl Pts',(-2.06805732997383,-1.,-0.567368421181229));
#22220=CARTESIAN_POINT('Ctrl Pts',(-2.07261449292757,-1.,-0.571816823242411));
#22221=CARTESIAN_POINT('Ctrl Pts',(-2.07715226767361,-1.,-0.576300797416274));
#22222=CARTESIAN_POINT('Ctrl Pts',(-2.08167059018138,-1.,-0.580819952107257));
#22223=CARTESIAN_POINT('Ctrl Pts',(-2.086169437277,-1.,-0.585373918990895));
#22224=CARTESIAN_POINT('Ctrl Pts',(-2.09064881812053,-1.,-0.589962365403189));
#22225=CARTESIAN_POINT('Ctrl Pts',(-2.09510876220501,-1.,-0.594585006052823));
#22226=CARTESIAN_POINT('Ctrl Pts',(-2.09954930865331,-1.,-0.599241616422144));
#22227=CARTESIAN_POINT('Ctrl Pts',(-2.10397049887709,-1.,-0.603932030738212));
#22228=CARTESIAN_POINT('Ctrl Pts',(-2.10749199615859,-1.,-0.607711315456826));
#22229=CARTESIAN_POINT('Ctrl Pts',(-2.11012443807661,-1.,-0.610560911691113));
#22230=CARTESIAN_POINT('Ctrl Pts',(-2.11187554260142,-1.,-0.61246736556225));
#22231=CARTESIAN_POINT('Ctrl Pts',(-2.11275013067528,-1.,-0.61342227326009));
#22232=CARTESIAN_POINT('',(-2.0698113262342,-1.,-0.745574324794401));
#22233=CARTESIAN_POINT('',(-2.11275013067528,-1.,-0.61342227326009));
#22234=CARTESIAN_POINT('',(-1.60662857109684,-1.,-0.693717979106306));
#22235=CARTESIAN_POINT('Ctrl Pts',(-2.0698113262342,-1.,-0.745574324794401));
#22236=CARTESIAN_POINT('Ctrl Pts',(-2.06854248895575,-1.,-0.74583279137781));
#22237=CARTESIAN_POINT('Ctrl Pts',(-2.06600523016401,-1.,-0.746345871542695));
#22238=CARTESIAN_POINT('Ctrl Pts',(-2.06220058927162,-1.,-0.747103932785504));
#22239=CARTESIAN_POINT('Ctrl Pts',(-2.05713023030263,-1.,-0.748091554181101));
#22240=CARTESIAN_POINT('Ctrl Pts',(-2.05079645591606,-1.,-0.749287468663053));
#22241=CARTESIAN_POINT('Ctrl Pts',(-2.04446689147754,-1.,-0.750444657874758));
#22242=CARTESIAN_POINT('Ctrl Pts',(-2.03814160092173,-1.,-0.751562963361383));
#22243=CARTESIAN_POINT('Ctrl Pts',(-2.03182068456467,-1.,-0.752642180488104));
#22244=CARTESIAN_POINT('Ctrl Pts',(-2.02550428623587,-1.,-0.753682061113765));
#22245=CARTESIAN_POINT('Ctrl Pts',(-2.01919259406003,-1.,-0.75468233072352));
#22246=CARTESIAN_POINT('Ctrl Pts',(-2.01288584328149,-1.,-0.7556427049581));
#22247=CARTESIAN_POINT('Ctrl Pts',(-2.00658431587682,-1.,-0.756562904646496));
#22248=CARTESIAN_POINT('Ctrl Pts',(-2.00028834739072,-1.,-0.757442676862341));
#22249=CARTESIAN_POINT('Ctrl Pts',(-1.9939983109871,-1.,-0.758281796766377));
#22250=CARTESIAN_POINT('Ctrl Pts',(-1.98771456680806,-1.,-0.759080037802242));
#22251=CARTESIAN_POINT('Ctrl Pts',(-1.98143741418156,-1.,-0.759837147452135));
#22252=CARTESIAN_POINT('Ctrl Pts',(-1.97516705321521,-1.,-0.760552825409855));
#22253=CARTESIAN_POINT('Ctrl Pts',(-1.96890351582545,-1.,-0.761226690483986));
#22254=CARTESIAN_POINT('Ctrl Pts',(-1.96264672744229,-1.,-0.761858300014575));
#22255=CARTESIAN_POINT('Ctrl Pts',(-1.95639665309893,-1.,-0.762447203806263));
#22256=CARTESIAN_POINT('Ctrl Pts',(-1.95015342590025,-1.,-0.762992990878774));
#22257=CARTESIAN_POINT('Ctrl Pts',(-1.94391746617626,-1.,-0.76349533353858));
#22258=CARTESIAN_POINT('Ctrl Pts',(-1.93768964875867,-1.,-0.763954049121393));
#22259=CARTESIAN_POINT('Ctrl Pts',(-1.93147105496367,-1.,-0.764369010673889));
#22260=CARTESIAN_POINT('Ctrl Pts',(-1.92526263537041,-1.,-0.764740025488189));
#22261=CARTESIAN_POINT('Ctrl Pts',(-1.91906491634197,-1.,-0.765066729667095));
#22262=CARTESIAN_POINT('Ctrl Pts',(-1.91287765805174,-1.,-0.765348465884739));
#22263=CARTESIAN_POINT('Ctrl Pts',(-1.90669961402362,-1.,-0.765584196937936));
#22264=CARTESIAN_POINT('Ctrl Pts',(-1.90052930393599,-1.,-0.765772772593395));
#22265=CARTESIAN_POINT('Ctrl Pts',(-1.89436577771389,-1.,-0.765913193856979));
#22266=CARTESIAN_POINT('Ctrl Pts',(-1.88820926433409,-1.,-0.76600483706209));
#22267=CARTESIAN_POINT('Ctrl Pts',(-1.88206215302561,-1.,-0.766047794851868));
#22268=CARTESIAN_POINT('Ctrl Pts',(-1.87592888967886,-1.,-0.766042837036759));
#22269=CARTESIAN_POINT('Ctrl Pts',(-1.86981398314345,-1.,-0.765990708546111));
#22270=CARTESIAN_POINT('Ctrl Pts',(-1.86372027063314,-1.,-0.765891519092557));
#22271=CARTESIAN_POINT('Ctrl Pts',(-1.85764741390391,-1.,-0.765744212909305));
#22272=CARTESIAN_POINT('Ctrl Pts',(-1.85158945130054,-1.,-0.765545710619023));
#22273=CARTESIAN_POINT('Ctrl Pts',(-1.8455369887591,-1.,-0.765291664861971));
#22274=CARTESIAN_POINT('Ctrl Pts',(-1.83948181064823,-1.,-0.764978057881687));
#22275=CARTESIAN_POINT('Ctrl Pts',(-1.8334207722714,-1.,-0.764602549687845));
#22276=CARTESIAN_POINT('Ctrl Pts',(-1.8273599120008,-1.,-0.764165902606055));
#22277=CARTESIAN_POINT('Ctrl Pts',(-1.82131873145297,-1.,-0.763673465462854));
#22278=CARTESIAN_POINT('Ctrl Pts',(-1.81532118405566,-1.,-0.763132003836783));
#22279=CARTESIAN_POINT('Ctrl Pts',(-1.80938551463989,-1.,-0.762546129464036));
#22280=CARTESIAN_POINT('Ctrl Pts',(-1.80351583877334,-1.,-0.761915336443515));
#22281=CARTESIAN_POINT('Ctrl Pts',(-1.79768986997735,-1.,-0.761229695230359));
#22282=CARTESIAN_POINT('Ctrl Pts',(-1.79185815610802,-1.,-0.760469555880425));
#22283=CARTESIAN_POINT('Ctrl Pts',(-1.78596964884526,-1.,-0.759614401109868));
#22284=CARTESIAN_POINT('Ctrl Pts',(-1.77999411220912,-1.,-0.75865062667738));
#22285=CARTESIAN_POINT('Ctrl Pts',(-1.77394167108342,-1.,-0.757578264077238));
#22286=CARTESIAN_POINT('Ctrl Pts',(-1.76789396003141,-1.,-0.756421896028403));
#22287=CARTESIAN_POINT('Ctrl Pts',(-1.7619781724032,-1.,-0.755220979975262));
#22288=CARTESIAN_POINT('Ctrl Pts',(-1.75631083600175,-1.,-0.75400925402848));
#22289=CARTESIAN_POINT('Ctrl Pts',(-1.75095139468809,-1.,-0.752797683531377));
#22290=CARTESIAN_POINT('Ctrl Pts',(-1.74585086852298,-1.,-0.751555614163629));
#22291=CARTESIAN_POINT('Ctrl Pts',(-1.74080458266705,-1.,-0.75019343597954));
#22292=CARTESIAN_POINT('Ctrl Pts',(-1.73550351679848,-1.,-0.748582462954854));
#22293=CARTESIAN_POINT('Ctrl Pts',(-1.72958533647399,-1.,-0.746574710096436));
#22294=CARTESIAN_POINT('Ctrl Pts',(-1.7226822991693,-1.,-0.744021445433764));
#22295=CARTESIAN_POINT('Ctrl Pts',(-1.71447789751927,-1.,-0.740795162032087));
#22296=CARTESIAN_POINT('Ctrl Pts',(-1.70473309006121,-1.,-0.736799665724771));
#22297=CARTESIAN_POINT('Ctrl Pts',(-1.69326921975743,-1.,-0.731963238697195));
#22298=CARTESIAN_POINT('Ctrl Pts',(-1.67996158455503,-1.,-0.726235967997433));
#22299=CARTESIAN_POINT('Ctrl Pts',(-1.6647288055568,-1.,-0.719585433804282));
#22300=CARTESIAN_POINT('Ctrl Pts',(-1.64752408832016,-1.,-0.711993139355394));
#22301=CARTESIAN_POINT('Ctrl Pts',(-1.63216541664676,-1.,-0.705159151988319));
#22302=CARTESIAN_POINT('Ctrl Pts',(-1.61974673472612,-1.,-0.699605146405088));
#22303=CARTESIAN_POINT('Ctrl Pts',(-1.61106790958151,-1.,-0.695712097881194));
#22304=CARTESIAN_POINT('Ctrl Pts',(-1.60662857109684,-1.,-0.693717979106306));
#22305=CARTESIAN_POINT('',(-1.5055822144029,-1.,-0.892032620296855));
#22306=CARTESIAN_POINT('Origin',(0.,-1.,0.));
#22307=CARTESIAN_POINT('',(-1.81978687191668,-1.,-1.23627494547115));
#22308=CARTESIAN_POINT('Ctrl Pts',(-1.5055822144029,-1.,-0.892032620296855));
#22309=CARTESIAN_POINT('Ctrl Pts',(-1.50980486806688,-1.,-0.894452006964543));
#22310=CARTESIAN_POINT('Ctrl Pts',(-1.51805569590094,-1.,-0.899185047483511));
#22311=CARTESIAN_POINT('Ctrl Pts',(-1.52984849887993,-1.,-0.905967409625651));
#22312=CARTESIAN_POINT('Ctrl Pts',(-1.54440491149498,-1.,-0.914375919026456));
#22313=CARTESIAN_POINT('Ctrl Pts',(-1.56065988578893,-1.,-0.923832188944341));
#22314=CARTESIAN_POINT('Ctrl Pts',(-1.57499388382243,-1.,-0.932246680108685));
#22315=CARTESIAN_POINT('Ctrl Pts',(-1.58744937487176,-1.,-0.939646377893399));
#22316=CARTESIAN_POINT('Ctrl Pts',(-1.59810042043673,-1.,-0.946078063315257));
#22317=CARTESIAN_POINT('Ctrl Pts',(-1.60706069896936,-1.,-0.951613284356035));
#22318=CARTESIAN_POINT('Ctrl Pts',(-1.61449324337085,-1.,-0.956354422920671));
#22319=CARTESIAN_POINT('Ctrl Pts',(-1.62061638140221,-1.,-0.960438326101729));
#22320=CARTESIAN_POINT('Ctrl Pts',(-1.62571930670187,-1.,-0.964046107040536));
#22321=CARTESIAN_POINT('Ctrl Pts',(-1.63013849959461,-1.,-0.967387853230345));
#22322=CARTESIAN_POINT('Ctrl Pts',(-1.63420665729798,-1.,-0.970669715997509));
#22323=CARTESIAN_POINT('Ctrl Pts',(-1.63820952658144,-1.,-0.974066058287418));
#22324=CARTESIAN_POINT('Ctrl Pts',(-1.64233990826687,-1.,-0.977689794119416));
#22325=CARTESIAN_POINT('Ctrl Pts',(-1.64665139190656,-1.,-0.981562530939489));
#22326=CARTESIAN_POINT('Ctrl Pts',(-1.65110016612638,-1.,-0.985642622920821));
#22327=CARTESIAN_POINT('Ctrl Pts',(-1.65559044289699,-1.,-0.989855627854165));
#22328=CARTESIAN_POINT('Ctrl Pts',(-1.66001553809947,-1.,-0.994121836661306));
#22329=CARTESIAN_POINT('Ctrl Pts',(-1.66430758030376,-1.,-0.998389654952758));
#22330=CARTESIAN_POINT('Ctrl Pts',(-1.66846059277303,-1.,-1.00265091003727));
#22331=CARTESIAN_POINT('Ctrl Pts',(-1.67250335383293,-1.,-1.00692206696414));
#22332=CARTESIAN_POINT('Ctrl Pts',(-1.67648246776464,-1.,-1.01123236493511));
#22333=CARTESIAN_POINT('Ctrl Pts',(-1.68044289894798,-1.,-1.01561026162773));
#22334=CARTESIAN_POINT('Ctrl Pts',(-1.68440578021706,-1.,-1.02006795074201));
#22335=CARTESIAN_POINT('Ctrl Pts',(-1.68836910178447,-1.,-1.02460180535255));
#22336=CARTESIAN_POINT('Ctrl Pts',(-1.69231840863458,-1.,-1.02919977579147));
#22337=CARTESIAN_POINT('Ctrl Pts',(-1.69623414782771,-1.,-1.03384646003588));
#22338=CARTESIAN_POINT('Ctrl Pts',(-1.70010052930962,-1.,-1.03852922490789));
#22339=CARTESIAN_POINT('Ctrl Pts',(-1.70391338707982,-1.,-1.04324363334554));
#22340=CARTESIAN_POINT('Ctrl Pts',(-1.70767646263649,-1.,-1.04799085404995));
#22341=CARTESIAN_POINT('Ctrl Pts',(-1.71139783543989,-1.,-1.05277517202855));
#22342=CARTESIAN_POINT('Ctrl Pts',(-1.7150865442702,-1.,-1.05760163192479));
#22343=CARTESIAN_POINT('Ctrl Pts',(-1.71874858456904,-1.,-1.06247324680647));
#22344=CARTESIAN_POINT('Ctrl Pts',(-1.72238500928453,-1.,-1.06738966975462));
#22345=CARTESIAN_POINT('Ctrl Pts',(-1.72599406198488,-1.,-1.07234866990252));
#22346=CARTESIAN_POINT('Ctrl Pts',(-1.72957248977424,-1.,-1.0773470373727));
#22347=CARTESIAN_POINT('Ctrl Pts',(-1.73311705663407,-1.,-1.08238162784749));
#22348=CARTESIAN_POINT('Ctrl Pts',(-1.73662628326091,-1.,-1.08745056285427));
#22349=CARTESIAN_POINT('Ctrl Pts',(-1.74010053962247,-1.,-1.09255329056493));
#22350=CARTESIAN_POINT('Ctrl Pts',(-1.74354119236208,-1.,-1.09768999241225));
#22351=CARTESIAN_POINT('Ctrl Pts',(-1.74695004214923,-1.,-1.10286118991143));
#22352=CARTESIAN_POINT('Ctrl Pts',(-1.7503286607592,-1.,-1.10806728183007));
#22353=CARTESIAN_POINT('Ctrl Pts',(-1.7536777209463,-1.,-1.11330807582551));
#22354=CARTESIAN_POINT('Ctrl Pts',(-1.75699720772105,-1.,-1.11858293216763));
#22355=CARTESIAN_POINT('Ctrl Pts',(-1.76028671825096,-1.,-1.12389096855086));
#22356=CARTESIAN_POINT('Ctrl Pts',(-1.7635457196617,-1.,-1.12923123555075));
#22357=CARTESIAN_POINT('Ctrl Pts',(-1.76677384551862,-1.,-1.1346029180462));
#22358=CARTESIAN_POINT('Ctrl Pts',(-1.76997111386769,-1.,-1.14000548336975));
#22359=CARTESIAN_POINT('Ctrl Pts',(-1.77313777896194,-1.,-1.1454385822692));
#22360=CARTESIAN_POINT('Ctrl Pts',(-1.7762742255701,-1.,-1.15090197841515));
#22361=CARTESIAN_POINT('Ctrl Pts',(-1.77938085564275,-1.,-1.15639547194698));
#22362=CARTESIAN_POINT('Ctrl Pts',(-1.78245795881009,-1.,-1.16191881298499));
#22363=CARTESIAN_POINT('Ctrl Pts',(-1.78550566040443,-1.,-1.16747166312303));
#22364=CARTESIAN_POINT('Ctrl Pts',(-1.78852398877616,-1.,-1.17305363177328));
#22365=CARTESIAN_POINT('Ctrl Pts',(-1.79151291552689,-1.,-1.17866429440809));
#22366=CARTESIAN_POINT('Ctrl Pts',(-1.79447240321515,-1.,-1.18430321697432));
#22367=CARTESIAN_POINT('Ctrl Pts',(-1.79740245923478,-1.,-1.18996997934445));
#22368=CARTESIAN_POINT('Ctrl Pts',(-1.80030314369879,-1.,-1.19566418930242));
#22369=CARTESIAN_POINT('Ctrl Pts',(-1.80317454838603,-1.,-1.20138548938974));
#22370=CARTESIAN_POINT('Ctrl Pts',(-1.80601678480707,-1.,-1.20713356605475));
#22371=CARTESIAN_POINT('Ctrl Pts',(-1.80882996917129,-1.,-1.21290815708314));
#22372=CARTESIAN_POINT('Ctrl Pts',(-1.81161420806656,-1.,-1.21870906103557));
#22373=CARTESIAN_POINT('Ctrl Pts',(-1.81436959210434,-1.,-1.2245361330495));
#22374=CARTESIAN_POINT('Ctrl Pts',(-1.8165508718364,-1.,-1.2292186489137));
#22375=CARTESIAN_POINT('Ctrl Pts',(-1.81817389921279,-1.,-1.2327422452705));
#22376=CARTESIAN_POINT('Ctrl Pts',(-1.81925017193666,-1.,-1.23509651170476));
#22377=CARTESIAN_POINT('Ctrl Pts',(-1.81978687191668,-1.,-1.23627494547115));
#22378=CARTESIAN_POINT('',(-1.73811241238545,-1.,-1.34869019493419));
#22379=CARTESIAN_POINT('',(-1.81978687191668,-1.,-1.23627494547115));
#22380=CARTESIAN_POINT('',(-1.31362392696032,-1.,-1.15624053661742));
#22381=CARTESIAN_POINT('Ctrl Pts',(-1.73811241238545,-1.,-1.34869019493419));
#22382=CARTESIAN_POINT('Ctrl Pts',(-1.73682580585691,-1.,-1.34854391898045));
#22383=CARTESIAN_POINT('Ctrl Pts',(-1.73425417885907,-1.,-1.34824783112887));
#22384=CARTESIAN_POINT('Ctrl Pts',(-1.7304014965394,-1.,-1.34779309152035));
#22385=CARTESIAN_POINT('Ctrl Pts',(-1.72527410680674,-1.,-1.34716554819527));
#22386=CARTESIAN_POINT('Ctrl Pts',(-1.7188807715049,-1.,-1.34634568653227));
#22387=CARTESIAN_POINT('Ctrl Pts',(-1.71250340686822,-1.,-1.34549029589416));
#22388=CARTESIAN_POINT('Ctrl Pts',(-1.70614212266738,-1.,-1.34459924533831));
#22389=CARTESIAN_POINT('Ctrl Pts',(-1.69979707754427,-1.,-1.34367237124483));
#22390=CARTESIAN_POINT('Ctrl Pts',(-1.6934684849687,-1.,-1.34270948206319));
#22391=CARTESIAN_POINT('Ctrl Pts',(-1.68715660868764,-1.,-1.341710374848));
#22392=CARTESIAN_POINT('Ctrl Pts',(-1.68086176030362,-1.,-1.34067485185203));
#22393=CARTESIAN_POINT('Ctrl Pts',(-1.67458429426086,-1.,-1.3396027347034));
#22394=CARTESIAN_POINT('Ctrl Pts',(-1.66832460783989,-1.,-1.33849388654388));
#22395=CARTESIAN_POINT('Ctrl Pts',(-1.66208312541983,-1.,-1.33734820885262));
#22396=CARTESIAN_POINT('Ctrl Pts',(-1.65586025952593,-1.,-1.33616559745172));
#22397=CARTESIAN_POINT('Ctrl Pts',(-1.6496563728683,-1.,-1.33494590467993));
#22398=CARTESIAN_POINT('Ctrl Pts',(-1.6434717485603,-1.,-1.33368890676572));
#22399=CARTESIAN_POINT('Ctrl Pts',(-1.63730653475089,-1.,-1.33239425103724));
#22400=CARTESIAN_POINT('Ctrl Pts',(-1.63116079730923,-1.,-1.33106149345645));
#22401=CARTESIAN_POINT('Ctrl Pts',(-1.62503464209797,-1.,-1.3296901950568));
#22402=CARTESIAN_POINT('Ctrl Pts',(-1.61892832270724,-1.,-1.32828000610449));
#22403=CARTESIAN_POINT('Ctrl Pts',(-1.6128423401575,-1.,-1.32683074483356));
#22404=CARTESIAN_POINT('Ctrl Pts',(-1.60677758290954,-1.,-1.32534250785782));
#22405=CARTESIAN_POINT('Ctrl Pts',(-1.60073511858687,-1.,-1.32381550858256));
#22406=CARTESIAN_POINT('Ctrl Pts',(-1.59471591079403,-1.,-1.32224985747682));
#22407=CARTESIAN_POINT('Ctrl Pts',(-1.58872057258245,-1.,-1.32064537110892));
#22408=CARTESIAN_POINT('Ctrl Pts',(-1.58274907898834,-1.,-1.31900135021432));
#22409=CARTESIAN_POINT('Ctrl Pts',(-1.5768005650559,-1.,-1.31731642317187));
#22410=CARTESIAN_POINT('Ctrl Pts',(-1.57087397835723,-1.,-1.31558903860016));
#22411=CARTESIAN_POINT('Ctrl Pts',(-1.56496872402353,-1.,-1.31381795281002));
#22412=CARTESIAN_POINT('Ctrl Pts',(-1.55908521254821,-1.,-1.31200264341696));
#22413=CARTESIAN_POINT('Ctrl Pts',(-1.55322568759481,-1.,-1.31014393684222));
#22414=CARTESIAN_POINT('Ctrl Pts',(-1.54739413957185,-1.,-1.30824393907473));
#22415=CARTESIAN_POINT('Ctrl Pts',(-1.54159462645432,-1.,-1.30630475189556));
#22416=CARTESIAN_POINT('Ctrl Pts',(-1.53582981268977,-1.,-1.30432735639489));
#22417=CARTESIAN_POINT('Ctrl Pts',(-1.53009970283891,-1.,-1.30231064395568));
#22418=CARTESIAN_POINT('Ctrl Pts',(-1.52439957861062,-1.,-1.30024984366328));
#22419=CARTESIAN_POINT('Ctrl Pts',(-1.51872184912724,-1.,-1.29813791800747));
#22420=CARTESIAN_POINT('Ctrl Pts',(-1.51305994241402,-1.,-1.29596850710509));
#22421=CARTESIAN_POINT('Ctrl Pts',(-1.50741159078365,-1.,-1.29373841372842));
#22422=CARTESIAN_POINT('Ctrl Pts',(-1.50178230149776,-1.,-1.29145022885181));
#22423=CARTESIAN_POINT('Ctrl Pts',(-1.49618896881754,-1.,-1.28911506584254));
#22424=CARTESIAN_POINT('Ctrl Pts',(-1.4906522831278,-1.,-1.2867467611644));
#22425=CARTESIAN_POINT('Ctrl Pts',(-1.4851881711891,-1.,-1.28435533880201));
#22426=CARTESIAN_POINT('Ctrl Pts',(-1.47980070347095,-1.,-1.28194158939517));
#22427=CARTESIAN_POINT('Ctrl Pts',(-1.4744717526707,-1.,-1.2794891824849));
#22428=CARTESIAN_POINT('Ctrl Pts',(-1.46916035917133,-1.,-1.27696414831089));
#22429=CARTESIAN_POINT('Ctrl Pts',(-1.46382431332476,-1.,-1.27433119897822));
#22430=CARTESIAN_POINT('Ctrl Pts',(-1.45843906294697,-1.,-1.27156805265289));
#22431=CARTESIAN_POINT('Ctrl Pts',(-1.45301422764247,-1.,-1.2686778680489));
#22432=CARTESIAN_POINT('Ctrl Pts',(-1.44761985001662,-1.,-1.26570925118868));
#22433=CARTESIAN_POINT('Ctrl Pts',(-1.44236470511303,-1.,-1.26273903323859));
#22434=CARTESIAN_POINT('Ctrl Pts',(-1.43734919180848,-1.,-1.25983531012005));
#22435=CARTESIAN_POINT('Ctrl Pts',(-1.43262645609691,-1.,-1.25702687965755));
#22436=CARTESIAN_POINT('Ctrl Pts',(-1.42815938799387,-1.,-1.25426945222639));
#22437=CARTESIAN_POINT('Ctrl Pts',(-1.42378102115575,-1.,-1.2514145557001));
#22438=CARTESIAN_POINT('Ctrl Pts',(-1.41923722596025,-1.,-1.24824430986571));
#22439=CARTESIAN_POINT('Ctrl Pts',(-1.41422913175179,-1.,-1.24450600513056));
#22440=CARTESIAN_POINT('Ctrl Pts',(-1.40845295531283,-1.,-1.23994455029534));
#22441=CARTESIAN_POINT('Ctrl Pts',(-1.40164708206106,-1.,-1.23434087290423));
#22442=CARTESIAN_POINT('Ctrl Pts',(-1.39361389568796,-1.,-1.22752961899387));
#22443=CARTESIAN_POINT('Ctrl Pts',(-1.38420564527715,-1.,-1.21938737280852));
#22444=CARTESIAN_POINT('Ctrl Pts',(-1.37331915607905,-1.,-1.20982812925645));
#22445=CARTESIAN_POINT('Ctrl Pts',(-1.36088705043885,-1.,-1.1987959077932));
#22446=CARTESIAN_POINT('Ctrl Pts',(-1.34687054001093,-1.,-1.18625865667441));
#22447=CARTESIAN_POINT('Ctrl Pts',(-1.33437539347008,-1.,-1.17501305789857));
#22448=CARTESIAN_POINT('Ctrl Pts',(-1.32428080721772,-1.,-1.16589330093588));
#22449=CARTESIAN_POINT('Ctrl Pts',(-1.31722977216397,-1.,-1.15950888730809));
#22450=CARTESIAN_POINT('Ctrl Pts',(-1.31362392696032,-1.,-1.15624053661742));
#22451=CARTESIAN_POINT('',(-1.15624053661742,-1.,-1.31362392696033));
#22452=CARTESIAN_POINT('Origin',(0.,-1.,0.));
#22453=CARTESIAN_POINT('',(-1.34869019493419,-1.,-1.73811241238545));
#22454=CARTESIAN_POINT('Ctrl Pts',(-1.15624053661742,-1.,-1.31362392696033));
#22455=CARTESIAN_POINT('Ctrl Pts',(-1.15950888730433,-1.,-1.3172297721596));
#22456=CARTESIAN_POINT('Ctrl Pts',(-1.16589330092532,-1.,-1.32428080720544));
#22457=CARTESIAN_POINT('Ctrl Pts',(-1.17501305787994,-1.,-1.33437539344842));
#22458=CARTESIAN_POINT('Ctrl Pts',(-1.18625865664915,-1.,-1.34687053998157));
#22459=CARTESIAN_POINT('Ctrl Pts',(-1.1987959077656,-1.,-1.36088705040677));
#22460=CARTESIAN_POINT('Ctrl Pts',(-1.20982812923113,-1.,-1.37331915604962));
#22461=CARTESIAN_POINT('Ctrl Pts',(-1.21938737278853,-1.,-1.38420564525391));
#22462=CARTESIAN_POINT('Ctrl Pts',(-1.22752961898063,-1.,-1.39361389567257));
#22463=CARTESIAN_POINT('Ctrl Pts',(-1.23434087289768,-1.,-1.40164708205345));
#22464=CARTESIAN_POINT('Ctrl Pts',(-1.23994455029421,-1.,-1.40845295531151));
#22465=CARTESIAN_POINT('Ctrl Pts',(-1.24450600513278,-1.,-1.41422913175437));
#22466=CARTESIAN_POINT('Ctrl Pts',(-1.24824430986911,-1.,-1.41923722596421));
#22467=CARTESIAN_POINT('Ctrl Pts',(-1.25141455570299,-1.,-1.42378102115911));
#22468=CARTESIAN_POINT('Ctrl Pts',(-1.25426945222783,-1.,-1.42815938799555));
#22469=CARTESIAN_POINT('Ctrl Pts',(-1.25702687965744,-1.,-1.43262645609679));
#22470=CARTESIAN_POINT('Ctrl Pts',(-1.25983531011894,-1.,-1.43734919180719));
#22471=CARTESIAN_POINT('Ctrl Pts',(-1.26273903323723,-1.,-1.44236470511145));
#22472=CARTESIAN_POINT('Ctrl Pts',(-1.26570925118767,-1.,-1.44761985001544));
#22473=CARTESIAN_POINT('Ctrl Pts',(-1.26867786804854,-1.,-1.45301422764205));
#22474=CARTESIAN_POINT('Ctrl Pts',(-1.27156805265312,-1.,-1.45843906294725));
#22475=CARTESIAN_POINT('Ctrl Pts',(-1.27433119897877,-1.,-1.4638243133254));
#22476=CARTESIAN_POINT('Ctrl Pts',(-1.27696414831144,-1.,-1.46916035917197));
#22477=CARTESIAN_POINT('Ctrl Pts',(-1.27948918248524,-1.,-1.4744717526711));
#22478=CARTESIAN_POINT('Ctrl Pts',(-1.28194158939522,-1.,-1.47980070347102));
#22479=CARTESIAN_POINT('Ctrl Pts',(-1.28435533880184,-1.,-1.48518817118891));
#22480=CARTESIAN_POINT('Ctrl Pts',(-1.28674676116415,-1.,-1.4906522831275));
#22481=CARTESIAN_POINT('Ctrl Pts',(-1.28911506584232,-1.,-1.49618896881729));
#22482=CARTESIAN_POINT('Ctrl Pts',(-1.29145022885171,-1.,-1.50178230149764));
#22483=CARTESIAN_POINT('Ctrl Pts',(-1.29373841372843,-1.,-1.50741159078367));
#22484=CARTESIAN_POINT('Ctrl Pts',(-1.29596850710518,-1.,-1.51305994241412));
#22485=CARTESIAN_POINT('Ctrl Pts',(-1.29813791800757,-1.,-1.51872184912735));
#22486=CARTESIAN_POINT('Ctrl Pts',(-1.30024984366334,-1.,-1.5243995786107));
#22487=CARTESIAN_POINT('Ctrl Pts',(-1.3023106439557,-1.,-1.53009970283893));
#22488=CARTESIAN_POINT('Ctrl Pts',(-1.30432735639487,-1.,-1.53582981268976));
#22489=CARTESIAN_POINT('Ctrl Pts',(-1.30630475189553,-1.,-1.54159462645428));
#22490=CARTESIAN_POINT('Ctrl Pts',(-1.30824393907471,-1.,-1.54739413957183));
#22491=CARTESIAN_POINT('Ctrl Pts',(-1.31014393684221,-1.,-1.55322568759481));
#22492=CARTESIAN_POINT('Ctrl Pts',(-1.31200264341696,-1.,-1.55908521254822));
#22493=CARTESIAN_POINT('Ctrl Pts',(-1.31381795281002,-1.,-1.56496872402352));
#22494=CARTESIAN_POINT('Ctrl Pts',(-1.31558903860015,-1.,-1.57087397835721));
#22495=CARTESIAN_POINT('Ctrl Pts',(-1.31731642317183,-1.,-1.57680056505585));
#22496=CARTESIAN_POINT('Ctrl Pts',(-1.31900135021428,-1.,-1.58274907898829));
#22497=CARTESIAN_POINT('Ctrl Pts',(-1.32064537110891,-1.,-1.58872057258244));
#22498=CARTESIAN_POINT('Ctrl Pts',(-1.32224985747686,-1.,-1.59471591079408));
#22499=CARTESIAN_POINT('Ctrl Pts',(-1.32381550858266,-1.,-1.600735118587));
#22500=CARTESIAN_POINT('Ctrl Pts',(-1.32534250785794,-1.,-1.6067775829097));
#22501=CARTESIAN_POINT('Ctrl Pts',(-1.32683074483365,-1.,-1.61284234015762));
#22502=CARTESIAN_POINT('Ctrl Pts',(-1.32828000610448,-1.,-1.61892832270723));
#22503=CARTESIAN_POINT('Ctrl Pts',(-1.32969019505665,-1.,-1.62503464209777));
#22504=CARTESIAN_POINT('Ctrl Pts',(-1.33106149345618,-1.,-1.63116079730887));
#22505=CARTESIAN_POINT('Ctrl Pts',(-1.33239425103694,-1.,-1.6373065347505));
#22506=CARTESIAN_POINT('Ctrl Pts',(-1.33368890676554,-1.,-1.64347174856007));
#22507=CARTESIAN_POINT('Ctrl Pts',(-1.33494590468003,-1.,-1.64965637286843));
#22508=CARTESIAN_POINT('Ctrl Pts',(-1.33616559745217,-1.,-1.65586025952651));
#22509=CARTESIAN_POINT('Ctrl Pts',(-1.33734820885331,-1.,-1.66208312542073));
#22510=CARTESIAN_POINT('Ctrl Pts',(-1.33849388654458,-1.,-1.66832460784078));
#22511=CARTESIAN_POINT('Ctrl Pts',(-1.33960273470372,-1.,-1.67458429426126));
#22512=CARTESIAN_POINT('Ctrl Pts',(-1.3406748518516,-1.,-1.68086176030308));
#22513=CARTESIAN_POINT('Ctrl Pts',(-1.34171037484673,-1.,-1.68715660868602));
#22514=CARTESIAN_POINT('Ctrl Pts',(-1.34270948206139,-1.,-1.6934684849664));
#22515=CARTESIAN_POINT('Ctrl Pts',(-1.34367237124322,-1.,-1.69979707754221));
#22516=CARTESIAN_POINT('Ctrl Pts',(-1.34459924533783,-1.,-1.70614212266676));
#22517=CARTESIAN_POINT('Ctrl Pts',(-1.34549029589563,-1.,-1.71250340687011));
#22518=CARTESIAN_POINT('Ctrl Pts',(-1.34634568653586,-1.,-1.7188807715095));
#22519=CARTESIAN_POINT('Ctrl Pts',(-1.34716554820013,-1.,-1.72527410681298));
#22520=CARTESIAN_POINT('Ctrl Pts',(-1.3477930915247,-1.,-1.73040149654497));
#22521=CARTESIAN_POINT('Ctrl Pts',(-1.34824783113158,-1.,-1.73425417886255));
#22522=CARTESIAN_POINT('Ctrl Pts',(-1.34854391898145,-1.,-1.73682580585819));
#22523=CARTESIAN_POINT('Ctrl Pts',(-1.34869019493419,-1.,-1.73811241238545));
#22524=CARTESIAN_POINT('',(-1.23627494547115,-1.,-1.81978687191668));
#22525=CARTESIAN_POINT('',(-1.34869019493419,-1.,-1.73811241238545));
#22526=CARTESIAN_POINT('',(-0.892032620296855,-1.,-1.5055822144029));
#22527=CARTESIAN_POINT('Ctrl Pts',(-1.23627494547115,-1.,-1.81978687191668));
#22528=CARTESIAN_POINT('Ctrl Pts',(-1.23509651170384,-1.,-1.81925017193531));
#22529=CARTESIAN_POINT('Ctrl Pts',(-1.23274224526804,-1.,-1.81817389920914));
#22530=CARTESIAN_POINT('Ctrl Pts',(-1.22921864890975,-1.,-1.81655087183054));
#22531=CARTESIAN_POINT('Ctrl Pts',(-1.22453613304507,-1.,-1.81436959209778));
#22532=CARTESIAN_POINT('Ctrl Pts',(-1.2187090610323,-1.,-1.81161420806172));
#22533=CARTESIAN_POINT('Ctrl Pts',(-1.2129081570818,-1.,-1.80882996916931));
#22534=CARTESIAN_POINT('Ctrl Pts',(-1.20713356605519,-1.,-1.80601678480772));
#22535=CARTESIAN_POINT('Ctrl Pts',(-1.2013854893912,-1.,-1.8031745483882));
#22536=CARTESIAN_POINT('Ctrl Pts',(-1.19566418930405,-1.,-1.80030314370121));
#22537=CARTESIAN_POINT('Ctrl Pts',(-1.1899699793456,-1.,-1.79740245923649));
#22538=CARTESIAN_POINT('Ctrl Pts',(-1.18430321697471,-1.,-1.79447240321572));
#22539=CARTESIAN_POINT('Ctrl Pts',(-1.17866429440781,-1.,-1.79151291552646));
#22540=CARTESIAN_POINT('Ctrl Pts',(-1.17305363177265,-1.,-1.78852398877523));
#22541=CARTESIAN_POINT('Ctrl Pts',(-1.16747166312239,-1.,-1.78550566040349));
#22542=CARTESIAN_POINT('Ctrl Pts',(-1.16191881298458,-1.,-1.78245795880949));
#22543=CARTESIAN_POINT('Ctrl Pts',(-1.15639547194689,-1.,-1.77938085564261));
#22544=CARTESIAN_POINT('Ctrl Pts',(-1.15090197841531,-1.,-1.77627422557034));
#22545=CARTESIAN_POINT('Ctrl Pts',(-1.14543858226948,-1.,-1.77313777896234));
#22546=CARTESIAN_POINT('Ctrl Pts',(-1.14000548337,-1.,-1.76997111386806));
#22547=CARTESIAN_POINT('Ctrl Pts',(-1.13460291804635,-1.,-1.76677384551883));
#22548=CARTESIAN_POINT('Ctrl Pts',(-1.12923123555076,-1.,-1.76354571966171));
#22549=CARTESIAN_POINT('Ctrl Pts',(-1.12389096855078,-1.,-1.76028671825084));
#22550=CARTESIAN_POINT('Ctrl Pts',(-1.11858293216752,-1.,-1.75699720772089));
#22551=CARTESIAN_POINT('Ctrl Pts',(-1.11330807582542,-1.,-1.75367772094617));
#22552=CARTESIAN_POINT('Ctrl Pts',(-1.10806728183003,-1.,-1.75032866075914));
#22553=CARTESIAN_POINT('Ctrl Pts',(-1.10286118991144,-1.,-1.74695004214924));
#22554=CARTESIAN_POINT('Ctrl Pts',(-1.09768999241229,-1.,-1.74354119236212));
#22555=CARTESIAN_POINT('Ctrl Pts',(-1.09255329056496,-1.,-1.74010053962252));
#22556=CARTESIAN_POINT('Ctrl Pts',(-1.08745056285429,-1.,-1.73662628326093));
#22557=CARTESIAN_POINT('Ctrl Pts',(-1.08238162784749,-1.,-1.73311705663407));
#22558=CARTESIAN_POINT('Ctrl Pts',(-1.0773470373727,-1.,-1.72957248977424));
#22559=CARTESIAN_POINT('Ctrl Pts',(-1.07234866990252,-1.,-1.72599406198489));
#22560=CARTESIAN_POINT('Ctrl Pts',(-1.06738966975463,-1.,-1.72238500928456));
#22561=CARTESIAN_POINT('Ctrl Pts',(-1.0624732468065,-1.,-1.71874858456908));
#22562=CARTESIAN_POINT('Ctrl Pts',(-1.05760163192481,-1.,-1.71508654427022));
#22563=CARTESIAN_POINT('Ctrl Pts',(-1.05277517202854,-1.,-1.71139783543986));
#22564=CARTESIAN_POINT('Ctrl Pts',(-1.0479908540499,-1.,-1.70767646263641));
#22565=CARTESIAN_POINT('Ctrl Pts',(-1.04324363334546,-1.,-1.70391338707969));
#22566=CARTESIAN_POINT('Ctrl Pts',(-1.03852922490782,-1.,-1.70010052930951));
#22567=CARTESIAN_POINT('Ctrl Pts',(-1.03384646003587,-1.,-1.69623414782769));
#22568=CARTESIAN_POINT('Ctrl Pts',(-1.02919977579155,-1.,-1.69231840863471));
#22569=CARTESIAN_POINT('Ctrl Pts',(-1.02460180535272,-1.,-1.68836910178475));
#22570=CARTESIAN_POINT('Ctrl Pts',(-1.02006795074222,-1.,-1.68440578021739));
#22571=CARTESIAN_POINT('Ctrl Pts',(-1.01561026162787,-1.,-1.6804428989482));
#22572=CARTESIAN_POINT('Ctrl Pts',(-1.01123236493507,-1.,-1.67648246776457));
#22573=CARTESIAN_POINT('Ctrl Pts',(-1.00692206696387,-1.,-1.67250335383248));
#22574=CARTESIAN_POINT('Ctrl Pts',(-1.00265091003682,-1.,-1.66846059277231));
#22575=CARTESIAN_POINT('Ctrl Pts',(-0.998389654952317,-1.,-1.66430758030304));
#22576=CARTESIAN_POINT('Ctrl Pts',(-0.994121836661116,-1.,-1.66001553809916));
#22577=CARTESIAN_POINT('Ctrl Pts',(-0.98985562785445,-1.,-1.65559044289746));
#22578=CARTESIAN_POINT('Ctrl Pts',(-0.985642622921626,-1.,-1.6511001661277));
#22579=CARTESIAN_POINT('Ctrl Pts',(-0.981562530940574,-1.,-1.64665139190834));
#22580=CARTESIAN_POINT('Ctrl Pts',(-0.977689794120297,-1.,-1.64233990826831));
#22581=CARTESIAN_POINT('Ctrl Pts',(-0.974066058287501,-1.,-1.63820952658157));
#22582=CARTESIAN_POINT('Ctrl Pts',(-0.970669715996356,-1.,-1.63420665729609));
#22583=CARTESIAN_POINT('Ctrl Pts',(-0.967387853228041,-1.,-1.63013849959083));
#22584=CARTESIAN_POINT('Ctrl Pts',(-0.964046107037821,-1.,-1.6257193066974));
#22585=CARTESIAN_POINT('Ctrl Pts',(-0.960438326099958,-1.,-1.62061638139929));
#22586=CARTESIAN_POINT('Ctrl Pts',(-0.956354422921573,-1.,-1.61449324337233));
#22587=CARTESIAN_POINT('Ctrl Pts',(-0.951613284361248,-1.,-1.60706069897794));
#22588=CARTESIAN_POINT('Ctrl Pts',(-0.946078063325796,-1.,-1.59810042045408));
#22589=CARTESIAN_POINT('Ctrl Pts',(-0.939646377909319,-1.,-1.58744937489796));
#22590=CARTESIAN_POINT('Ctrl Pts',(-0.932246680128849,-1.,-1.57499388385561));
#22591=CARTESIAN_POINT('Ctrl Pts',(-0.923832188966322,-1.,-1.56065988582509));
#22592=CARTESIAN_POINT('Ctrl Pts',(-0.91437591904658,-1.,-1.54440491152808));
#22593=CARTESIAN_POINT('Ctrl Pts',(-0.905967409640499,-1.,-1.52984849890434));
#22594=CARTESIAN_POINT('Ctrl Pts',(-0.89918504749193,-1.,-1.51805569591479));
#22595=CARTESIAN_POINT('Ctrl Pts',(-0.894452006967538,-1.,-1.50980486807181));
#22596=CARTESIAN_POINT('Ctrl Pts',(-0.892032620296855,-1.,-1.5055822144029));
#22597=CARTESIAN_POINT('',(-0.693717979106305,-1.,-1.60662857109684));
#22598=CARTESIAN_POINT('Origin',(0.,-1.,0.));
#22599=CARTESIAN_POINT('',(-0.745574324794401,-1.,-2.0698113262342));
#22600=CARTESIAN_POINT('Ctrl Pts',(-0.693717979106305,-1.,-1.60662857109684));
#22601=CARTESIAN_POINT('Ctrl Pts',(-0.69571209787897,-1.,-1.61106790957619));
#22602=CARTESIAN_POINT('Ctrl Pts',(-0.699605146398837,-1.,-1.61974673471117));
#22603=CARTESIAN_POINT('Ctrl Pts',(-0.705159151977294,-1.,-1.6321654166204));
#22604=CARTESIAN_POINT('Ctrl Pts',(-0.711993139340447,-1.,-1.64752408828442));
#22605=CARTESIAN_POINT('Ctrl Pts',(-0.71958543378795,-1.,-1.66472880551777));
#22606=CARTESIAN_POINT('Ctrl Pts',(-0.726235967982445,-1.,-1.67996158451922));
#22607=CARTESIAN_POINT('Ctrl Pts',(-0.731963238685357,-1.,-1.69326921972915));
#22608=CARTESIAN_POINT('Ctrl Pts',(-0.736799665716932,-1.,-1.70473309004249));
#22609=CARTESIAN_POINT('Ctrl Pts',(-0.74079516202821,-1.,-1.71447789751001));
#22610=CARTESIAN_POINT('Ctrl Pts',(-0.744021445433093,-1.,-1.72268229916769));
#22611=CARTESIAN_POINT('Ctrl Pts',(-0.746574710097752,-1.,-1.72958533647714));
#22612=CARTESIAN_POINT('Ctrl Pts',(-0.74858246295687,-1.,-1.7355035168033));
#22613=CARTESIAN_POINT('Ctrl Pts',(-0.750193435981249,-1.,-1.74080458267114));
#22614=CARTESIAN_POINT('Ctrl Pts',(-0.751555614164482,-1.,-1.74585086852502));
#22615=CARTESIAN_POINT('Ctrl Pts',(-0.752797683531314,-1.,-1.75095139468794));
#22616=CARTESIAN_POINT('Ctrl Pts',(-0.754009254027829,-1.,-1.75631083600019));
#22617=CARTESIAN_POINT('Ctrl Pts',(-0.755220979974461,-1.,-1.76197817240128));
#22618=CARTESIAN_POINT('Ctrl Pts',(-0.75642189602781,-1.,-1.76789396002998));
#22619=CARTESIAN_POINT('Ctrl Pts',(-0.757578264077029,-1.,-1.77394167108292));
#22620=CARTESIAN_POINT('Ctrl Pts',(-0.758650626677518,-1.,-1.77999411220945));
#22621=CARTESIAN_POINT('Ctrl Pts',(-0.759614401110189,-1.,-1.78596964884604));
#22622=CARTESIAN_POINT('Ctrl Pts',(-0.760469555880749,-1.,-1.7918581561088));
#22623=CARTESIAN_POINT('Ctrl Pts',(-0.761229695230558,-1.,-1.79768986997783));
#22624=CARTESIAN_POINT('Ctrl Pts',(-0.761915336443547,-1.,-1.80351583877342));
#22625=CARTESIAN_POINT('Ctrl Pts',(-0.762546129463938,-1.,-1.80938551463965));
#22626=CARTESIAN_POINT('Ctrl Pts',(-0.763132003836634,-1.,-1.8153211840553));
#22627=CARTESIAN_POINT('Ctrl Pts',(-0.763673465462726,-1.,-1.82131873145266));
#22628=CARTESIAN_POINT('Ctrl Pts',(-0.764165902605995,-1.,-1.82735991200065));
#22629=CARTESIAN_POINT('Ctrl Pts',(-0.764602549687853,-1.,-1.83342077227142));
#22630=CARTESIAN_POINT('Ctrl Pts',(-0.764978057881737,-1.,-1.83948181064835));
#22631=CARTESIAN_POINT('Ctrl Pts',(-0.765291664862029,-1.,-1.84553698875924));
#22632=CARTESIAN_POINT('Ctrl Pts',(-0.765545710619062,-1.,-1.85158945130063));
#22633=CARTESIAN_POINT('Ctrl Pts',(-0.765744212909318,-1.,-1.85764741390394));
#22634=CARTESIAN_POINT('Ctrl Pts',(-0.765891519092547,-1.,-1.86372027063312));
#22635=CARTESIAN_POINT('Ctrl Pts',(-0.765990708546091,-1.,-1.86981398314341));
#22636=CARTESIAN_POINT('Ctrl Pts',(-0.766042837036744,-1.,-1.87592888967883));
#22637=CARTESIAN_POINT('Ctrl Pts',(-0.766047794851865,-1.,-1.88206215302561));
#22638=CARTESIAN_POINT('Ctrl Pts',(-0.766004837062091,-1.,-1.88820926433409));
#22639=CARTESIAN_POINT('Ctrl Pts',(-0.765913193856978,-1.,-1.89436577771388));
#22640=CARTESIAN_POINT('Ctrl Pts',(-0.765772772593386,-1.,-1.90052930393596));
#22641=CARTESIAN_POINT('Ctrl Pts',(-0.765584196937919,-1.,-1.90669961402356));
#22642=CARTESIAN_POINT('Ctrl Pts',(-0.765348465884722,-1.,-1.91287765805169));
#22643=CARTESIAN_POINT('Ctrl Pts',(-0.765066729667088,-1.,-1.91906491634196));
#22644=CARTESIAN_POINT('Ctrl Pts',(-0.764740025488211,-1.,-1.92526263537048));
#22645=CARTESIAN_POINT('Ctrl Pts',(-0.764369010673941,-1.,-1.93147105496382));
#22646=CARTESIAN_POINT('Ctrl Pts',(-0.763954049121458,-1.,-1.93768964875886));
#22647=CARTESIAN_POINT('Ctrl Pts',(-0.763495333538629,-1.,-1.9439174661764));
#22648=CARTESIAN_POINT('Ctrl Pts',(-0.762992990878769,-1.,-1.95015342590024));
#22649=CARTESIAN_POINT('Ctrl Pts',(-0.762447203806179,-1.,-1.95639665309869));
#22650=CARTESIAN_POINT('Ctrl Pts',(-0.761858300014423,-1.,-1.96264672744186));
#22651=CARTESIAN_POINT('Ctrl Pts',(-0.76122669048382,-1.,-1.96890351582499));
#22652=CARTESIAN_POINT('Ctrl Pts',(-0.760552825409757,-1.,-1.97516705321494));
#22653=CARTESIAN_POINT('Ctrl Pts',(-0.75983714745219,-1.,-1.98143741418172));
#22654=CARTESIAN_POINT('Ctrl Pts',(-0.759080037802488,-1.,-1.98771456680874));
#22655=CARTESIAN_POINT('Ctrl Pts',(-0.758281796766761,-1.,-1.99399831098817));
#22656=CARTESIAN_POINT('Ctrl Pts',(-0.757442676862724,-1.,-2.00028834739178));
#22657=CARTESIAN_POINT('Ctrl Pts',(-0.75656290464667,-1.,-2.0065843158773));
#22658=CARTESIAN_POINT('Ctrl Pts',(-0.755642704957865,-1.,-2.01288584328084));
#22659=CARTESIAN_POINT('Ctrl Pts',(-0.754682330722816,-1.,-2.01919259405809));
#22660=CARTESIAN_POINT('Ctrl Pts',(-0.753682061112768,-1.,-2.02550428623313));
#22661=CARTESIAN_POINT('Ctrl Pts',(-0.752642180487211,-1.,-2.03182068456221));
#22662=CARTESIAN_POINT('Ctrl Pts',(-0.751562963361115,-1.,-2.03814160092099));
#22663=CARTESIAN_POINT('Ctrl Pts',(-0.750444657875576,-1.,-2.04446689147979));
#22664=CARTESIAN_POINT('Ctrl Pts',(-0.749287468665046,-1.,-2.05079645592154));
#22665=CARTESIAN_POINT('Ctrl Pts',(-0.748091554183802,-1.,-2.05713023031006));
#22666=CARTESIAN_POINT('Ctrl Pts',(-0.747103932787919,-1.,-2.06220058927826));
#22667=CARTESIAN_POINT('Ctrl Pts',(-0.7463458715442,-1.,-2.06600523016815));
#22668=CARTESIAN_POINT('Ctrl Pts',(-0.745832791378367,-1.,-2.06854248895728));
#22669=CARTESIAN_POINT('Ctrl Pts',(-0.745574324794401,-1.,-2.0698113262342));
#22670=CARTESIAN_POINT('',(-0.61342227326009,-1.,-2.11275013067528));
#22671=CARTESIAN_POINT('',(-0.745574324794401,-1.,-2.0698113262342));
#22672=CARTESIAN_POINT('',(-0.383122945602004,-1.,-1.7075470150345));
#22673=CARTESIAN_POINT('Ctrl Pts',(-0.61342227326009,-1.,-2.11275013067528));
#22674=CARTESIAN_POINT('Ctrl Pts',(-0.6124673655618,-1.,-2.11187554259986));
#22675=CARTESIAN_POINT('Ctrl Pts',(-0.610560911689899,-1.,-2.11012443807238));
#22676=CARTESIAN_POINT('Ctrl Pts',(-0.607711315454876,-1.,-2.1074919961518));
#22677=CARTESIAN_POINT('Ctrl Pts',(-0.60393203073603,-1.,-2.10397049886949));
#22678=CARTESIAN_POINT('Ctrl Pts',(-0.599241616420533,-1.,-2.0995493086477));
#22679=CARTESIAN_POINT('Ctrl Pts',(-0.594585006052162,-1.,-2.0951087622027));
#22680=CARTESIAN_POINT('Ctrl Pts',(-0.589962365403406,-1.,-2.09064881812129));
#22681=CARTESIAN_POINT('Ctrl Pts',(-0.585373918991617,-1.,-2.08616943727951));
#22682=CARTESIAN_POINT('Ctrl Pts',(-0.580819952108063,-1.,-2.08167059018418));
#22683=CARTESIAN_POINT('Ctrl Pts',(-0.576300797416844,-1.,-2.07715226767559));
#22684=CARTESIAN_POINT('Ctrl Pts',(-0.571816823242603,-1.,-2.07261449292824));
#22685=CARTESIAN_POINT('Ctrl Pts',(-0.567368421181087,-1.,-2.06805732997334));
#22686=CARTESIAN_POINT('Ctrl Pts',(-0.562955993082261,-1.,-2.06348090160589));
#22687=CARTESIAN_POINT('Ctrl Pts',(-0.558579940185151,-1.,-2.05888537756462));
#22688=CARTESIAN_POINT('Ctrl Pts',(-0.554240657463906,-1.,-2.05427091604413));
#22689=CARTESIAN_POINT('Ctrl Pts',(-0.549938525150295,-1.,-2.04963761077958));
#22690=CARTESIAN_POINT('Ctrl Pts',(-0.54567390381743,-1.,-2.04498544714588));
#22691=CARTESIAN_POINT('Ctrl Pts',(-0.541447120615659,-1.,-2.04031422690527));
#22692=CARTESIAN_POINT('Ctrl Pts',(-0.537258489833262,-1.,-2.03562362954037));
#22693=CARTESIAN_POINT('Ctrl Pts',(-0.533108355132977,-1.,-2.03091336214426));
#22694=CARTESIAN_POINT('Ctrl Pts',(-0.528997127241914,-1.,-2.0261832908329));
#22695=CARTESIAN_POINT('Ctrl Pts',(-0.524925318333476,-1.,-2.02143356304698));
#22696=CARTESIAN_POINT('Ctrl Pts',(-0.52089359039937,-1.,-2.01666477917286));
#22697=CARTESIAN_POINT('Ctrl Pts',(-0.516902681728687,-1.,-2.01187773939242));
#22698=CARTESIAN_POINT('Ctrl Pts',(-0.512953306961792,-1.,-2.00707309946949));
#22699=CARTESIAN_POINT('Ctrl Pts',(-0.509046069886157,-1.,-2.00225107134734));
#22700=CARTESIAN_POINT('Ctrl Pts',(-0.505181361323026,-1.,-1.99741107463572));
#22701=CARTESIAN_POINT('Ctrl Pts',(-0.501359287727146,-1.,-1.99255149126155));
#22702=CARTESIAN_POINT('Ctrl Pts',(-0.497579909545574,-1.,-1.98767044752932));
#22703=CARTESIAN_POINT('Ctrl Pts',(-0.493843476541495,-1.,-1.98276658761821));
#22704=CARTESIAN_POINT('Ctrl Pts',(-0.490150627860952,-1.,-1.97783973019229));
#22705=CARTESIAN_POINT('Ctrl Pts',(-0.486502692907659,-1.,-1.97289186263272));
#22706=CARTESIAN_POINT('Ctrl Pts',(-0.482901662120691,-1.,-1.96792703422362));
#22707=CARTESIAN_POINT('Ctrl Pts',(-0.479349583074855,-1.,-1.96294933055943));
#22708=CARTESIAN_POINT('Ctrl Pts',(-0.475848034683176,-1.,-1.95796111148177));
#22709=CARTESIAN_POINT('Ctrl Pts',(-0.472397672264072,-1.,-1.95296148278133));
#22710=CARTESIAN_POINT('Ctrl Pts',(-0.468997482913135,-1.,-1.94794381136514));
#22711=CARTESIAN_POINT('Ctrl Pts',(-0.46564546202603,-1.,-1.9428979419619));
#22712=CARTESIAN_POINT('Ctrl Pts',(-0.462340031009056,-1.,-1.93781486640821));
#22713=CARTESIAN_POINT('Ctrl Pts',(-0.459081234547926,-1.,-1.93269066517934));
#22714=CARTESIAN_POINT('Ctrl Pts',(-0.455872005174371,-1.,-1.92753067150476));
#22715=CARTESIAN_POINT('Ctrl Pts',(-0.452719478359432,-1.,-1.92235380648502));
#22716=CARTESIAN_POINT('Ctrl Pts',(-0.449632260106662,-1.,-1.91718342555755));
#22717=CARTESIAN_POINT('Ctrl Pts',(-0.446617343485711,-1.,-1.9120369998112));
#22718=CARTESIAN_POINT('Ctrl Pts',(-0.443677556849151,-1.,-1.90691756144898));
#22719=CARTESIAN_POINT('Ctrl Pts',(-0.440807833704038,-1.,-1.90180124389086));
#22720=CARTESIAN_POINT('Ctrl Pts',(-0.437995003948244,-1.,-1.89663648956466));
#22721=CARTESIAN_POINT('Ctrl Pts',(-0.435225660963383,-1.,-1.89136993975504));
#22722=CARTESIAN_POINT('Ctrl Pts',(-0.432493038548748,-1.,-1.88596913666793));
#22723=CARTESIAN_POINT('Ctrl Pts',(-0.429803062482344,-1.,-1.88044229001832));
#22724=CARTESIAN_POINT('Ctrl Pts',(-0.427183828519102,-1.,-1.87486989291484));
#22725=CARTESIAN_POINT('Ctrl Pts',(-0.424678177291359,-1.,-1.86937803944323));
#22726=CARTESIAN_POINT('Ctrl Pts',(-0.422327307418275,-1.,-1.86408083334028));
#22727=CARTESIAN_POINT('Ctrl Pts',(-0.420157287975619,-1.,-1.85903281096686));
#22728=CARTESIAN_POINT('Ctrl Pts',(-0.418164129143534,-1.,-1.85417632856234));
#22729=CARTESIAN_POINT('Ctrl Pts',(-0.416300022038864,-1.,-1.84929312929882));
#22730=CARTESIAN_POINT('Ctrl Pts',(-0.41448743825434,-1.,-1.8440575707371));
#22731=CARTESIAN_POINT('Ctrl Pts',(-0.412633125322162,-1.,-1.83808953475839));
#22732=CARTESIAN_POINT('Ctrl Pts',(-0.410641256301675,-1.,-1.83100408895216));
#22733=CARTESIAN_POINT('Ctrl Pts',(-0.408428948108533,-1.,-1.8224702267854));
#22734=CARTESIAN_POINT('Ctrl Pts',(-0.405933518411838,-1.,-1.81223801813988));
#22735=CARTESIAN_POINT('Ctrl Pts',(-0.403107976170441,-1.,-1.80012077176221));
#22736=CARTESIAN_POINT('Ctrl Pts',(-0.39991940378308,-1.,-1.78598826347533));
#22737=CARTESIAN_POINT('Ctrl Pts',(-0.39634619612042,-1.,-1.7697556004756));
#22738=CARTESIAN_POINT('Ctrl Pts',(-0.392375812294307,-1.,-1.75137405313962));
#22739=CARTESIAN_POINT('Ctrl Pts',(-0.388877023509191,-1.,-1.7349317097561));
#22740=CARTESIAN_POINT('Ctrl Pts',(-0.38607079032701,-1.,-1.72162022246158));
#22741=CARTESIAN_POINT('Ctrl Pts',(-0.384119047315542,-1.,-1.71231062891958));
#22742=CARTESIAN_POINT('Ctrl Pts',(-0.383122945602004,-1.,-1.7075470150345));
#22743=CARTESIAN_POINT('',(-0.163289472382896,-1.,-1.74236521665491));
#22744=CARTESIAN_POINT('Origin',(0.,-1.,0.));
#22745=CARTESIAN_POINT('',(-0.0694764450219581,-1.,-2.19890268624765));
#22746=CARTESIAN_POINT('Ctrl Pts',(-0.163289472382896,-1.,-1.74236521665491));
#22747=CARTESIAN_POINT('Ctrl Pts',(-0.163814161002002,-1.,-1.7472034950333));
#22748=CARTESIAN_POINT('Ctrl Pts',(-0.164834765707158,-1.,-1.75666056638427));
#22749=CARTESIAN_POINT('Ctrl Pts',(-0.1662793551464,-1.,-1.77018771684844));
#22750=CARTESIAN_POINT('Ctrl Pts',(-0.168032772805197,-1.,-1.7869064998507));
#22751=CARTESIAN_POINT('Ctrl Pts',(-0.169936923904608,-1.,-1.80561530629706));
#22752=CARTESIAN_POINT('Ctrl Pts',(-0.171554770204119,-1.,-1.82215766811545));
#22753=CARTESIAN_POINT('Ctrl Pts',(-0.1728894428919,-1.,-1.83658380527692));
#22754=CARTESIAN_POINT('Ctrl Pts',(-0.173946627587731,-1.,-1.8489811319852));
#22755=CARTESIAN_POINT('Ctrl Pts',(-0.17473525927603,-1.,-1.85948367088837));
#22756=CARTESIAN_POINT('Ctrl Pts',(-0.175268337590758,-1.,-1.86828349694799));
#22757=CARTESIAN_POINT('Ctrl Pts',(-0.175563480746485,-1.,-1.87563767773588));
#22758=CARTESIAN_POINT('Ctrl Pts',(-0.175644148889699,-1.,-1.88188663145367));
#22759=CARTESIAN_POINT('Ctrl Pts',(-0.175538155840648,-1.,-1.88742606273259));
#22760=CARTESIAN_POINT('Ctrl Pts',(-0.175274276190844,-1.,-1.892646301985));
#22761=CARTESIAN_POINT('Ctrl Pts',(-0.174879405091263,-1.,-1.89788101117132));
#22762=CARTESIAN_POINT('Ctrl Pts',(-0.174375518661085,-1.,-1.90335253862834));
#22763=CARTESIAN_POINT('Ctrl Pts',(-0.173776635257817,-1.,-1.90911693975267));
#22764=CARTESIAN_POINT('Ctrl Pts',(-0.173090695383496,-1.,-1.91511429159527));
#22765=CARTESIAN_POINT('Ctrl Pts',(-0.172321621259514,-1.,-1.9212233439798));
#22766=CARTESIAN_POINT('Ctrl Pts',(-0.171471191532988,-1.,-1.92731093582036));
#22767=CARTESIAN_POINT('Ctrl Pts',(-0.170541253116202,-1.,-1.93329183155539));
#22768=CARTESIAN_POINT('Ctrl Pts',(-0.169534904817491,-1.,-1.93915639211581));
#22769=CARTESIAN_POINT('Ctrl Pts',(-0.168455741607556,-1.,-1.94493757756931));
#22770=CARTESIAN_POINT('Ctrl Pts',(-0.167307501784475,-1.,-1.95069027794294));
#22771=CARTESIAN_POINT('Ctrl Pts',(-0.166093592002812,-1.,-1.9564675971873));
#22772=CARTESIAN_POINT('Ctrl Pts',(-0.164816568920269,-1.,-1.96229379940136));
#22773=CARTESIAN_POINT('Ctrl Pts',(-0.163478185457734,-1.,-1.96816512677967));
#22774=CARTESIAN_POINT('Ctrl Pts',(-0.162079693556289,-1.,-1.97406280235188));
#22775=CARTESIAN_POINT('Ctrl Pts',(-0.160622060784611,-1.,-1.97996195437559));
#22776=CARTESIAN_POINT('Ctrl Pts',(-0.159106226437299,-1.,-1.98584238283292));
#22777=CARTESIAN_POINT('Ctrl Pts',(-0.157533331459227,-1.,-1.99169810931908));
#22778=CARTESIAN_POINT('Ctrl Pts',(-0.155904629548783,-1.,-1.99753284771497));
#22779=CARTESIAN_POINT('Ctrl Pts',(-0.154221403049722,-1.,-2.00335565310543));
#22780=CARTESIAN_POINT('Ctrl Pts',(-0.15248488362145,-1.,-2.00917680318424));
#22781=CARTESIAN_POINT('Ctrl Pts',(-0.150696157673078,-1.,-2.01500291940238));
#22782=CARTESIAN_POINT('Ctrl Pts',(-0.148856124775337,-1.,-2.02083464969894));
#22783=CARTESIAN_POINT('Ctrl Pts',(-0.146965557332583,-1.,-2.02666926182017));
#22784=CARTESIAN_POINT('Ctrl Pts',(-0.145025140186057,-1.,-2.03250223739942));
#22785=CARTESIAN_POINT('Ctrl Pts',(-0.143035515058209,-1.,-2.03832911025912));
#22786=CARTESIAN_POINT('Ctrl Pts',(-0.140997332152546,-1.,-2.04414757947916));
#22787=CARTESIAN_POINT('Ctrl Pts',(-0.138911255368966,-1.,-2.04995762001328));
#22788=CARTESIAN_POINT('Ctrl Pts',(-0.136777941218044,-1.,-2.05576044414264));
#22789=CARTESIAN_POINT('Ctrl Pts',(-0.134598026192106,-1.,-2.06155781517842));
#22790=CARTESIAN_POINT('Ctrl Pts',(-0.13237211154771,-1.,-2.06735123910326));
#22791=CARTESIAN_POINT('Ctrl Pts',(-0.130100748328403,-1.,-2.07314114713063));
#22792=CARTESIAN_POINT('Ctrl Pts',(-0.12778444527612,-1.,-2.07892715110987));
#22793=CARTESIAN_POINT('Ctrl Pts',(-0.125423679412061,-1.,-2.08470840653643));
#22794=CARTESIAN_POINT('Ctrl Pts',(-0.123018905621083,-1.,-2.09048392424825));
#22795=CARTESIAN_POINT('Ctrl Pts',(-0.120570567965122,-1.,-2.0962529286773));
#22796=CARTESIAN_POINT('Ctrl Pts',(-0.118079107988355,-1.,-2.102015121329));
#22797=CARTESIAN_POINT('Ctrl Pts',(-0.115544957687926,-1.,-2.10777050261309));
#22798=CARTESIAN_POINT('Ctrl Pts',(-0.112968534419737,-1.,-2.11351924490306));
#22799=CARTESIAN_POINT('Ctrl Pts',(-0.110350236135025,-1.,-2.11926155590865));
#22800=CARTESIAN_POINT('Ctrl Pts',(-0.10769043523109,-1.,-2.12499752307));
#22801=CARTESIAN_POINT('Ctrl Pts',(-0.104989479152739,-1.,-2.13072704887293));
#22802=CARTESIAN_POINT('Ctrl Pts',(-0.1022477005561,-1.,-2.13644992667165));
#22803=CARTESIAN_POINT('Ctrl Pts',(-0.0994654261990915,-1.,-2.14216588396025));
#22804=CARTESIAN_POINT('Ctrl Pts',(-0.0966429852305459,-1.,-2.14787463531795));
#22805=CARTESIAN_POINT('Ctrl Pts',(-0.0937807218867643,-1.,-2.1535759397817));
#22806=CARTESIAN_POINT('Ctrl Pts',(-0.0908789888107265,-1.,-2.15926961544516));
#22807=CARTESIAN_POINT('Ctrl Pts',(-0.0879381291386923,-1.,-2.16495552645014));
#22808=CARTESIAN_POINT('Ctrl Pts',(-0.0849584620835372,-1.,-2.17063357870952));
#22809=CARTESIAN_POINT('Ctrl Pts',(-0.0819402680872765,-1.,-2.176303712113));
#22810=CARTESIAN_POINT('Ctrl Pts',(-0.0788837727685243,-1.,-2.18196589448887));
#22811=CARTESIAN_POINT('Ctrl Pts',(-0.0757891465836148,-1.,-2.1876201139953));
#22812=CARTESIAN_POINT('Ctrl Pts',(-0.0732830357306725,-1.,-2.19213712013662));
#22813=CARTESIAN_POINT('Ctrl Pts',(-0.0713863779526154,-1.,-2.19552129484002));
#22814=CARTESIAN_POINT('Ctrl Pts',(-0.070114353632549,-1.,-2.19777582085423));
#22815=CARTESIAN_POINT('Ctrl Pts',(-0.0694764450219581,-1.,-2.19890268624765));
#22816=CARTESIAN_POINT('',(0.0694764450219584,-1.,-2.19890268624765));
#22817=CARTESIAN_POINT('',(-0.0694764450219581,-1.,-2.19890268624765));
#22818=CARTESIAN_POINT('',(0.163289472382896,-1.,-1.74236521665491));
#22819=CARTESIAN_POINT('Ctrl Pts',(0.0694764450219584,-1.,-2.19890268624765));
#22820=CARTESIAN_POINT('Ctrl Pts',(0.0701143536324926,-1.,-2.19777582085261));
#22821=CARTESIAN_POINT('Ctrl Pts',(0.0713863779524627,-1.,-2.19552129483562));
#22822=CARTESIAN_POINT('Ctrl Pts',(0.0732830357304276,-1.,-2.19213712012956));
#22823=CARTESIAN_POINT('Ctrl Pts',(0.0757891465833411,-1.,-2.1876201139874));
#22824=CARTESIAN_POINT('Ctrl Pts',(0.0788837727683228,-1.,-2.18196589448304));
#22825=CARTESIAN_POINT('Ctrl Pts',(0.0819402680871939,-1.,-2.1763037121106));
#22826=CARTESIAN_POINT('Ctrl Pts',(0.0849584620835643,-1.,-2.17063357871031));
#22827=CARTESIAN_POINT('Ctrl Pts',(0.0879381291387823,-1.,-2.16495552645275));
#22828=CARTESIAN_POINT('Ctrl Pts',(0.0908789888108266,-1.,-2.15926961544808));
#22829=CARTESIAN_POINT('Ctrl Pts',(0.0937807218868345,-1.,-2.15357593978377));
#22830=CARTESIAN_POINT('Ctrl Pts',(0.0966429852305689,-1.,-2.14787463531864));
#22831=CARTESIAN_POINT('Ctrl Pts',(0.0994654261990743,-1.,-2.14216588395974));
#22832=CARTESIAN_POINT('Ctrl Pts',(0.102247700556064,-1.,-2.13644992667052));
#22833=CARTESIAN_POINT('Ctrl Pts',(0.104989479152703,-1.,-2.1307270488718));
#22834=CARTESIAN_POINT('Ctrl Pts',(0.107690435231068,-1.,-2.12499752306927));
#22835=CARTESIAN_POINT('Ctrl Pts',(0.11035023613502,-1.,-2.11926155590849));
#22836=CARTESIAN_POINT('Ctrl Pts',(0.112968534419746,-1.,-2.11351924490335));
#22837=CARTESIAN_POINT('Ctrl Pts',(0.11554495768794,-1.,-2.10777050261359));
#22838=CARTESIAN_POINT('Ctrl Pts',(0.118079107988368,-1.,-2.10201512132945));
#22839=CARTESIAN_POINT('Ctrl Pts',(0.120570567965129,-1.,-2.09625292867756));
#22840=CARTESIAN_POINT('Ctrl Pts',(0.123018905621083,-1.,-2.09048392424826));
#22841=CARTESIAN_POINT('Ctrl Pts',(0.125423679412058,-1.,-2.08470840653628));
#22842=CARTESIAN_POINT('Ctrl Pts',(0.127784445276116,-1.,-2.07892715110967));
#22843=CARTESIAN_POINT('Ctrl Pts',(0.1301007483284,-1.,-2.07314114713047));
#22844=CARTESIAN_POINT('Ctrl Pts',(0.13237211154771,-1.,-2.06735123910319));
#22845=CARTESIAN_POINT('Ctrl Pts',(0.134598026192107,-1.,-2.06155781517844));
#22846=CARTESIAN_POINT('Ctrl Pts',(0.136777941218044,-1.,-2.0557604441427));
#22847=CARTESIAN_POINT('Ctrl Pts',(0.138911255368966,-1.,-2.04995762001333));
#22848=CARTESIAN_POINT('Ctrl Pts',(0.140997332152545,-1.,-2.04414757947919));
#22849=CARTESIAN_POINT('Ctrl Pts',(0.143035515058208,-1.,-2.03832911025913));
#22850=CARTESIAN_POINT('Ctrl Pts',(0.145025140186058,-1.,-2.03250223739941));
#22851=CARTESIAN_POINT('Ctrl Pts',(0.146965557332586,-1.,-2.02666926182017));
#22852=CARTESIAN_POINT('Ctrl Pts',(0.148856124775343,-1.,-2.02083464969897));
#22853=CARTESIAN_POINT('Ctrl Pts',(0.150696157673084,-1.,-2.01500291940243));
#22854=CARTESIAN_POINT('Ctrl Pts',(0.152484883621452,-1.,-2.00917680318426));
#22855=CARTESIAN_POINT('Ctrl Pts',(0.154221403049719,-1.,-2.00335565310539));
#22856=CARTESIAN_POINT('Ctrl Pts',(0.155904629548774,-1.,-1.99753284771487));
#22857=CARTESIAN_POINT('Ctrl Pts',(0.157533331459215,-1.,-1.99169810931893));
#22858=CARTESIAN_POINT('Ctrl Pts',(0.159106226437288,-1.,-1.98584238283279));
#22859=CARTESIAN_POINT('Ctrl Pts',(0.16062206078461,-1.,-1.97996195437557));
#22860=CARTESIAN_POINT('Ctrl Pts',(0.162079693556302,-1.,-1.97406280235204));
#22861=CARTESIAN_POINT('Ctrl Pts',(0.16347818545776,-1.,-1.96816512678));
#22862=CARTESIAN_POINT('Ctrl Pts',(0.1648165689203,-1.,-1.96229379940174));
#22863=CARTESIAN_POINT('Ctrl Pts',(0.166093592002833,-1.,-1.95646759718755));
#22864=CARTESIAN_POINT('Ctrl Pts',(0.167307501784469,-1.,-1.95069027794286));
#22865=CARTESIAN_POINT('Ctrl Pts',(0.168455741607516,-1.,-1.94493757756879));
#22866=CARTESIAN_POINT('Ctrl Pts',(0.169534904817425,-1.,-1.93915639211497));
#22867=CARTESIAN_POINT('Ctrl Pts',(0.170541253116136,-1.,-1.93329183155455));
#22868=CARTESIAN_POINT('Ctrl Pts',(0.17147119153296,-1.,-1.92731093582));
#22869=CARTESIAN_POINT('Ctrl Pts',(0.172321621259557,-1.,-1.92122334398034));
#22870=CARTESIAN_POINT('Ctrl Pts',(0.173090695383619,-1.,-1.91511429159681));
#22871=CARTESIAN_POINT('Ctrl Pts',(0.173776635257984,-1.,-1.90911693975475));
#22872=CARTESIAN_POINT('Ctrl Pts',(0.174375518661222,-1.,-1.90335253863003));
#22873=CARTESIAN_POINT('Ctrl Pts',(0.174879405091277,-1.,-1.89788101117148));
#22874=CARTESIAN_POINT('Ctrl Pts',(0.175274276190664,-1.,-1.89264630198279));
#22875=CARTESIAN_POINT('Ctrl Pts',(0.175538155840286,-1.,-1.88742606272818));
#22876=CARTESIAN_POINT('Ctrl Pts',(0.175644148889271,-1.,-1.88188663144846));
#22877=CARTESIAN_POINT('Ctrl Pts',(0.175563480746205,-1.,-1.87563767773249));
#22878=CARTESIAN_POINT('Ctrl Pts',(0.175268337590901,-1.,-1.86828349694972));
#22879=CARTESIAN_POINT('Ctrl Pts',(0.174735259276856,-1.,-1.85948367089838));
#22880=CARTESIAN_POINT('Ctrl Pts',(0.173946627589401,-1.,-1.84898113200543));
#22881=CARTESIAN_POINT('Ctrl Pts',(0.17288944289442,-1.,-1.83658380530747));
#22882=CARTESIAN_POINT('Ctrl Pts',(0.171554770207306,-1.,-1.82215766815414));
#22883=CARTESIAN_POINT('Ctrl Pts',(0.169936923908078,-1.,-1.80561530633924));
#22884=CARTESIAN_POINT('Ctrl Pts',(0.16803277280837,-1.,-1.78690649988931));
#22885=CARTESIAN_POINT('Ctrl Pts',(0.166279355148738,-1.,-1.77018771687692));
#22886=CARTESIAN_POINT('Ctrl Pts',(0.164834765708484,-1.,-1.75666056640041));
#22887=CARTESIAN_POINT('Ctrl Pts',(0.163814161002474,-1.,-1.74720349503904));
#22888=CARTESIAN_POINT('Ctrl Pts',(0.163289472382896,-1.,-1.74236521665491));
#22889=CARTESIAN_POINT('',(0.383122945602004,-1.,-1.7075470150345));
#22890=CARTESIAN_POINT('Origin',(0.,-1.,0.));
#22891=CARTESIAN_POINT('',(0.61342227326009,-1.,-2.11275013067528));
#22892=CARTESIAN_POINT('Ctrl Pts',(0.383122945602004,-1.,-1.7075470150345));
#22893=CARTESIAN_POINT('Ctrl Pts',(0.384119047314215,-1.,-1.71231062891398));
#22894=CARTESIAN_POINT('Ctrl Pts',(0.386070790323281,-1.,-1.72162022244582));
#22895=CARTESIAN_POINT('Ctrl Pts',(0.388877023502615,-1.,-1.73493170972829));
#22896=CARTESIAN_POINT('Ctrl Pts',(0.392375812285395,-1.,-1.75137405310193));
#22897=CARTESIAN_POINT('Ctrl Pts',(0.396346196110688,-1.,-1.76975560043442));
#22898=CARTESIAN_POINT('Ctrl Pts',(0.399919403774155,-1.,-1.78598826343754));
#22899=CARTESIAN_POINT('Ctrl Pts',(0.403107976163396,-1.,-1.80012077173238));
#22900=CARTESIAN_POINT('Ctrl Pts',(0.405933518407175,-1.,-1.81223801812013));
#22901=CARTESIAN_POINT('Ctrl Pts',(0.408428948106227,-1.,-1.82247022677562));
#22902=CARTESIAN_POINT('Ctrl Pts',(0.410641256301276,-1.,-1.83100408895047));
#22903=CARTESIAN_POINT('Ctrl Pts',(0.412633125322945,-1.,-1.8380895347617));
#22904=CARTESIAN_POINT('Ctrl Pts',(0.414487438255542,-1.,-1.84405757074218));
#22905=CARTESIAN_POINT('Ctrl Pts',(0.416300022039885,-1.,-1.84929312930314));
#22906=CARTESIAN_POINT('Ctrl Pts',(0.418164129144045,-1.,-1.8541763285645));
#22907=CARTESIAN_POINT('Ctrl Pts',(0.420157287975583,-1.,-1.8590328109667));
#22908=CARTESIAN_POINT('Ctrl Pts',(0.422327307417884,-1.,-1.86408083333863));
#22909=CARTESIAN_POINT('Ctrl Pts',(0.424678177290876,-1.,-1.8693780394412));
#22910=CARTESIAN_POINT('Ctrl Pts',(0.427183828518743,-1.,-1.87486989291334));
#22911=CARTESIAN_POINT('Ctrl Pts',(0.429803062482217,-1.,-1.88044229001779));
#22912=CARTESIAN_POINT('Ctrl Pts',(0.432493038548833,-1.,-1.88596913666828));
#22913=CARTESIAN_POINT('Ctrl Pts',(0.43522566096358,-1.,-1.89136993975585));
#22914=CARTESIAN_POINT('Ctrl Pts',(0.437995003948443,-1.,-1.89663648956549));
#22915=CARTESIAN_POINT('Ctrl Pts',(0.44080783370416,-1.,-1.90180124389137));
#22916=CARTESIAN_POINT('Ctrl Pts',(0.44367755684917,-1.,-1.90691756144906));
#22917=CARTESIAN_POINT('Ctrl Pts',(0.446617343485651,-1.,-1.91203699981095));
#22918=CARTESIAN_POINT('Ctrl Pts',(0.449632260106572,-1.,-1.91718342555717));
#22919=CARTESIAN_POINT('Ctrl Pts',(0.452719478359356,-1.,-1.9223538064847));
#22920=CARTESIAN_POINT('Ctrl Pts',(0.455872005174335,-1.,-1.92753067150461));
#22921=CARTESIAN_POINT('Ctrl Pts',(0.459081234547931,-1.,-1.93269066517936));
#22922=CARTESIAN_POINT('Ctrl Pts',(0.462340031009087,-1.,-1.93781486640834));
#22923=CARTESIAN_POINT('Ctrl Pts',(0.465645462026064,-1.,-1.94289794196205));
#22924=CARTESIAN_POINT('Ctrl Pts',(0.468997482913158,-1.,-1.94794381136524));
#22925=CARTESIAN_POINT('Ctrl Pts',(0.472397672264079,-1.,-1.95296148278136));
#22926=CARTESIAN_POINT('Ctrl Pts',(0.475848034683171,-1.,-1.95796111148175));
#22927=CARTESIAN_POINT('Ctrl Pts',(0.479349583074846,-1.,-1.96294933055938));
#22928=CARTESIAN_POINT('Ctrl Pts',(0.482901662120686,-1.,-1.96792703422358));
#22929=CARTESIAN_POINT('Ctrl Pts',(0.486502692907661,-1.,-1.97289186263272));
#22930=CARTESIAN_POINT('Ctrl Pts',(0.490150627860955,-1.,-1.97783973019229));
#22931=CARTESIAN_POINT('Ctrl Pts',(0.493843476541492,-1.,-1.9827665876182));
#22932=CARTESIAN_POINT('Ctrl Pts',(0.497579909545564,-1.,-1.98767044752929));
#22933=CARTESIAN_POINT('Ctrl Pts',(0.501359287727129,-1.,-1.9925514912615));
#22934=CARTESIAN_POINT('Ctrl Pts',(0.505181361323011,-1.,-1.99741107463567));
#22935=CARTESIAN_POINT('Ctrl Pts',(0.509046069886152,-1.,-2.00225107134733));
#22936=CARTESIAN_POINT('Ctrl Pts',(0.512953306961813,-1.,-2.00707309946955));
#22937=CARTESIAN_POINT('Ctrl Pts',(0.516902681728733,-1.,-2.01187773939257));
#22938=CARTESIAN_POINT('Ctrl Pts',(0.520893590399428,-1.,-2.01666477917306));
#22939=CARTESIAN_POINT('Ctrl Pts',(0.524925318333518,-1.,-2.02143356304712));
#22940=CARTESIAN_POINT('Ctrl Pts',(0.52899712724191,-1.,-2.02618329083289));
#22941=CARTESIAN_POINT('Ctrl Pts',(0.533108355132905,-1.,-2.03091336214401));
#22942=CARTESIAN_POINT('Ctrl Pts',(0.537258489833134,-1.,-2.03562362953993));
#22943=CARTESIAN_POINT('Ctrl Pts',(0.54144712061552,-1.,-2.0403142269048));
#22944=CARTESIAN_POINT('Ctrl Pts',(0.545673903817348,-1.,-2.0449854471456));
#22945=CARTESIAN_POINT('Ctrl Pts',(0.549938525150342,-1.,-2.04963761077974));
#22946=CARTESIAN_POINT('Ctrl Pts',(0.554240657464109,-1.,-2.05427091604482));
#22947=CARTESIAN_POINT('Ctrl Pts',(0.558579940185467,-1.,-2.05888537756571));
#22948=CARTESIAN_POINT('Ctrl Pts',(0.562955993082574,-1.,-2.06348090160697));
#22949=CARTESIAN_POINT('Ctrl Pts',(0.567368421181229,-1.,-2.06805732997383));
#22950=CARTESIAN_POINT('Ctrl Pts',(0.571816823242411,-1.,-2.07261449292758));
#22951=CARTESIAN_POINT('Ctrl Pts',(0.576300797416274,-1.,-2.07715226767361));
#22952=CARTESIAN_POINT('Ctrl Pts',(0.580819952107256,-1.,-2.08167059018138));
#22953=CARTESIAN_POINT('Ctrl Pts',(0.585373918990895,-1.,-2.086169437277));
#22954=CARTESIAN_POINT('Ctrl Pts',(0.589962365403189,-1.,-2.09064881812053));
#22955=CARTESIAN_POINT('Ctrl Pts',(0.594585006052823,-1.,-2.09510876220501));
#22956=CARTESIAN_POINT('Ctrl Pts',(0.599241616422144,-1.,-2.09954930865331));
#22957=CARTESIAN_POINT('Ctrl Pts',(0.603932030738212,-1.,-2.10397049887709));
#22958=CARTESIAN_POINT('Ctrl Pts',(0.607711315456826,-1.,-2.10749199615859));
#22959=CARTESIAN_POINT('Ctrl Pts',(0.610560911691113,-1.,-2.11012443807661));
#22960=CARTESIAN_POINT('Ctrl Pts',(0.61246736556225,-1.,-2.11187554260142));
#22961=CARTESIAN_POINT('Ctrl Pts',(0.61342227326009,-1.,-2.11275013067528));
#22962=CARTESIAN_POINT('',(0.745574324794401,-1.,-2.0698113262342));
#22963=CARTESIAN_POINT('',(0.61342227326009,-1.,-2.11275013067528));
#22964=CARTESIAN_POINT('',(0.693717979106306,-1.,-1.60662857109684));
#22965=CARTESIAN_POINT('Ctrl Pts',(0.745574324794401,-1.,-2.0698113262342));
#22966=CARTESIAN_POINT('Ctrl Pts',(0.74583279137781,-1.,-2.06854248895575));
#22967=CARTESIAN_POINT('Ctrl Pts',(0.746345871542695,-1.,-2.06600523016401));
#22968=CARTESIAN_POINT('Ctrl Pts',(0.747103932785504,-1.,-2.06220058927162));
#22969=CARTESIAN_POINT('Ctrl Pts',(0.748091554181101,-1.,-2.05713023030263));
#22970=CARTESIAN_POINT('Ctrl Pts',(0.749287468663053,-1.,-2.05079645591606));
#22971=CARTESIAN_POINT('Ctrl Pts',(0.750444657874758,-1.,-2.04446689147754));
#22972=CARTESIAN_POINT('Ctrl Pts',(0.751562963361383,-1.,-2.03814160092173));
#22973=CARTESIAN_POINT('Ctrl Pts',(0.752642180488104,-1.,-2.03182068456467));
#22974=CARTESIAN_POINT('Ctrl Pts',(0.753682061113765,-1.,-2.02550428623587));
#22975=CARTESIAN_POINT('Ctrl Pts',(0.75468233072352,-1.,-2.01919259406003));
#22976=CARTESIAN_POINT('Ctrl Pts',(0.7556427049581,-1.,-2.01288584328149));
#22977=CARTESIAN_POINT('Ctrl Pts',(0.756562904646496,-1.,-2.00658431587682));
#22978=CARTESIAN_POINT('Ctrl Pts',(0.757442676862341,-1.,-2.00028834739072));
#22979=CARTESIAN_POINT('Ctrl Pts',(0.758281796766377,-1.,-1.9939983109871));
#22980=CARTESIAN_POINT('Ctrl Pts',(0.759080037802242,-1.,-1.98771456680806));
#22981=CARTESIAN_POINT('Ctrl Pts',(0.759837147452135,-1.,-1.98143741418156));
#22982=CARTESIAN_POINT('Ctrl Pts',(0.760552825409855,-1.,-1.97516705321521));
#22983=CARTESIAN_POINT('Ctrl Pts',(0.761226690483986,-1.,-1.96890351582545));
#22984=CARTESIAN_POINT('Ctrl Pts',(0.761858300014575,-1.,-1.96264672744229));
#22985=CARTESIAN_POINT('Ctrl Pts',(0.762447203806263,-1.,-1.95639665309893));
#22986=CARTESIAN_POINT('Ctrl Pts',(0.762992990878774,-1.,-1.95015342590025));
#22987=CARTESIAN_POINT('Ctrl Pts',(0.76349533353858,-1.,-1.94391746617626));
#22988=CARTESIAN_POINT('Ctrl Pts',(0.763954049121393,-1.,-1.93768964875867));
#22989=CARTESIAN_POINT('Ctrl Pts',(0.764369010673889,-1.,-1.93147105496367));
#22990=CARTESIAN_POINT('Ctrl Pts',(0.764740025488189,-1.,-1.92526263537041));
#22991=CARTESIAN_POINT('Ctrl Pts',(0.765066729667095,-1.,-1.91906491634197));
#22992=CARTESIAN_POINT('Ctrl Pts',(0.765348465884739,-1.,-1.91287765805174));
#22993=CARTESIAN_POINT('Ctrl Pts',(0.765584196937936,-1.,-1.90669961402362));
#22994=CARTESIAN_POINT('Ctrl Pts',(0.765772772593395,-1.,-1.90052930393599));
#22995=CARTESIAN_POINT('Ctrl Pts',(0.765913193856979,-1.,-1.89436577771389));
#22996=CARTESIAN_POINT('Ctrl Pts',(0.76600483706209,-1.,-1.88820926433409));
#22997=CARTESIAN_POINT('Ctrl Pts',(0.766047794851868,-1.,-1.88206215302561));
#22998=CARTESIAN_POINT('Ctrl Pts',(0.766042837036759,-1.,-1.87592888967886));
#22999=CARTESIAN_POINT('Ctrl Pts',(0.765990708546111,-1.,-1.86981398314345));
#23000=CARTESIAN_POINT('Ctrl Pts',(0.765891519092557,-1.,-1.86372027063315));
#23001=CARTESIAN_POINT('Ctrl Pts',(0.765744212909305,-1.,-1.85764741390391));
#23002=CARTESIAN_POINT('Ctrl Pts',(0.765545710619023,-1.,-1.85158945130054));
#23003=CARTESIAN_POINT('Ctrl Pts',(0.765291664861971,-1.,-1.84553698875911));
#23004=CARTESIAN_POINT('Ctrl Pts',(0.764978057881687,-1.,-1.83948181064823));
#23005=CARTESIAN_POINT('Ctrl Pts',(0.764602549687845,-1.,-1.8334207722714));
#23006=CARTESIAN_POINT('Ctrl Pts',(0.764165902606055,-1.,-1.8273599120008));
#23007=CARTESIAN_POINT('Ctrl Pts',(0.763673465462854,-1.,-1.82131873145297));
#23008=CARTESIAN_POINT('Ctrl Pts',(0.763132003836783,-1.,-1.81532118405566));
#23009=CARTESIAN_POINT('Ctrl Pts',(0.762546129464036,-1.,-1.80938551463989));
#23010=CARTESIAN_POINT('Ctrl Pts',(0.761915336443515,-1.,-1.80351583877334));
#23011=CARTESIAN_POINT('Ctrl Pts',(0.761229695230359,-1.,-1.79768986997735));
#23012=CARTESIAN_POINT('Ctrl Pts',(0.760469555880425,-1.,-1.79185815610802));
#23013=CARTESIAN_POINT('Ctrl Pts',(0.759614401109868,-1.,-1.78596964884527));
#23014=CARTESIAN_POINT('Ctrl Pts',(0.75865062667738,-1.,-1.77999411220912));
#23015=CARTESIAN_POINT('Ctrl Pts',(0.757578264077238,-1.,-1.77394167108342));
#23016=CARTESIAN_POINT('Ctrl Pts',(0.756421896028403,-1.,-1.76789396003141));
#23017=CARTESIAN_POINT('Ctrl Pts',(0.755220979975262,-1.,-1.7619781724032));
#23018=CARTESIAN_POINT('Ctrl Pts',(0.75400925402848,-1.,-1.75631083600175));
#23019=CARTESIAN_POINT('Ctrl Pts',(0.752797683531377,-1.,-1.75095139468809));
#23020=CARTESIAN_POINT('Ctrl Pts',(0.751555614163629,-1.,-1.74585086852298));
#23021=CARTESIAN_POINT('Ctrl Pts',(0.75019343597954,-1.,-1.74080458266705));
#23022=CARTESIAN_POINT('Ctrl Pts',(0.748582462954854,-1.,-1.73550351679848));
#23023=CARTESIAN_POINT('Ctrl Pts',(0.746574710096436,-1.,-1.72958533647399));
#23024=CARTESIAN_POINT('Ctrl Pts',(0.744021445433764,-1.,-1.7226822991693));
#23025=CARTESIAN_POINT('Ctrl Pts',(0.740795162032087,-1.,-1.71447789751927));
#23026=CARTESIAN_POINT('Ctrl Pts',(0.736799665724771,-1.,-1.70473309006121));
#23027=CARTESIAN_POINT('Ctrl Pts',(0.731963238697195,-1.,-1.69326921975743));
#23028=CARTESIAN_POINT('Ctrl Pts',(0.726235967997433,-1.,-1.67996158455503));
#23029=CARTESIAN_POINT('Ctrl Pts',(0.719585433804282,-1.,-1.6647288055568));
#23030=CARTESIAN_POINT('Ctrl Pts',(0.711993139355394,-1.,-1.64752408832016));
#23031=CARTESIAN_POINT('Ctrl Pts',(0.705159151988319,-1.,-1.63216541664676));
#23032=CARTESIAN_POINT('Ctrl Pts',(0.699605146405088,-1.,-1.61974673472612));
#23033=CARTESIAN_POINT('Ctrl Pts',(0.695712097881194,-1.,-1.61106790958151));
#23034=CARTESIAN_POINT('Ctrl Pts',(0.693717979106306,-1.,-1.60662857109684));
#23035=CARTESIAN_POINT('',(0.892032620296855,-1.,-1.5055822144029));
#23036=CARTESIAN_POINT('Origin',(0.,-1.,0.));
#23037=CARTESIAN_POINT('',(1.23627494547115,-1.,-1.81978687191668));
#23038=CARTESIAN_POINT('Ctrl Pts',(0.892032620296855,-1.,-1.5055822144029));
#23039=CARTESIAN_POINT('Ctrl Pts',(0.894452006964543,-1.,-1.50980486806688));
#23040=CARTESIAN_POINT('Ctrl Pts',(0.89918504748351,-1.,-1.51805569590094));
#23041=CARTESIAN_POINT('Ctrl Pts',(0.905967409625651,-1.,-1.52984849887993));
#23042=CARTESIAN_POINT('Ctrl Pts',(0.914375919026456,-1.,-1.54440491149498));
#23043=CARTESIAN_POINT('Ctrl Pts',(0.923832188944341,-1.,-1.56065988578893));
#23044=CARTESIAN_POINT('Ctrl Pts',(0.932246680108685,-1.,-1.57499388382243));
#23045=CARTESIAN_POINT('Ctrl Pts',(0.939646377893399,-1.,-1.58744937487176));
#23046=CARTESIAN_POINT('Ctrl Pts',(0.946078063315257,-1.,-1.59810042043673));
#23047=CARTESIAN_POINT('Ctrl Pts',(0.951613284356035,-1.,-1.60706069896936));
#23048=CARTESIAN_POINT('Ctrl Pts',(0.95635442292067,-1.,-1.61449324337085));
#23049=CARTESIAN_POINT('Ctrl Pts',(0.960438326101728,-1.,-1.62061638140221));
#23050=CARTESIAN_POINT('Ctrl Pts',(0.964046107040535,-1.,-1.62571930670187));
#23051=CARTESIAN_POINT('Ctrl Pts',(0.967387853230345,-1.,-1.63013849959462));
#23052=CARTESIAN_POINT('Ctrl Pts',(0.970669715997509,-1.,-1.63420665729798));
#23053=CARTESIAN_POINT('Ctrl Pts',(0.974066058287418,-1.,-1.63820952658144));
#23054=CARTESIAN_POINT('Ctrl Pts',(0.977689794119416,-1.,-1.64233990826687));
#23055=CARTESIAN_POINT('Ctrl Pts',(0.981562530939489,-1.,-1.64665139190656));
#23056=CARTESIAN_POINT('Ctrl Pts',(0.98564262292082,-1.,-1.65110016612638));
#23057=CARTESIAN_POINT('Ctrl Pts',(0.989855627854164,-1.,-1.65559044289699));
#23058=CARTESIAN_POINT('Ctrl Pts',(0.994121836661305,-1.,-1.66001553809947));
#23059=CARTESIAN_POINT('Ctrl Pts',(0.998389654952757,-1.,-1.66430758030376));
#23060=CARTESIAN_POINT('Ctrl Pts',(1.00265091003727,-1.,-1.66846059277303));
#23061=CARTESIAN_POINT('Ctrl Pts',(1.00692206696414,-1.,-1.67250335383293));
#23062=CARTESIAN_POINT('Ctrl Pts',(1.01123236493511,-1.,-1.67648246776464));
#23063=CARTESIAN_POINT('Ctrl Pts',(1.01561026162773,-1.,-1.68044289894798));
#23064=CARTESIAN_POINT('Ctrl Pts',(1.02006795074201,-1.,-1.68440578021706));
#23065=CARTESIAN_POINT('Ctrl Pts',(1.02460180535255,-1.,-1.68836910178447));
#23066=CARTESIAN_POINT('Ctrl Pts',(1.02919977579147,-1.,-1.69231840863458));
#23067=CARTESIAN_POINT('Ctrl Pts',(1.03384646003588,-1.,-1.69623414782771));
#23068=CARTESIAN_POINT('Ctrl Pts',(1.03852922490789,-1.,-1.70010052930962));
#23069=CARTESIAN_POINT('Ctrl Pts',(1.04324363334554,-1.,-1.70391338707982));
#23070=CARTESIAN_POINT('Ctrl Pts',(1.04799085404995,-1.,-1.70767646263649));
#23071=CARTESIAN_POINT('Ctrl Pts',(1.05277517202855,-1.,-1.71139783543989));
#23072=CARTESIAN_POINT('Ctrl Pts',(1.05760163192479,-1.,-1.7150865442702));
#23073=CARTESIAN_POINT('Ctrl Pts',(1.06247324680647,-1.,-1.71874858456904));
#23074=CARTESIAN_POINT('Ctrl Pts',(1.06738966975462,-1.,-1.72238500928453));
#23075=CARTESIAN_POINT('Ctrl Pts',(1.07234866990252,-1.,-1.72599406198488));
#23076=CARTESIAN_POINT('Ctrl Pts',(1.0773470373727,-1.,-1.72957248977424));
#23077=CARTESIAN_POINT('Ctrl Pts',(1.08238162784749,-1.,-1.73311705663407));
#23078=CARTESIAN_POINT('Ctrl Pts',(1.08745056285427,-1.,-1.73662628326091));
#23079=CARTESIAN_POINT('Ctrl Pts',(1.09255329056493,-1.,-1.74010053962247));
#23080=CARTESIAN_POINT('Ctrl Pts',(1.09768999241225,-1.,-1.74354119236208));
#23081=CARTESIAN_POINT('Ctrl Pts',(1.10286118991143,-1.,-1.74695004214923));
#23082=CARTESIAN_POINT('Ctrl Pts',(1.10806728183007,-1.,-1.7503286607592));
#23083=CARTESIAN_POINT('Ctrl Pts',(1.11330807582551,-1.,-1.7536777209463));
#23084=CARTESIAN_POINT('Ctrl Pts',(1.11858293216763,-1.,-1.75699720772105));
#23085=CARTESIAN_POINT('Ctrl Pts',(1.12389096855086,-1.,-1.76028671825096));
#23086=CARTESIAN_POINT('Ctrl Pts',(1.12923123555075,-1.,-1.7635457196617));
#23087=CARTESIAN_POINT('Ctrl Pts',(1.1346029180462,-1.,-1.76677384551862));
#23088=CARTESIAN_POINT('Ctrl Pts',(1.14000548336975,-1.,-1.76997111386769));
#23089=CARTESIAN_POINT('Ctrl Pts',(1.1454385822692,-1.,-1.77313777896194));
#23090=CARTESIAN_POINT('Ctrl Pts',(1.15090197841514,-1.,-1.7762742255701));
#23091=CARTESIAN_POINT('Ctrl Pts',(1.15639547194698,-1.,-1.77938085564275));
#23092=CARTESIAN_POINT('Ctrl Pts',(1.16191881298499,-1.,-1.78245795881009));
#23093=CARTESIAN_POINT('Ctrl Pts',(1.16747166312303,-1.,-1.78550566040443));
#23094=CARTESIAN_POINT('Ctrl Pts',(1.17305363177328,-1.,-1.78852398877617));
#23095=CARTESIAN_POINT('Ctrl Pts',(1.17866429440809,-1.,-1.79151291552689));
#23096=CARTESIAN_POINT('Ctrl Pts',(1.18430321697432,-1.,-1.79447240321515));
#23097=CARTESIAN_POINT('Ctrl Pts',(1.18996997934445,-1.,-1.79740245923478));
#23098=CARTESIAN_POINT('Ctrl Pts',(1.19566418930242,-1.,-1.80030314369879));
#23099=CARTESIAN_POINT('Ctrl Pts',(1.20138548938974,-1.,-1.80317454838603));
#23100=CARTESIAN_POINT('Ctrl Pts',(1.20713356605475,-1.,-1.80601678480707));
#23101=CARTESIAN_POINT('Ctrl Pts',(1.21290815708314,-1.,-1.80882996917129));
#23102=CARTESIAN_POINT('Ctrl Pts',(1.21870906103557,-1.,-1.81161420806656));
#23103=CARTESIAN_POINT('Ctrl Pts',(1.2245361330495,-1.,-1.81436959210434));
#23104=CARTESIAN_POINT('Ctrl Pts',(1.2292186489137,-1.,-1.8165508718364));
#23105=CARTESIAN_POINT('Ctrl Pts',(1.2327422452705,-1.,-1.81817389921279));
#23106=CARTESIAN_POINT('Ctrl Pts',(1.23509651170476,-1.,-1.81925017193666));
#23107=CARTESIAN_POINT('Ctrl Pts',(1.23627494547115,-1.,-1.81978687191668));
#23108=CARTESIAN_POINT('',(1.34869019493419,-1.,-1.73811241238545));
#23109=CARTESIAN_POINT('',(1.23627494547115,-1.,-1.81978687191668));
#23110=CARTESIAN_POINT('',(1.15624053661742,-1.,-1.31362392696032));
#23111=CARTESIAN_POINT('Ctrl Pts',(1.34869019493419,-1.,-1.73811241238545));
#23112=CARTESIAN_POINT('Ctrl Pts',(1.34854391898045,-1.,-1.73682580585691));
#23113=CARTESIAN_POINT('Ctrl Pts',(1.34824783112887,-1.,-1.73425417885907));
#23114=CARTESIAN_POINT('Ctrl Pts',(1.34779309152035,-1.,-1.7304014965394));
#23115=CARTESIAN_POINT('Ctrl Pts',(1.34716554819527,-1.,-1.72527410680674));
#23116=CARTESIAN_POINT('Ctrl Pts',(1.34634568653227,-1.,-1.7188807715049));
#23117=CARTESIAN_POINT('Ctrl Pts',(1.34549029589416,-1.,-1.71250340686822));
#23118=CARTESIAN_POINT('Ctrl Pts',(1.34459924533831,-1.,-1.70614212266738));
#23119=CARTESIAN_POINT('Ctrl Pts',(1.34367237124483,-1.,-1.69979707754427));
#23120=CARTESIAN_POINT('Ctrl Pts',(1.34270948206319,-1.,-1.6934684849687));
#23121=CARTESIAN_POINT('Ctrl Pts',(1.341710374848,-1.,-1.68715660868764));
#23122=CARTESIAN_POINT('Ctrl Pts',(1.34067485185203,-1.,-1.68086176030362));
#23123=CARTESIAN_POINT('Ctrl Pts',(1.3396027347034,-1.,-1.67458429426086));
#23124=CARTESIAN_POINT('Ctrl Pts',(1.33849388654388,-1.,-1.66832460783989));
#23125=CARTESIAN_POINT('Ctrl Pts',(1.33734820885262,-1.,-1.66208312541983));
#23126=CARTESIAN_POINT('Ctrl Pts',(1.33616559745172,-1.,-1.65586025952593));
#23127=CARTESIAN_POINT('Ctrl Pts',(1.33494590467993,-1.,-1.6496563728683));
#23128=CARTESIAN_POINT('Ctrl Pts',(1.33368890676572,-1.,-1.6434717485603));
#23129=CARTESIAN_POINT('Ctrl Pts',(1.33239425103724,-1.,-1.63730653475089));
#23130=CARTESIAN_POINT('Ctrl Pts',(1.33106149345645,-1.,-1.63116079730923));
#23131=CARTESIAN_POINT('Ctrl Pts',(1.3296901950568,-1.,-1.62503464209797));
#23132=CARTESIAN_POINT('Ctrl Pts',(1.32828000610449,-1.,-1.61892832270724));
#23133=CARTESIAN_POINT('Ctrl Pts',(1.32683074483356,-1.,-1.6128423401575));
#23134=CARTESIAN_POINT('Ctrl Pts',(1.32534250785782,-1.,-1.60677758290954));
#23135=CARTESIAN_POINT('Ctrl Pts',(1.32381550858256,-1.,-1.60073511858687));
#23136=CARTESIAN_POINT('Ctrl Pts',(1.32224985747682,-1.,-1.59471591079403));
#23137=CARTESIAN_POINT('Ctrl Pts',(1.32064537110892,-1.,-1.58872057258245));
#23138=CARTESIAN_POINT('Ctrl Pts',(1.31900135021432,-1.,-1.58274907898834));
#23139=CARTESIAN_POINT('Ctrl Pts',(1.31731642317187,-1.,-1.5768005650559));
#23140=CARTESIAN_POINT('Ctrl Pts',(1.31558903860016,-1.,-1.57087397835723));
#23141=CARTESIAN_POINT('Ctrl Pts',(1.31381795281002,-1.,-1.56496872402353));
#23142=CARTESIAN_POINT('Ctrl Pts',(1.31200264341696,-1.,-1.55908521254821));
#23143=CARTESIAN_POINT('Ctrl Pts',(1.31014393684222,-1.,-1.55322568759481));
#23144=CARTESIAN_POINT('Ctrl Pts',(1.30824393907473,-1.,-1.54739413957185));
#23145=CARTESIAN_POINT('Ctrl Pts',(1.30630475189556,-1.,-1.54159462645432));
#23146=CARTESIAN_POINT('Ctrl Pts',(1.30432735639489,-1.,-1.53582981268977));
#23147=CARTESIAN_POINT('Ctrl Pts',(1.30231064395568,-1.,-1.53009970283891));
#23148=CARTESIAN_POINT('Ctrl Pts',(1.30024984366328,-1.,-1.52439957861062));
#23149=CARTESIAN_POINT('Ctrl Pts',(1.29813791800747,-1.,-1.51872184912724));
#23150=CARTESIAN_POINT('Ctrl Pts',(1.29596850710509,-1.,-1.51305994241402));
#23151=CARTESIAN_POINT('Ctrl Pts',(1.29373841372842,-1.,-1.50741159078365));
#23152=CARTESIAN_POINT('Ctrl Pts',(1.29145022885181,-1.,-1.50178230149776));
#23153=CARTESIAN_POINT('Ctrl Pts',(1.28911506584254,-1.,-1.49618896881754));
#23154=CARTESIAN_POINT('Ctrl Pts',(1.2867467611644,-1.,-1.4906522831278));
#23155=CARTESIAN_POINT('Ctrl Pts',(1.28435533880201,-1.,-1.4851881711891));
#23156=CARTESIAN_POINT('Ctrl Pts',(1.28194158939517,-1.,-1.47980070347096));
#23157=CARTESIAN_POINT('Ctrl Pts',(1.2794891824849,-1.,-1.4744717526707));
#23158=CARTESIAN_POINT('Ctrl Pts',(1.27696414831089,-1.,-1.46916035917133));
#23159=CARTESIAN_POINT('Ctrl Pts',(1.27433119897822,-1.,-1.46382431332476));
#23160=CARTESIAN_POINT('Ctrl Pts',(1.27156805265289,-1.,-1.45843906294697));
#23161=CARTESIAN_POINT('Ctrl Pts',(1.2686778680489,-1.,-1.45301422764247));
#23162=CARTESIAN_POINT('Ctrl Pts',(1.26570925118868,-1.,-1.44761985001662));
#23163=CARTESIAN_POINT('Ctrl Pts',(1.26273903323858,-1.,-1.44236470511303));
#23164=CARTESIAN_POINT('Ctrl Pts',(1.25983531012005,-1.,-1.43734919180848));
#23165=CARTESIAN_POINT('Ctrl Pts',(1.25702687965755,-1.,-1.43262645609691));
#23166=CARTESIAN_POINT('Ctrl Pts',(1.25426945222639,-1.,-1.42815938799387));
#23167=CARTESIAN_POINT('Ctrl Pts',(1.2514145557001,-1.,-1.42378102115575));
#23168=CARTESIAN_POINT('Ctrl Pts',(1.24824430986571,-1.,-1.41923722596025));
#23169=CARTESIAN_POINT('Ctrl Pts',(1.24450600513056,-1.,-1.41422913175179));
#23170=CARTESIAN_POINT('Ctrl Pts',(1.23994455029534,-1.,-1.40845295531283));
#23171=CARTESIAN_POINT('Ctrl Pts',(1.23434087290423,-1.,-1.40164708206106));
#23172=CARTESIAN_POINT('Ctrl Pts',(1.22752961899387,-1.,-1.39361389568796));
#23173=CARTESIAN_POINT('Ctrl Pts',(1.21938737280852,-1.,-1.38420564527715));
#23174=CARTESIAN_POINT('Ctrl Pts',(1.20982812925645,-1.,-1.37331915607905));
#23175=CARTESIAN_POINT('Ctrl Pts',(1.1987959077932,-1.,-1.36088705043885));
#23176=CARTESIAN_POINT('Ctrl Pts',(1.18625865667441,-1.,-1.34687054001093));
#23177=CARTESIAN_POINT('Ctrl Pts',(1.17501305789857,-1.,-1.33437539347008));
#23178=CARTESIAN_POINT('Ctrl Pts',(1.16589330093588,-1.,-1.32428080721772));
#23179=CARTESIAN_POINT('Ctrl Pts',(1.15950888730809,-1.,-1.31722977216397));
#23180=CARTESIAN_POINT('Ctrl Pts',(1.15624053661742,-1.,-1.31362392696032));
#23181=CARTESIAN_POINT('',(1.31362392696032,-1.,-1.15624053661742));
#23182=CARTESIAN_POINT('Origin',(0.,-1.,0.));
#23183=CARTESIAN_POINT('',(1.73811241238545,-1.,-1.34869019493419));
#23184=CARTESIAN_POINT('Ctrl Pts',(1.31362392696032,-1.,-1.15624053661742));
#23185=CARTESIAN_POINT('Ctrl Pts',(1.3172297721596,-1.,-1.15950888730433));
#23186=CARTESIAN_POINT('Ctrl Pts',(1.32428080720544,-1.,-1.16589330092532));
#23187=CARTESIAN_POINT('Ctrl Pts',(1.33437539344842,-1.,-1.17501305787994));
#23188=CARTESIAN_POINT('Ctrl Pts',(1.34687053998157,-1.,-1.18625865664915));
#23189=CARTESIAN_POINT('Ctrl Pts',(1.36088705040677,-1.,-1.1987959077656));
#23190=CARTESIAN_POINT('Ctrl Pts',(1.37331915604962,-1.,-1.20982812923113));
#23191=CARTESIAN_POINT('Ctrl Pts',(1.38420564525391,-1.,-1.21938737278853));
#23192=CARTESIAN_POINT('Ctrl Pts',(1.39361389567257,-1.,-1.22752961898063));
#23193=CARTESIAN_POINT('Ctrl Pts',(1.40164708205345,-1.,-1.23434087289768));
#23194=CARTESIAN_POINT('Ctrl Pts',(1.40845295531151,-1.,-1.23994455029421));
#23195=CARTESIAN_POINT('Ctrl Pts',(1.41422913175437,-1.,-1.24450600513278));
#23196=CARTESIAN_POINT('Ctrl Pts',(1.41923722596421,-1.,-1.24824430986911));
#23197=CARTESIAN_POINT('Ctrl Pts',(1.42378102115911,-1.,-1.25141455570299));
#23198=CARTESIAN_POINT('Ctrl Pts',(1.42815938799555,-1.,-1.25426945222783));
#23199=CARTESIAN_POINT('Ctrl Pts',(1.43262645609679,-1.,-1.25702687965744));
#23200=CARTESIAN_POINT('Ctrl Pts',(1.43734919180719,-1.,-1.25983531011894));
#23201=CARTESIAN_POINT('Ctrl Pts',(1.44236470511145,-1.,-1.26273903323723));
#23202=CARTESIAN_POINT('Ctrl Pts',(1.44761985001544,-1.,-1.26570925118767));
#23203=CARTESIAN_POINT('Ctrl Pts',(1.45301422764205,-1.,-1.26867786804854));
#23204=CARTESIAN_POINT('Ctrl Pts',(1.45843906294725,-1.,-1.27156805265312));
#23205=CARTESIAN_POINT('Ctrl Pts',(1.4638243133254,-1.,-1.27433119897877));
#23206=CARTESIAN_POINT('Ctrl Pts',(1.46916035917197,-1.,-1.27696414831144));
#23207=CARTESIAN_POINT('Ctrl Pts',(1.4744717526711,-1.,-1.27948918248524));
#23208=CARTESIAN_POINT('Ctrl Pts',(1.47980070347102,-1.,-1.28194158939522));
#23209=CARTESIAN_POINT('Ctrl Pts',(1.48518817118891,-1.,-1.28435533880184));
#23210=CARTESIAN_POINT('Ctrl Pts',(1.4906522831275,-1.,-1.28674676116415));
#23211=CARTESIAN_POINT('Ctrl Pts',(1.49618896881729,-1.,-1.28911506584232));
#23212=CARTESIAN_POINT('Ctrl Pts',(1.50178230149764,-1.,-1.29145022885171));
#23213=CARTESIAN_POINT('Ctrl Pts',(1.50741159078367,-1.,-1.29373841372843));
#23214=CARTESIAN_POINT('Ctrl Pts',(1.51305994241412,-1.,-1.29596850710518));
#23215=CARTESIAN_POINT('Ctrl Pts',(1.51872184912735,-1.,-1.29813791800757));
#23216=CARTESIAN_POINT('Ctrl Pts',(1.5243995786107,-1.,-1.30024984366334));
#23217=CARTESIAN_POINT('Ctrl Pts',(1.53009970283893,-1.,-1.3023106439557));
#23218=CARTESIAN_POINT('Ctrl Pts',(1.53582981268976,-1.,-1.30432735639487));
#23219=CARTESIAN_POINT('Ctrl Pts',(1.54159462645428,-1.,-1.30630475189553));
#23220=CARTESIAN_POINT('Ctrl Pts',(1.54739413957183,-1.,-1.30824393907471));
#23221=CARTESIAN_POINT('Ctrl Pts',(1.55322568759481,-1.,-1.31014393684221));
#23222=CARTESIAN_POINT('Ctrl Pts',(1.55908521254822,-1.,-1.31200264341696));
#23223=CARTESIAN_POINT('Ctrl Pts',(1.56496872402352,-1.,-1.31381795281002));
#23224=CARTESIAN_POINT('Ctrl Pts',(1.57087397835721,-1.,-1.31558903860015));
#23225=CARTESIAN_POINT('Ctrl Pts',(1.57680056505585,-1.,-1.31731642317183));
#23226=CARTESIAN_POINT('Ctrl Pts',(1.58274907898829,-1.,-1.31900135021428));
#23227=CARTESIAN_POINT('Ctrl Pts',(1.58872057258244,-1.,-1.32064537110891));
#23228=CARTESIAN_POINT('Ctrl Pts',(1.59471591079408,-1.,-1.32224985747686));
#23229=CARTESIAN_POINT('Ctrl Pts',(1.600735118587,-1.,-1.32381550858266));
#23230=CARTESIAN_POINT('Ctrl Pts',(1.6067775829097,-1.,-1.32534250785794));
#23231=CARTESIAN_POINT('Ctrl Pts',(1.61284234015762,-1.,-1.32683074483365));
#23232=CARTESIAN_POINT('Ctrl Pts',(1.61892832270723,-1.,-1.32828000610448));
#23233=CARTESIAN_POINT('Ctrl Pts',(1.62503464209777,-1.,-1.32969019505665));
#23234=CARTESIAN_POINT('Ctrl Pts',(1.63116079730887,-1.,-1.33106149345618));
#23235=CARTESIAN_POINT('Ctrl Pts',(1.63730653475049,-1.,-1.33239425103694));
#23236=CARTESIAN_POINT('Ctrl Pts',(1.64347174856007,-1.,-1.33368890676554));
#23237=CARTESIAN_POINT('Ctrl Pts',(1.64965637286843,-1.,-1.33494590468003));
#23238=CARTESIAN_POINT('Ctrl Pts',(1.65586025952651,-1.,-1.33616559745217));
#23239=CARTESIAN_POINT('Ctrl Pts',(1.66208312542073,-1.,-1.33734820885331));
#23240=CARTESIAN_POINT('Ctrl Pts',(1.66832460784078,-1.,-1.33849388654458));
#23241=CARTESIAN_POINT('Ctrl Pts',(1.67458429426126,-1.,-1.33960273470372));
#23242=CARTESIAN_POINT('Ctrl Pts',(1.68086176030308,-1.,-1.3406748518516));
#23243=CARTESIAN_POINT('Ctrl Pts',(1.68715660868602,-1.,-1.34171037484673));
#23244=CARTESIAN_POINT('Ctrl Pts',(1.6934684849664,-1.,-1.34270948206139));
#23245=CARTESIAN_POINT('Ctrl Pts',(1.69979707754221,-1.,-1.34367237124322));
#23246=CARTESIAN_POINT('Ctrl Pts',(1.70614212266676,-1.,-1.34459924533783));
#23247=CARTESIAN_POINT('Ctrl Pts',(1.71250340687011,-1.,-1.34549029589563));
#23248=CARTESIAN_POINT('Ctrl Pts',(1.7188807715095,-1.,-1.34634568653586));
#23249=CARTESIAN_POINT('Ctrl Pts',(1.72527410681298,-1.,-1.34716554820013));
#23250=CARTESIAN_POINT('Ctrl Pts',(1.73040149654497,-1.,-1.3477930915247));
#23251=CARTESIAN_POINT('Ctrl Pts',(1.73425417886254,-1.,-1.34824783113158));
#23252=CARTESIAN_POINT('Ctrl Pts',(1.73682580585819,-1.,-1.34854391898145));
#23253=CARTESIAN_POINT('Ctrl Pts',(1.73811241238545,-1.,-1.34869019493419));
#23254=CARTESIAN_POINT('',(1.81978687191668,-1.,-1.23627494547115));
#23255=CARTESIAN_POINT('',(1.73811241238545,-1.,-1.34869019493419));
#23256=CARTESIAN_POINT('',(1.5055822144029,-1.,-0.892032620296855));
#23257=CARTESIAN_POINT('Ctrl Pts',(1.81978687191668,-1.,-1.23627494547115));
#23258=CARTESIAN_POINT('Ctrl Pts',(1.81925017193531,-1.,-1.23509651170384));
#23259=CARTESIAN_POINT('Ctrl Pts',(1.81817389920914,-1.,-1.23274224526804));
#23260=CARTESIAN_POINT('Ctrl Pts',(1.81655087183054,-1.,-1.22921864890975));
#23261=CARTESIAN_POINT('Ctrl Pts',(1.81436959209778,-1.,-1.22453613304507));
#23262=CARTESIAN_POINT('Ctrl Pts',(1.81161420806172,-1.,-1.2187090610323));
#23263=CARTESIAN_POINT('Ctrl Pts',(1.80882996916931,-1.,-1.2129081570818));
#23264=CARTESIAN_POINT('Ctrl Pts',(1.80601678480772,-1.,-1.20713356605519));
#23265=CARTESIAN_POINT('Ctrl Pts',(1.8031745483882,-1.,-1.2013854893912));
#23266=CARTESIAN_POINT('Ctrl Pts',(1.80030314370121,-1.,-1.19566418930405));
#23267=CARTESIAN_POINT('Ctrl Pts',(1.79740245923649,-1.,-1.1899699793456));
#23268=CARTESIAN_POINT('Ctrl Pts',(1.79447240321572,-1.,-1.18430321697471));
#23269=CARTESIAN_POINT('Ctrl Pts',(1.79151291552646,-1.,-1.17866429440781));
#23270=CARTESIAN_POINT('Ctrl Pts',(1.78852398877523,-1.,-1.17305363177265));
#23271=CARTESIAN_POINT('Ctrl Pts',(1.78550566040349,-1.,-1.16747166312239));
#23272=CARTESIAN_POINT('Ctrl Pts',(1.78245795880949,-1.,-1.16191881298458));
#23273=CARTESIAN_POINT('Ctrl Pts',(1.77938085564261,-1.,-1.15639547194689));
#23274=CARTESIAN_POINT('Ctrl Pts',(1.77627422557034,-1.,-1.15090197841531));
#23275=CARTESIAN_POINT('Ctrl Pts',(1.77313777896234,-1.,-1.14543858226948));
#23276=CARTESIAN_POINT('Ctrl Pts',(1.76997111386806,-1.,-1.14000548337));
#23277=CARTESIAN_POINT('Ctrl Pts',(1.76677384551883,-1.,-1.13460291804635));
#23278=CARTESIAN_POINT('Ctrl Pts',(1.76354571966171,-1.,-1.12923123555076));
#23279=CARTESIAN_POINT('Ctrl Pts',(1.76028671825084,-1.,-1.12389096855078));
#23280=CARTESIAN_POINT('Ctrl Pts',(1.75699720772089,-1.,-1.11858293216752));
#23281=CARTESIAN_POINT('Ctrl Pts',(1.75367772094617,-1.,-1.11330807582542));
#23282=CARTESIAN_POINT('Ctrl Pts',(1.75032866075914,-1.,-1.10806728183003));
#23283=CARTESIAN_POINT('Ctrl Pts',(1.74695004214924,-1.,-1.10286118991144));
#23284=CARTESIAN_POINT('Ctrl Pts',(1.74354119236212,-1.,-1.09768999241229));
#23285=CARTESIAN_POINT('Ctrl Pts',(1.74010053962252,-1.,-1.09255329056496));
#23286=CARTESIAN_POINT('Ctrl Pts',(1.73662628326093,-1.,-1.08745056285429));
#23287=CARTESIAN_POINT('Ctrl Pts',(1.73311705663407,-1.,-1.08238162784749));
#23288=CARTESIAN_POINT('Ctrl Pts',(1.72957248977424,-1.,-1.0773470373727));
#23289=CARTESIAN_POINT('Ctrl Pts',(1.72599406198489,-1.,-1.07234866990252));
#23290=CARTESIAN_POINT('Ctrl Pts',(1.72238500928456,-1.,-1.06738966975463));
#23291=CARTESIAN_POINT('Ctrl Pts',(1.71874858456908,-1.,-1.0624732468065));
#23292=CARTESIAN_POINT('Ctrl Pts',(1.71508654427022,-1.,-1.05760163192481));
#23293=CARTESIAN_POINT('Ctrl Pts',(1.71139783543986,-1.,-1.05277517202854));
#23294=CARTESIAN_POINT('Ctrl Pts',(1.70767646263641,-1.,-1.0479908540499));
#23295=CARTESIAN_POINT('Ctrl Pts',(1.70391338707969,-1.,-1.04324363334546));
#23296=CARTESIAN_POINT('Ctrl Pts',(1.70010052930951,-1.,-1.03852922490782));
#23297=CARTESIAN_POINT('Ctrl Pts',(1.69623414782769,-1.,-1.03384646003587));
#23298=CARTESIAN_POINT('Ctrl Pts',(1.69231840863471,-1.,-1.02919977579155));
#23299=CARTESIAN_POINT('Ctrl Pts',(1.68836910178475,-1.,-1.02460180535272));
#23300=CARTESIAN_POINT('Ctrl Pts',(1.68440578021739,-1.,-1.02006795074222));
#23301=CARTESIAN_POINT('Ctrl Pts',(1.6804428989482,-1.,-1.01561026162787));
#23302=CARTESIAN_POINT('Ctrl Pts',(1.67648246776457,-1.,-1.01123236493507));
#23303=CARTESIAN_POINT('Ctrl Pts',(1.67250335383248,-1.,-1.00692206696387));
#23304=CARTESIAN_POINT('Ctrl Pts',(1.66846059277231,-1.,-1.00265091003682));
#23305=CARTESIAN_POINT('Ctrl Pts',(1.66430758030304,-1.,-0.998389654952317));
#23306=CARTESIAN_POINT('Ctrl Pts',(1.66001553809916,-1.,-0.994121836661116));
#23307=CARTESIAN_POINT('Ctrl Pts',(1.65559044289746,-1.,-0.98985562785445));
#23308=CARTESIAN_POINT('Ctrl Pts',(1.6511001661277,-1.,-0.985642622921626));
#23309=CARTESIAN_POINT('Ctrl Pts',(1.64665139190834,-1.,-0.981562530940574));
#23310=CARTESIAN_POINT('Ctrl Pts',(1.64233990826831,-1.,-0.977689794120297));
#23311=CARTESIAN_POINT('Ctrl Pts',(1.63820952658157,-1.,-0.974066058287501));
#23312=CARTESIAN_POINT('Ctrl Pts',(1.63420665729609,-1.,-0.970669715996356));
#23313=CARTESIAN_POINT('Ctrl Pts',(1.63013849959083,-1.,-0.967387853228041));
#23314=CARTESIAN_POINT('Ctrl Pts',(1.6257193066974,-1.,-0.964046107037821));
#23315=CARTESIAN_POINT('Ctrl Pts',(1.62061638139929,-1.,-0.960438326099958));
#23316=CARTESIAN_POINT('Ctrl Pts',(1.61449324337233,-1.,-0.956354422921573));
#23317=CARTESIAN_POINT('Ctrl Pts',(1.60706069897794,-1.,-0.951613284361248));
#23318=CARTESIAN_POINT('Ctrl Pts',(1.59810042045408,-1.,-0.946078063325796));
#23319=CARTESIAN_POINT('Ctrl Pts',(1.58744937489796,-1.,-0.939646377909319));
#23320=CARTESIAN_POINT('Ctrl Pts',(1.57499388385561,-1.,-0.932246680128849));
#23321=CARTESIAN_POINT('Ctrl Pts',(1.56065988582509,-1.,-0.923832188966322));
#23322=CARTESIAN_POINT('Ctrl Pts',(1.54440491152807,-1.,-0.91437591904658));
#23323=CARTESIAN_POINT('Ctrl Pts',(1.52984849890434,-1.,-0.905967409640499));
#23324=CARTESIAN_POINT('Ctrl Pts',(1.51805569591479,-1.,-0.89918504749193));
#23325=CARTESIAN_POINT('Ctrl Pts',(1.50980486807181,-1.,-0.894452006967538));
#23326=CARTESIAN_POINT('Ctrl Pts',(1.5055822144029,-1.,-0.892032620296855));
#23327=CARTESIAN_POINT('',(1.60662857109684,-1.,-0.693717979106306));
#23328=CARTESIAN_POINT('Origin',(0.,-1.,0.));
#23329=CARTESIAN_POINT('',(2.0698113262342,-1.,-0.745574324794401));
#23330=CARTESIAN_POINT('Ctrl Pts',(1.60662857109684,-1.,-0.693717979106306));
#23331=CARTESIAN_POINT('Ctrl Pts',(1.61106790957619,-1.,-0.69571209787897));
#23332=CARTESIAN_POINT('Ctrl Pts',(1.61974673471117,-1.,-0.699605146398837));
#23333=CARTESIAN_POINT('Ctrl Pts',(1.6321654166204,-1.,-0.705159151977294));
#23334=CARTESIAN_POINT('Ctrl Pts',(1.64752408828442,-1.,-0.711993139340448));
#23335=CARTESIAN_POINT('Ctrl Pts',(1.66472880551777,-1.,-0.71958543378795));
#23336=CARTESIAN_POINT('Ctrl Pts',(1.67996158451922,-1.,-0.726235967982445));
#23337=CARTESIAN_POINT('Ctrl Pts',(1.69326921972915,-1.,-0.731963238685357));
#23338=CARTESIAN_POINT('Ctrl Pts',(1.70473309004249,-1.,-0.736799665716932));
#23339=CARTESIAN_POINT('Ctrl Pts',(1.71447789751001,-1.,-0.74079516202821));
#23340=CARTESIAN_POINT('Ctrl Pts',(1.72268229916769,-1.,-0.744021445433094));
#23341=CARTESIAN_POINT('Ctrl Pts',(1.72958533647714,-1.,-0.746574710097752));
#23342=CARTESIAN_POINT('Ctrl Pts',(1.7355035168033,-1.,-0.74858246295687));
#23343=CARTESIAN_POINT('Ctrl Pts',(1.74080458267114,-1.,-0.75019343598125));
#23344=CARTESIAN_POINT('Ctrl Pts',(1.74585086852502,-1.,-0.751555614164483));
#23345=CARTESIAN_POINT('Ctrl Pts',(1.75095139468794,-1.,-0.752797683531314));
#23346=CARTESIAN_POINT('Ctrl Pts',(1.75631083600019,-1.,-0.754009254027829));
#23347=CARTESIAN_POINT('Ctrl Pts',(1.76197817240128,-1.,-0.755220979974462));
#23348=CARTESIAN_POINT('Ctrl Pts',(1.76789396002998,-1.,-0.75642189602781));
#23349=CARTESIAN_POINT('Ctrl Pts',(1.77394167108292,-1.,-0.757578264077029));
#23350=CARTESIAN_POINT('Ctrl Pts',(1.77999411220945,-1.,-0.758650626677519));
#23351=CARTESIAN_POINT('Ctrl Pts',(1.78596964884604,-1.,-0.75961440111019));
#23352=CARTESIAN_POINT('Ctrl Pts',(1.7918581561088,-1.,-0.760469555880749));
#23353=CARTESIAN_POINT('Ctrl Pts',(1.79768986997783,-1.,-0.761229695230558));
#23354=CARTESIAN_POINT('Ctrl Pts',(1.80351583877342,-1.,-0.761915336443547));
#23355=CARTESIAN_POINT('Ctrl Pts',(1.80938551463965,-1.,-0.762546129463938));
#23356=CARTESIAN_POINT('Ctrl Pts',(1.8153211840553,-1.,-0.763132003836634));
#23357=CARTESIAN_POINT('Ctrl Pts',(1.82131873145266,-1.,-0.763673465462727));
#23358=CARTESIAN_POINT('Ctrl Pts',(1.82735991200065,-1.,-0.764165902605995));
#23359=CARTESIAN_POINT('Ctrl Pts',(1.83342077227142,-1.,-0.764602549687853));
#23360=CARTESIAN_POINT('Ctrl Pts',(1.83948181064835,-1.,-0.764978057881738));
#23361=CARTESIAN_POINT('Ctrl Pts',(1.84553698875924,-1.,-0.765291664862029));
#23362=CARTESIAN_POINT('Ctrl Pts',(1.85158945130063,-1.,-0.765545710619063));
#23363=CARTESIAN_POINT('Ctrl Pts',(1.85764741390394,-1.,-0.765744212909319));
#23364=CARTESIAN_POINT('Ctrl Pts',(1.86372027063312,-1.,-0.765891519092547));
#23365=CARTESIAN_POINT('Ctrl Pts',(1.86981398314341,-1.,-0.765990708546091));
#23366=CARTESIAN_POINT('Ctrl Pts',(1.87592888967883,-1.,-0.766042837036744));
#23367=CARTESIAN_POINT('Ctrl Pts',(1.88206215302561,-1.,-0.766047794851865));
#23368=CARTESIAN_POINT('Ctrl Pts',(1.88820926433409,-1.,-0.766004837062091));
#23369=CARTESIAN_POINT('Ctrl Pts',(1.89436577771388,-1.,-0.765913193856978));
#23370=CARTESIAN_POINT('Ctrl Pts',(1.90052930393596,-1.,-0.765772772593386));
#23371=CARTESIAN_POINT('Ctrl Pts',(1.90669961402356,-1.,-0.765584196937919));
#23372=CARTESIAN_POINT('Ctrl Pts',(1.91287765805169,-1.,-0.765348465884722));
#23373=CARTESIAN_POINT('Ctrl Pts',(1.91906491634196,-1.,-0.765066729667089));
#23374=CARTESIAN_POINT('Ctrl Pts',(1.92526263537048,-1.,-0.764740025488212));
#23375=CARTESIAN_POINT('Ctrl Pts',(1.93147105496382,-1.,-0.764369010673941));
#23376=CARTESIAN_POINT('Ctrl Pts',(1.93768964875886,-1.,-0.763954049121459));
#23377=CARTESIAN_POINT('Ctrl Pts',(1.9439174661764,-1.,-0.763495333538629));
#23378=CARTESIAN_POINT('Ctrl Pts',(1.95015342590024,-1.,-0.762992990878769));
#23379=CARTESIAN_POINT('Ctrl Pts',(1.95639665309869,-1.,-0.762447203806179));
#23380=CARTESIAN_POINT('Ctrl Pts',(1.96264672744186,-1.,-0.761858300014424));
#23381=CARTESIAN_POINT('Ctrl Pts',(1.96890351582499,-1.,-0.761226690483821));
#23382=CARTESIAN_POINT('Ctrl Pts',(1.97516705321494,-1.,-0.760552825409757));
#23383=CARTESIAN_POINT('Ctrl Pts',(1.98143741418172,-1.,-0.75983714745219));
#23384=CARTESIAN_POINT('Ctrl Pts',(1.98771456680874,-1.,-0.759080037802488));
#23385=CARTESIAN_POINT('Ctrl Pts',(1.99399831098817,-1.,-0.758281796766761));
#23386=CARTESIAN_POINT('Ctrl Pts',(2.00028834739178,-1.,-0.757442676862724));
#23387=CARTESIAN_POINT('Ctrl Pts',(2.0065843158773,-1.,-0.756562904646671));
#23388=CARTESIAN_POINT('Ctrl Pts',(2.01288584328084,-1.,-0.755642704957865));
#23389=CARTESIAN_POINT('Ctrl Pts',(2.01919259405809,-1.,-0.754682330722816));
#23390=CARTESIAN_POINT('Ctrl Pts',(2.02550428623313,-1.,-0.753682061112768));
#23391=CARTESIAN_POINT('Ctrl Pts',(2.03182068456221,-1.,-0.752642180487211));
#23392=CARTESIAN_POINT('Ctrl Pts',(2.03814160092099,-1.,-0.751562963361115));
#23393=CARTESIAN_POINT('Ctrl Pts',(2.04446689147979,-1.,-0.750444657875576));
#23394=CARTESIAN_POINT('Ctrl Pts',(2.05079645592154,-1.,-0.749287468665046));
#23395=CARTESIAN_POINT('Ctrl Pts',(2.05713023031006,-1.,-0.748091554183803));
#23396=CARTESIAN_POINT('Ctrl Pts',(2.06220058927826,-1.,-0.74710393278792));
#23397=CARTESIAN_POINT('Ctrl Pts',(2.06600523016815,-1.,-0.746345871544201));
#23398=CARTESIAN_POINT('Ctrl Pts',(2.06854248895728,-1.,-0.745832791378367));
#23399=CARTESIAN_POINT('Ctrl Pts',(2.0698113262342,-1.,-0.745574324794401));
#23400=CARTESIAN_POINT('',(2.11275013067528,-1.,-0.61342227326009));
#23401=CARTESIAN_POINT('',(2.0698113262342,-1.,-0.745574324794401));
#23402=CARTESIAN_POINT('',(1.7075470150345,-1.,-0.383122945602004));
#23403=CARTESIAN_POINT('Ctrl Pts',(2.11275013067528,-1.,-0.61342227326009));
#23404=CARTESIAN_POINT('Ctrl Pts',(2.11187554259986,-1.,-0.6124673655618));
#23405=CARTESIAN_POINT('Ctrl Pts',(2.11012443807238,-1.,-0.610560911689899));
#23406=CARTESIAN_POINT('Ctrl Pts',(2.1074919961518,-1.,-0.607711315454876));
#23407=CARTESIAN_POINT('Ctrl Pts',(2.10397049886949,-1.,-0.60393203073603));
#23408=CARTESIAN_POINT('Ctrl Pts',(2.0995493086477,-1.,-0.599241616420534));
#23409=CARTESIAN_POINT('Ctrl Pts',(2.0951087622027,-1.,-0.594585006052162));
#23410=CARTESIAN_POINT('Ctrl Pts',(2.09064881812129,-1.,-0.589962365403406));
#23411=CARTESIAN_POINT('Ctrl Pts',(2.08616943727951,-1.,-0.585373918991617));
#23412=CARTESIAN_POINT('Ctrl Pts',(2.08167059018418,-1.,-0.580819952108064));
#23413=CARTESIAN_POINT('Ctrl Pts',(2.07715226767559,-1.,-0.576300797416845));
#23414=CARTESIAN_POINT('Ctrl Pts',(2.07261449292824,-1.,-0.571816823242603));
#23415=CARTESIAN_POINT('Ctrl Pts',(2.06805732997334,-1.,-0.567368421181087));
#23416=CARTESIAN_POINT('Ctrl Pts',(2.06348090160589,-1.,-0.562955993082262));
#23417=CARTESIAN_POINT('Ctrl Pts',(2.05888537756462,-1.,-0.558579940185152));
#23418=CARTESIAN_POINT('Ctrl Pts',(2.05427091604413,-1.,-0.554240657463906));
#23419=CARTESIAN_POINT('Ctrl Pts',(2.04963761077958,-1.,-0.549938525150295));
#23420=CARTESIAN_POINT('Ctrl Pts',(2.04498544714588,-1.,-0.54567390381743));
#23421=CARTESIAN_POINT('Ctrl Pts',(2.04031422690527,-1.,-0.541447120615659));
#23422=CARTESIAN_POINT('Ctrl Pts',(2.03562362954037,-1.,-0.537258489833262));
#23423=CARTESIAN_POINT('Ctrl Pts',(2.03091336214426,-1.,-0.533108355132977));
#23424=CARTESIAN_POINT('Ctrl Pts',(2.0261832908329,-1.,-0.528997127241914));
#23425=CARTESIAN_POINT('Ctrl Pts',(2.02143356304698,-1.,-0.524925318333476));
#23426=CARTESIAN_POINT('Ctrl Pts',(2.01666477917286,-1.,-0.520893590399371));
#23427=CARTESIAN_POINT('Ctrl Pts',(2.01187773939242,-1.,-0.516902681728687));
#23428=CARTESIAN_POINT('Ctrl Pts',(2.00707309946949,-1.,-0.512953306961793));
#23429=CARTESIAN_POINT('Ctrl Pts',(2.00225107134734,-1.,-0.509046069886157));
#23430=CARTESIAN_POINT('Ctrl Pts',(1.99741107463572,-1.,-0.505181361323026));
#23431=CARTESIAN_POINT('Ctrl Pts',(1.99255149126155,-1.,-0.501359287727146));
#23432=CARTESIAN_POINT('Ctrl Pts',(1.98767044752932,-1.,-0.497579909545574));
#23433=CARTESIAN_POINT('Ctrl Pts',(1.98276658761821,-1.,-0.493843476541495));
#23434=CARTESIAN_POINT('Ctrl Pts',(1.97783973019229,-1.,-0.490150627860953));
#23435=CARTESIAN_POINT('Ctrl Pts',(1.97289186263272,-1.,-0.486502692907659));
#23436=CARTESIAN_POINT('Ctrl Pts',(1.96792703422362,-1.,-0.482901662120691));
#23437=CARTESIAN_POINT('Ctrl Pts',(1.96294933055943,-1.,-0.479349583074855));
#23438=CARTESIAN_POINT('Ctrl Pts',(1.95796111148177,-1.,-0.475848034683176));
#23439=CARTESIAN_POINT('Ctrl Pts',(1.95296148278133,-1.,-0.472397672264072));
#23440=CARTESIAN_POINT('Ctrl Pts',(1.94794381136514,-1.,-0.468997482913135));
#23441=CARTESIAN_POINT('Ctrl Pts',(1.9428979419619,-1.,-0.46564546202603));
#23442=CARTESIAN_POINT('Ctrl Pts',(1.93781486640821,-1.,-0.462340031009057));
#23443=CARTESIAN_POINT('Ctrl Pts',(1.93269066517934,-1.,-0.459081234547926));
#23444=CARTESIAN_POINT('Ctrl Pts',(1.92753067150476,-1.,-0.455872005174371));
#23445=CARTESIAN_POINT('Ctrl Pts',(1.92235380648502,-1.,-0.452719478359433));
#23446=CARTESIAN_POINT('Ctrl Pts',(1.91718342555755,-1.,-0.449632260106662));
#23447=CARTESIAN_POINT('Ctrl Pts',(1.9120369998112,-1.,-0.446617343485711));
#23448=CARTESIAN_POINT('Ctrl Pts',(1.90691756144898,-1.,-0.443677556849151));
#23449=CARTESIAN_POINT('Ctrl Pts',(1.90180124389086,-1.,-0.440807833704038));
#23450=CARTESIAN_POINT('Ctrl Pts',(1.89663648956466,-1.,-0.437995003948244));
#23451=CARTESIAN_POINT('Ctrl Pts',(1.89136993975504,-1.,-0.435225660963383));
#23452=CARTESIAN_POINT('Ctrl Pts',(1.88596913666793,-1.,-0.432493038548748));
#23453=CARTESIAN_POINT('Ctrl Pts',(1.88044229001832,-1.,-0.429803062482345));
#23454=CARTESIAN_POINT('Ctrl Pts',(1.87486989291484,-1.,-0.427183828519102));
#23455=CARTESIAN_POINT('Ctrl Pts',(1.86937803944323,-1.,-0.424678177291359));
#23456=CARTESIAN_POINT('Ctrl Pts',(1.86408083334028,-1.,-0.422327307418275));
#23457=CARTESIAN_POINT('Ctrl Pts',(1.85903281096686,-1.,-0.42015728797562));
#23458=CARTESIAN_POINT('Ctrl Pts',(1.85417632856234,-1.,-0.418164129143534));
#23459=CARTESIAN_POINT('Ctrl Pts',(1.84929312929882,-1.,-0.416300022038864));
#23460=CARTESIAN_POINT('Ctrl Pts',(1.8440575707371,-1.,-0.41448743825434));
#23461=CARTESIAN_POINT('Ctrl Pts',(1.83808953475839,-1.,-0.412633125322162));
#23462=CARTESIAN_POINT('Ctrl Pts',(1.83100408895216,-1.,-0.410641256301675));
#23463=CARTESIAN_POINT('Ctrl Pts',(1.8224702267854,-1.,-0.408428948108534));
#23464=CARTESIAN_POINT('Ctrl Pts',(1.81223801813988,-1.,-0.405933518411838));
#23465=CARTESIAN_POINT('Ctrl Pts',(1.80012077176221,-1.,-0.403107976170441));
#23466=CARTESIAN_POINT('Ctrl Pts',(1.78598826347533,-1.,-0.399919403783081));
#23467=CARTESIAN_POINT('Ctrl Pts',(1.7697556004756,-1.,-0.39634619612042));
#23468=CARTESIAN_POINT('Ctrl Pts',(1.75137405313962,-1.,-0.392375812294307));
#23469=CARTESIAN_POINT('Ctrl Pts',(1.7349317097561,-1.,-0.388877023509192));
#23470=CARTESIAN_POINT('Ctrl Pts',(1.72162022246158,-1.,-0.38607079032701));
#23471=CARTESIAN_POINT('Ctrl Pts',(1.71231062891958,-1.,-0.384119047315542));
#23472=CARTESIAN_POINT('Ctrl Pts',(1.7075470150345,-1.,-0.383122945602004));
#23473=CARTESIAN_POINT('',(1.74236521665491,-1.,-0.163289472382896));
#23474=CARTESIAN_POINT('Origin',(0.,-1.,0.));
#23475=CARTESIAN_POINT('',(2.19890268624765,-1.,-0.0694764450219582));
#23476=CARTESIAN_POINT('Ctrl Pts',(1.74236521665491,-1.,-0.163289472382896));
#23477=CARTESIAN_POINT('Ctrl Pts',(1.7472034950333,-1.,-0.163814161002002));
#23478=CARTESIAN_POINT('Ctrl Pts',(1.75666056638427,-1.,-0.164834765707159));
#23479=CARTESIAN_POINT('Ctrl Pts',(1.77018771684844,-1.,-0.1662793551464));
#23480=CARTESIAN_POINT('Ctrl Pts',(1.7869064998507,-1.,-0.168032772805197));
#23481=CARTESIAN_POINT('Ctrl Pts',(1.80561530629706,-1.,-0.169936923904608));
#23482=CARTESIAN_POINT('Ctrl Pts',(1.82215766811545,-1.,-0.171554770204119));
#23483=CARTESIAN_POINT('Ctrl Pts',(1.83658380527692,-1.,-0.1728894428919));
#23484=CARTESIAN_POINT('Ctrl Pts',(1.8489811319852,-1.,-0.173946627587732));
#23485=CARTESIAN_POINT('Ctrl Pts',(1.85948367088837,-1.,-0.17473525927603));
#23486=CARTESIAN_POINT('Ctrl Pts',(1.86828349694799,-1.,-0.175268337590758));
#23487=CARTESIAN_POINT('Ctrl Pts',(1.87563767773588,-1.,-0.175563480746485));
#23488=CARTESIAN_POINT('Ctrl Pts',(1.88188663145367,-1.,-0.175644148889699));
#23489=CARTESIAN_POINT('Ctrl Pts',(1.88742606273259,-1.,-0.175538155840648));
#23490=CARTESIAN_POINT('Ctrl Pts',(1.892646301985,-1.,-0.175274276190844));
#23491=CARTESIAN_POINT('Ctrl Pts',(1.89788101117132,-1.,-0.174879405091263));
#23492=CARTESIAN_POINT('Ctrl Pts',(1.90335253862834,-1.,-0.174375518661085));
#23493=CARTESIAN_POINT('Ctrl Pts',(1.90911693975267,-1.,-0.173776635257817));
#23494=CARTESIAN_POINT('Ctrl Pts',(1.91511429159527,-1.,-0.173090695383496));
#23495=CARTESIAN_POINT('Ctrl Pts',(1.9212233439798,-1.,-0.172321621259514));
#23496=CARTESIAN_POINT('Ctrl Pts',(1.92731093582036,-1.,-0.171471191532988));
#23497=CARTESIAN_POINT('Ctrl Pts',(1.93329183155539,-1.,-0.170541253116202));
#23498=CARTESIAN_POINT('Ctrl Pts',(1.93915639211581,-1.,-0.169534904817491));
#23499=CARTESIAN_POINT('Ctrl Pts',(1.94493757756931,-1.,-0.168455741607556));
#23500=CARTESIAN_POINT('Ctrl Pts',(1.95069027794294,-1.,-0.167307501784476));
#23501=CARTESIAN_POINT('Ctrl Pts',(1.9564675971873,-1.,-0.166093592002813));
#23502=CARTESIAN_POINT('Ctrl Pts',(1.96229379940136,-1.,-0.164816568920269));
#23503=CARTESIAN_POINT('Ctrl Pts',(1.96816512677967,-1.,-0.163478185457734));
#23504=CARTESIAN_POINT('Ctrl Pts',(1.97406280235188,-1.,-0.162079693556289));
#23505=CARTESIAN_POINT('Ctrl Pts',(1.97996195437559,-1.,-0.160622060784611));
#23506=CARTESIAN_POINT('Ctrl Pts',(1.98584238283292,-1.,-0.159106226437299));
#23507=CARTESIAN_POINT('Ctrl Pts',(1.99169810931908,-1.,-0.157533331459227));
#23508=CARTESIAN_POINT('Ctrl Pts',(1.99753284771497,-1.,-0.155904629548784));
#23509=CARTESIAN_POINT('Ctrl Pts',(2.00335565310543,-1.,-0.154221403049722));
#23510=CARTESIAN_POINT('Ctrl Pts',(2.00917680318424,-1.,-0.15248488362145));
#23511=CARTESIAN_POINT('Ctrl Pts',(2.01500291940238,-1.,-0.150696157673078));
#23512=CARTESIAN_POINT('Ctrl Pts',(2.02083464969894,-1.,-0.148856124775337));
#23513=CARTESIAN_POINT('Ctrl Pts',(2.02666926182017,-1.,-0.146965557332583));
#23514=CARTESIAN_POINT('Ctrl Pts',(2.03250223739942,-1.,-0.145025140186058));
#23515=CARTESIAN_POINT('Ctrl Pts',(2.03832911025912,-1.,-0.143035515058209));
#23516=CARTESIAN_POINT('Ctrl Pts',(2.04414757947916,-1.,-0.140997332152546));
#23517=CARTESIAN_POINT('Ctrl Pts',(2.04995762001328,-1.,-0.138911255368966));
#23518=CARTESIAN_POINT('Ctrl Pts',(2.05576044414264,-1.,-0.136777941218044));
#23519=CARTESIAN_POINT('Ctrl Pts',(2.06155781517842,-1.,-0.134598026192106));
#23520=CARTESIAN_POINT('Ctrl Pts',(2.06735123910326,-1.,-0.132372111547711));
#23521=CARTESIAN_POINT('Ctrl Pts',(2.07314114713063,-1.,-0.130100748328404));
#23522=CARTESIAN_POINT('Ctrl Pts',(2.07892715110987,-1.,-0.12778444527612));
#23523=CARTESIAN_POINT('Ctrl Pts',(2.08470840653643,-1.,-0.125423679412062));
#23524=CARTESIAN_POINT('Ctrl Pts',(2.09048392424825,-1.,-0.123018905621083));
#23525=CARTESIAN_POINT('Ctrl Pts',(2.0962529286773,-1.,-0.120570567965122));
#23526=CARTESIAN_POINT('Ctrl Pts',(2.102015121329,-1.,-0.118079107988356));
#23527=CARTESIAN_POINT('Ctrl Pts',(2.10777050261309,-1.,-0.115544957687927));
#23528=CARTESIAN_POINT('Ctrl Pts',(2.11351924490306,-1.,-0.112968534419737));
#23529=CARTESIAN_POINT('Ctrl Pts',(2.11926155590865,-1.,-0.110350236135025));
#23530=CARTESIAN_POINT('Ctrl Pts',(2.12499752307,-1.,-0.10769043523109));
#23531=CARTESIAN_POINT('Ctrl Pts',(2.13072704887293,-1.,-0.10498947915274));
#23532=CARTESIAN_POINT('Ctrl Pts',(2.13644992667165,-1.,-0.102247700556101));
#23533=CARTESIAN_POINT('Ctrl Pts',(2.14216588396025,-1.,-0.0994654261990917));
#23534=CARTESIAN_POINT('Ctrl Pts',(2.14787463531795,-1.,-0.096642985230546));
#23535=CARTESIAN_POINT('Ctrl Pts',(2.1535759397817,-1.,-0.0937807218867645));
#23536=CARTESIAN_POINT('Ctrl Pts',(2.15926961544516,-1.,-0.0908789888107267));
#23537=CARTESIAN_POINT('Ctrl Pts',(2.16495552645014,-1.,-0.0879381291386924));
#23538=CARTESIAN_POINT('Ctrl Pts',(2.17063357870952,-1.,-0.0849584620835374));
#23539=CARTESIAN_POINT('Ctrl Pts',(2.176303712113,-1.,-0.0819402680872767));
#23540=CARTESIAN_POINT('Ctrl Pts',(2.18196589448887,-1.,-0.0788837727685244));
#23541=CARTESIAN_POINT('Ctrl Pts',(2.1876201139953,-1.,-0.0757891465836149));
#23542=CARTESIAN_POINT('Ctrl Pts',(2.19213712013662,-1.,-0.0732830357306726));
#23543=CARTESIAN_POINT('Ctrl Pts',(2.19552129484002,-1.,-0.0713863779526155));
#23544=CARTESIAN_POINT('Ctrl Pts',(2.19777582085423,-1.,-0.0701143536325491));
#23545=CARTESIAN_POINT('Ctrl Pts',(2.19890268624765,-1.,-0.0694764450219582));
#23546=CARTESIAN_POINT('',(2.19890268624765,-1.,0.0694764450219582));
#23547=CARTESIAN_POINT('',(2.19890268624765,-1.,-0.0694764450219582));
#23548=CARTESIAN_POINT('',(1.74236521665491,-1.,0.163289472382896));
#23549=CARTESIAN_POINT('Ctrl Pts',(2.19890268624765,-1.,0.0694764450219582));
#23550=CARTESIAN_POINT('Ctrl Pts',(2.19777582085261,-1.,0.0701143536324925));
#23551=CARTESIAN_POINT('Ctrl Pts',(2.19552129483562,-1.,0.0713863779524626));
#23552=CARTESIAN_POINT('Ctrl Pts',(2.19213712012956,-1.,0.0732830357304275));
#23553=CARTESIAN_POINT('Ctrl Pts',(2.1876201139874,-1.,0.075789146583341));
#23554=CARTESIAN_POINT('Ctrl Pts',(2.18196589448304,-1.,0.0788837727683226));
#23555=CARTESIAN_POINT('Ctrl Pts',(2.1763037121106,-1.,0.0819402680871938));
#23556=CARTESIAN_POINT('Ctrl Pts',(2.17063357871031,-1.,0.0849584620835642));
#23557=CARTESIAN_POINT('Ctrl Pts',(2.16495552645275,-1.,0.0879381291387821));
#23558=CARTESIAN_POINT('Ctrl Pts',(2.15926961544808,-1.,0.0908789888108265));
#23559=CARTESIAN_POINT('Ctrl Pts',(2.15357593978377,-1.,0.0937807218868344));
#23560=CARTESIAN_POINT('Ctrl Pts',(2.14787463531864,-1.,0.0966429852305688));
#23561=CARTESIAN_POINT('Ctrl Pts',(2.14216588395974,-1.,0.0994654261990741));
#23562=CARTESIAN_POINT('Ctrl Pts',(2.13644992667052,-1.,0.102247700556063));
#23563=CARTESIAN_POINT('Ctrl Pts',(2.1307270488718,-1.,0.104989479152703));
#23564=CARTESIAN_POINT('Ctrl Pts',(2.12499752306927,-1.,0.107690435231068));
#23565=CARTESIAN_POINT('Ctrl Pts',(2.11926155590849,-1.,0.11035023613502));
#23566=CARTESIAN_POINT('Ctrl Pts',(2.11351924490335,-1.,0.112968534419746));
#23567=CARTESIAN_POINT('Ctrl Pts',(2.10777050261359,-1.,0.11554495768794));
#23568=CARTESIAN_POINT('Ctrl Pts',(2.10201512132945,-1.,0.118079107988368));
#23569=CARTESIAN_POINT('Ctrl Pts',(2.09625292867756,-1.,0.120570567965129));
#23570=CARTESIAN_POINT('Ctrl Pts',(2.09048392424826,-1.,0.123018905621083));
#23571=CARTESIAN_POINT('Ctrl Pts',(2.08470840653628,-1.,0.125423679412058));
#23572=CARTESIAN_POINT('Ctrl Pts',(2.07892715110967,-1.,0.127784445276116));
#23573=CARTESIAN_POINT('Ctrl Pts',(2.07314114713047,-1.,0.1301007483284));
#23574=CARTESIAN_POINT('Ctrl Pts',(2.06735123910319,-1.,0.132372111547709));
#23575=CARTESIAN_POINT('Ctrl Pts',(2.06155781517844,-1.,0.134598026192107));
#23576=CARTESIAN_POINT('Ctrl Pts',(2.0557604441427,-1.,0.136777941218044));
#23577=CARTESIAN_POINT('Ctrl Pts',(2.04995762001333,-1.,0.138911255368966));
#23578=CARTESIAN_POINT('Ctrl Pts',(2.04414757947919,-1.,0.140997332152545));
#23579=CARTESIAN_POINT('Ctrl Pts',(2.03832911025913,-1.,0.143035515058208));
#23580=CARTESIAN_POINT('Ctrl Pts',(2.03250223739941,-1.,0.145025140186058));
#23581=CARTESIAN_POINT('Ctrl Pts',(2.02666926182017,-1.,0.146965557332586));
#23582=CARTESIAN_POINT('Ctrl Pts',(2.02083464969897,-1.,0.148856124775342));
#23583=CARTESIAN_POINT('Ctrl Pts',(2.01500291940243,-1.,0.150696157673084));
#23584=CARTESIAN_POINT('Ctrl Pts',(2.00917680318426,-1.,0.152484883621452));
#23585=CARTESIAN_POINT('Ctrl Pts',(2.00335565310539,-1.,0.154221403049719));
#23586=CARTESIAN_POINT('Ctrl Pts',(1.99753284771487,-1.,0.155904629548774));
#23587=CARTESIAN_POINT('Ctrl Pts',(1.99169810931893,-1.,0.157533331459215));
#23588=CARTESIAN_POINT('Ctrl Pts',(1.98584238283279,-1.,0.159106226437288));
#23589=CARTESIAN_POINT('Ctrl Pts',(1.97996195437557,-1.,0.16062206078461));
#23590=CARTESIAN_POINT('Ctrl Pts',(1.97406280235204,-1.,0.162079693556302));
#23591=CARTESIAN_POINT('Ctrl Pts',(1.96816512678,-1.,0.16347818545776));
#23592=CARTESIAN_POINT('Ctrl Pts',(1.96229379940174,-1.,0.1648165689203));
#23593=CARTESIAN_POINT('Ctrl Pts',(1.95646759718755,-1.,0.166093592002832));
#23594=CARTESIAN_POINT('Ctrl Pts',(1.95069027794286,-1.,0.167307501784469));
#23595=CARTESIAN_POINT('Ctrl Pts',(1.94493757756879,-1.,0.168455741607515));
#23596=CARTESIAN_POINT('Ctrl Pts',(1.93915639211497,-1.,0.169534904817425));
#23597=CARTESIAN_POINT('Ctrl Pts',(1.93329183155455,-1.,0.170541253116136));
#23598=CARTESIAN_POINT('Ctrl Pts',(1.92731093582,-1.,0.17147119153296));
#23599=CARTESIAN_POINT('Ctrl Pts',(1.92122334398034,-1.,0.172321621259556));
#23600=CARTESIAN_POINT('Ctrl Pts',(1.91511429159681,-1.,0.173090695383619));
#23601=CARTESIAN_POINT('Ctrl Pts',(1.90911693975475,-1.,0.173776635257983));
#23602=CARTESIAN_POINT('Ctrl Pts',(1.90335253863003,-1.,0.174375518661222));
#23603=CARTESIAN_POINT('Ctrl Pts',(1.89788101117148,-1.,0.174879405091277));
#23604=CARTESIAN_POINT('Ctrl Pts',(1.89264630198279,-1.,0.175274276190664));
#23605=CARTESIAN_POINT('Ctrl Pts',(1.88742606272818,-1.,0.175538155840286));
#23606=CARTESIAN_POINT('Ctrl Pts',(1.88188663144846,-1.,0.175644148889271));
#23607=CARTESIAN_POINT('Ctrl Pts',(1.87563767773249,-1.,0.175563480746205));
#23608=CARTESIAN_POINT('Ctrl Pts',(1.86828349694972,-1.,0.1752683375909));
#23609=CARTESIAN_POINT('Ctrl Pts',(1.85948367089838,-1.,0.174735259276856));
#23610=CARTESIAN_POINT('Ctrl Pts',(1.84898113200543,-1.,0.173946627589401));
#23611=CARTESIAN_POINT('Ctrl Pts',(1.83658380530747,-1.,0.17288944289442));
#23612=CARTESIAN_POINT('Ctrl Pts',(1.82215766815414,-1.,0.171554770207306));
#23613=CARTESIAN_POINT('Ctrl Pts',(1.80561530633924,-1.,0.169936923908078));
#23614=CARTESIAN_POINT('Ctrl Pts',(1.78690649988931,-1.,0.16803277280837));
#23615=CARTESIAN_POINT('Ctrl Pts',(1.77018771687692,-1.,0.166279355148738));
#23616=CARTESIAN_POINT('Ctrl Pts',(1.75666056640041,-1.,0.164834765708484));
#23617=CARTESIAN_POINT('Ctrl Pts',(1.74720349503904,-1.,0.163814161002474));
#23618=CARTESIAN_POINT('Ctrl Pts',(1.74236521665491,-1.,0.163289472382896));
#23619=CARTESIAN_POINT('',(1.7075470150345,-1.,0.383122945602004));
#23620=CARTESIAN_POINT('Origin',(0.,-1.,0.));
#23621=CARTESIAN_POINT('',(2.11275013067528,-1.,0.613422273260091));
#23622=CARTESIAN_POINT('Ctrl Pts',(1.7075470150345,-1.,0.383122945602004));
#23623=CARTESIAN_POINT('Ctrl Pts',(1.71231062891398,-1.,0.384119047314215));
#23624=CARTESIAN_POINT('Ctrl Pts',(1.72162022244582,-1.,0.386070790323281));
#23625=CARTESIAN_POINT('Ctrl Pts',(1.73493170972829,-1.,0.388877023502615));
#23626=CARTESIAN_POINT('Ctrl Pts',(1.75137405310193,-1.,0.392375812285396));
#23627=CARTESIAN_POINT('Ctrl Pts',(1.76975560043442,-1.,0.396346196110688));
#23628=CARTESIAN_POINT('Ctrl Pts',(1.78598826343754,-1.,0.399919403774156));
#23629=CARTESIAN_POINT('Ctrl Pts',(1.80012077173238,-1.,0.403107976163396));
#23630=CARTESIAN_POINT('Ctrl Pts',(1.81223801812013,-1.,0.405933518407176));
#23631=CARTESIAN_POINT('Ctrl Pts',(1.82247022677562,-1.,0.408428948106228));
#23632=CARTESIAN_POINT('Ctrl Pts',(1.83100408895047,-1.,0.410641256301276));
#23633=CARTESIAN_POINT('Ctrl Pts',(1.8380895347617,-1.,0.412633125322945));
#23634=CARTESIAN_POINT('Ctrl Pts',(1.84405757074218,-1.,0.414487438255542));
#23635=CARTESIAN_POINT('Ctrl Pts',(1.84929312930314,-1.,0.416300022039885));
#23636=CARTESIAN_POINT('Ctrl Pts',(1.8541763285645,-1.,0.418164129144046));
#23637=CARTESIAN_POINT('Ctrl Pts',(1.8590328109667,-1.,0.420157287975583));
#23638=CARTESIAN_POINT('Ctrl Pts',(1.86408083333863,-1.,0.422327307417885));
#23639=CARTESIAN_POINT('Ctrl Pts',(1.8693780394412,-1.,0.424678177290876));
#23640=CARTESIAN_POINT('Ctrl Pts',(1.87486989291333,-1.,0.427183828518743));
#23641=CARTESIAN_POINT('Ctrl Pts',(1.88044229001778,-1.,0.429803062482217));
#23642=CARTESIAN_POINT('Ctrl Pts',(1.88596913666828,-1.,0.432493038548833));
#23643=CARTESIAN_POINT('Ctrl Pts',(1.89136993975585,-1.,0.43522566096358));
#23644=CARTESIAN_POINT('Ctrl Pts',(1.89663648956549,-1.,0.437995003948443));
#23645=CARTESIAN_POINT('Ctrl Pts',(1.90180124389137,-1.,0.440807833704161));
#23646=CARTESIAN_POINT('Ctrl Pts',(1.90691756144906,-1.,0.443677556849171));
#23647=CARTESIAN_POINT('Ctrl Pts',(1.91203699981095,-1.,0.446617343485651));
#23648=CARTESIAN_POINT('Ctrl Pts',(1.91718342555717,-1.,0.449632260106572));
#23649=CARTESIAN_POINT('Ctrl Pts',(1.9223538064847,-1.,0.452719478359356));
#23650=CARTESIAN_POINT('Ctrl Pts',(1.92753067150461,-1.,0.455872005174336));
#23651=CARTESIAN_POINT('Ctrl Pts',(1.93269066517936,-1.,0.459081234547932));
#23652=CARTESIAN_POINT('Ctrl Pts',(1.93781486640834,-1.,0.462340031009087));
#23653=CARTESIAN_POINT('Ctrl Pts',(1.94289794196205,-1.,0.465645462026065));
#23654=CARTESIAN_POINT('Ctrl Pts',(1.94794381136524,-1.,0.468997482913158));
#23655=CARTESIAN_POINT('Ctrl Pts',(1.95296148278136,-1.,0.47239767226408));
#23656=CARTESIAN_POINT('Ctrl Pts',(1.95796111148175,-1.,0.475848034683172));
#23657=CARTESIAN_POINT('Ctrl Pts',(1.96294933055938,-1.,0.479349583074846));
#23658=CARTESIAN_POINT('Ctrl Pts',(1.96792703422358,-1.,0.482901662120687));
#23659=CARTESIAN_POINT('Ctrl Pts',(1.97289186263272,-1.,0.486502692907661));
#23660=CARTESIAN_POINT('Ctrl Pts',(1.97783973019229,-1.,0.490150627860955));
#23661=CARTESIAN_POINT('Ctrl Pts',(1.9827665876182,-1.,0.493843476541493));
#23662=CARTESIAN_POINT('Ctrl Pts',(1.98767044752929,-1.,0.497579909545564));
#23663=CARTESIAN_POINT('Ctrl Pts',(1.9925514912615,-1.,0.501359287727129));
#23664=CARTESIAN_POINT('Ctrl Pts',(1.99741107463567,-1.,0.505181361323011));
#23665=CARTESIAN_POINT('Ctrl Pts',(2.00225107134733,-1.,0.509046069886152));
#23666=CARTESIAN_POINT('Ctrl Pts',(2.00707309946955,-1.,0.512953306961814));
#23667=CARTESIAN_POINT('Ctrl Pts',(2.01187773939257,-1.,0.516902681728733));
#23668=CARTESIAN_POINT('Ctrl Pts',(2.01666477917305,-1.,0.520893590399429));
#23669=CARTESIAN_POINT('Ctrl Pts',(2.02143356304712,-1.,0.524925318333519));
#23670=CARTESIAN_POINT('Ctrl Pts',(2.02618329083289,-1.,0.528997127241911));
#23671=CARTESIAN_POINT('Ctrl Pts',(2.03091336214401,-1.,0.533108355132905));
#23672=CARTESIAN_POINT('Ctrl Pts',(2.03562362953993,-1.,0.537258489833135));
#23673=CARTESIAN_POINT('Ctrl Pts',(2.0403142269048,-1.,0.54144712061552));
#23674=CARTESIAN_POINT('Ctrl Pts',(2.0449854471456,-1.,0.545673903817349));
#23675=CARTESIAN_POINT('Ctrl Pts',(2.04963761077974,-1.,0.549938525150342));
#23676=CARTESIAN_POINT('Ctrl Pts',(2.05427091604482,-1.,0.55424065746411));
#23677=CARTESIAN_POINT('Ctrl Pts',(2.05888537756571,-1.,0.558579940185468));
#23678=CARTESIAN_POINT('Ctrl Pts',(2.06348090160697,-1.,0.562955993082574));
#23679=CARTESIAN_POINT('Ctrl Pts',(2.06805732997383,-1.,0.56736842118123));
#23680=CARTESIAN_POINT('Ctrl Pts',(2.07261449292757,-1.,0.571816823242411));
#23681=CARTESIAN_POINT('Ctrl Pts',(2.07715226767361,-1.,0.576300797416275));
#23682=CARTESIAN_POINT('Ctrl Pts',(2.08167059018138,-1.,0.580819952107257));
#23683=CARTESIAN_POINT('Ctrl Pts',(2.086169437277,-1.,0.585373918990895));
#23684=CARTESIAN_POINT('Ctrl Pts',(2.09064881812053,-1.,0.58996236540319));
#23685=CARTESIAN_POINT('Ctrl Pts',(2.09510876220501,-1.,0.594585006052824));
#23686=CARTESIAN_POINT('Ctrl Pts',(2.09954930865331,-1.,0.599241616422144));
#23687=CARTESIAN_POINT('Ctrl Pts',(2.10397049887709,-1.,0.603932030738212));
#23688=CARTESIAN_POINT('Ctrl Pts',(2.10749199615859,-1.,0.607711315456826));
#23689=CARTESIAN_POINT('Ctrl Pts',(2.11012443807661,-1.,0.610560911691114));
#23690=CARTESIAN_POINT('Ctrl Pts',(2.11187554260142,-1.,0.61246736556225));
#23691=CARTESIAN_POINT('Ctrl Pts',(2.11275013067528,-1.,0.613422273260091));
#23692=CARTESIAN_POINT('',(2.0698113262342,-1.,0.745574324794401));
#23693=CARTESIAN_POINT('',(2.11275013067528,-1.,0.613422273260091));
#23694=CARTESIAN_POINT('Ctrl Pts',(2.0698113262342,-1.,0.745574324794401));
#23695=CARTESIAN_POINT('Ctrl Pts',(2.06854248895575,-1.,0.74583279137781));
#23696=CARTESIAN_POINT('Ctrl Pts',(2.06600523016401,-1.,0.746345871542696));
#23697=CARTESIAN_POINT('Ctrl Pts',(2.06220058927162,-1.,0.747103932785504));
#23698=CARTESIAN_POINT('Ctrl Pts',(2.05713023030263,-1.,0.748091554181101));
#23699=CARTESIAN_POINT('Ctrl Pts',(2.05079645591606,-1.,0.749287468663053));
#23700=CARTESIAN_POINT('Ctrl Pts',(2.04446689147754,-1.,0.750444657874758));
#23701=CARTESIAN_POINT('Ctrl Pts',(2.03814160092173,-1.,0.751562963361384));
#23702=CARTESIAN_POINT('Ctrl Pts',(2.03182068456467,-1.,0.752642180488104));
#23703=CARTESIAN_POINT('Ctrl Pts',(2.02550428623587,-1.,0.753682061113766));
#23704=CARTESIAN_POINT('Ctrl Pts',(2.01919259406003,-1.,0.75468233072352));
#23705=CARTESIAN_POINT('Ctrl Pts',(2.01288584328149,-1.,0.755642704958101));
#23706=CARTESIAN_POINT('Ctrl Pts',(2.00658431587682,-1.,0.756562904646496));
#23707=CARTESIAN_POINT('Ctrl Pts',(2.00028834739072,-1.,0.757442676862342));
#23708=CARTESIAN_POINT('Ctrl Pts',(1.9939983109871,-1.,0.758281796766377));
#23709=CARTESIAN_POINT('Ctrl Pts',(1.98771456680806,-1.,0.759080037802243));
#23710=CARTESIAN_POINT('Ctrl Pts',(1.98143741418156,-1.,0.759837147452135));
#23711=CARTESIAN_POINT('Ctrl Pts',(1.97516705321521,-1.,0.760552825409856));
#23712=CARTESIAN_POINT('Ctrl Pts',(1.96890351582545,-1.,0.761226690483986));
#23713=CARTESIAN_POINT('Ctrl Pts',(1.96264672744229,-1.,0.761858300014575));
#23714=CARTESIAN_POINT('Ctrl Pts',(1.95639665309893,-1.,0.762447203806264));
#23715=CARTESIAN_POINT('Ctrl Pts',(1.95015342590025,-1.,0.762992990878774));
#23716=CARTESIAN_POINT('Ctrl Pts',(1.94391746617626,-1.,0.763495333538581));
#23717=CARTESIAN_POINT('Ctrl Pts',(1.93768964875867,-1.,0.763954049121394));
#23718=CARTESIAN_POINT('Ctrl Pts',(1.93147105496367,-1.,0.76436901067389));
#23719=CARTESIAN_POINT('Ctrl Pts',(1.92526263537041,-1.,0.764740025488189));
#23720=CARTESIAN_POINT('Ctrl Pts',(1.91906491634197,-1.,0.765066729667095));
#23721=CARTESIAN_POINT('Ctrl Pts',(1.91287765805174,-1.,0.765348465884739));
#23722=CARTESIAN_POINT('Ctrl Pts',(1.90669961402362,-1.,0.765584196937937));
#23723=CARTESIAN_POINT('Ctrl Pts',(1.90052930393599,-1.,0.765772772593395));
#23724=CARTESIAN_POINT('Ctrl Pts',(1.89436577771389,-1.,0.765913193856979));
#23725=CARTESIAN_POINT('Ctrl Pts',(1.88820926433409,-1.,0.76600483706209));
#23726=CARTESIAN_POINT('Ctrl Pts',(1.88206215302561,-1.,0.766047794851869));
#23727=CARTESIAN_POINT('Ctrl Pts',(1.87592888967886,-1.,0.766042837036759));
#23728=CARTESIAN_POINT('Ctrl Pts',(1.86981398314345,-1.,0.765990708546112));
#23729=CARTESIAN_POINT('Ctrl Pts',(1.86372027063314,-1.,0.765891519092557));
#23730=CARTESIAN_POINT('Ctrl Pts',(1.85764741390391,-1.,0.765744212909305));
#23731=CARTESIAN_POINT('Ctrl Pts',(1.85158945130054,-1.,0.765545710619023));
#23732=CARTESIAN_POINT('Ctrl Pts',(1.8455369887591,-1.,0.765291664861972));
#23733=CARTESIAN_POINT('Ctrl Pts',(1.83948181064823,-1.,0.764978057881688));
#23734=CARTESIAN_POINT('Ctrl Pts',(1.8334207722714,-1.,0.764602549687846));
#23735=CARTESIAN_POINT('Ctrl Pts',(1.8273599120008,-1.,0.764165902606056));
#23736=CARTESIAN_POINT('Ctrl Pts',(1.82131873145297,-1.,0.763673465462854));
#23737=CARTESIAN_POINT('Ctrl Pts',(1.81532118405566,-1.,0.763132003836783));
#23738=CARTESIAN_POINT('Ctrl Pts',(1.80938551463989,-1.,0.762546129464036));
#23739=CARTESIAN_POINT('Ctrl Pts',(1.80351583877334,-1.,0.761915336443516));
#23740=CARTESIAN_POINT('Ctrl Pts',(1.79768986997735,-1.,0.761229695230359));
#23741=CARTESIAN_POINT('Ctrl Pts',(1.79185815610802,-1.,0.760469555880425));
#23742=CARTESIAN_POINT('Ctrl Pts',(1.78596964884526,-1.,0.759614401109868));
#23743=CARTESIAN_POINT('Ctrl Pts',(1.77999411220912,-1.,0.75865062667738));
#23744=CARTESIAN_POINT('Ctrl Pts',(1.77394167108342,-1.,0.757578264077238));
#23745=CARTESIAN_POINT('Ctrl Pts',(1.76789396003141,-1.,0.756421896028403));
#23746=CARTESIAN_POINT('Ctrl Pts',(1.7619781724032,-1.,0.755220979975262));
#23747=CARTESIAN_POINT('Ctrl Pts',(1.75631083600175,-1.,0.75400925402848));
#23748=CARTESIAN_POINT('Ctrl Pts',(1.75095139468809,-1.,0.752797683531377));
#23749=CARTESIAN_POINT('Ctrl Pts',(1.74585086852298,-1.,0.751555614163629));
#23750=CARTESIAN_POINT('Ctrl Pts',(1.74080458266705,-1.,0.750193435979541));
#23751=CARTESIAN_POINT('Ctrl Pts',(1.73550351679848,-1.,0.748582462954855));
#23752=CARTESIAN_POINT('Ctrl Pts',(1.72958533647399,-1.,0.746574710096437));
#23753=CARTESIAN_POINT('Ctrl Pts',(1.7226822991693,-1.,0.744021445433765));
#23754=CARTESIAN_POINT('Ctrl Pts',(1.71447789751927,-1.,0.740795162032088));
#23755=CARTESIAN_POINT('Ctrl Pts',(1.70473309006121,-1.,0.736799665724771));
#23756=CARTESIAN_POINT('Ctrl Pts',(1.69326921975743,-1.,0.731963238697195));
#23757=CARTESIAN_POINT('Ctrl Pts',(1.67996158455503,-1.,0.726235967997433));
#23758=CARTESIAN_POINT('Ctrl Pts',(1.6647288055568,-1.,0.719585433804282));
#23759=CARTESIAN_POINT('Ctrl Pts',(1.64752408832016,-1.,0.711993139355394));
#23760=CARTESIAN_POINT('Ctrl Pts',(1.63216541664676,-1.,0.705159151988319));
#23761=CARTESIAN_POINT('Ctrl Pts',(1.61974673472612,-1.,0.699605146405088));
#23762=CARTESIAN_POINT('Ctrl Pts',(1.61106790958151,-1.,0.695712097881194));
#23763=CARTESIAN_POINT('Ctrl Pts',(1.60662857109684,-1.,0.693717979106306));
#23764=CARTESIAN_POINT('Origin',(0.,-1.,0.));
#23765=CARTESIAN_POINT('Origin',(0.,0.,0.));
#23766=CARTESIAN_POINT('Origin',(0.,2.2,0.));
#23767=CARTESIAN_POINT('Origin',(0.,1.,0.));
#23768=CARTESIAN_POINT('',(-1.4,2.2,1.71450551880629E-16));
#23769=CARTESIAN_POINT('Origin',(0.,2.2,0.));
#23770=CARTESIAN_POINT('',(-1.4,1.,1.71450551880629E-16));
#23771=CARTESIAN_POINT('',(-1.4,1.,1.71450551880629E-16));
#23772=CARTESIAN_POINT('Origin',(0.,1.,0.));
#23773=CARTESIAN_POINT('Origin',(0.,2.2,0.));
#23774=CARTESIAN_POINT('Ctrl Pts',(2.11275013067528,-1.,0.613422273260091));
#23775=CARTESIAN_POINT('Ctrl Pts',(2.11275013067528,1.,0.613422273260091));
#23776=CARTESIAN_POINT('Ctrl Pts',(2.11187554260142,-1.,0.61246736556225));
#23777=CARTESIAN_POINT('Ctrl Pts',(2.11187554260142,1.,0.61246736556225));
#23778=CARTESIAN_POINT('Ctrl Pts',(2.11012443807661,-1.,0.610560911691114));
#23779=CARTESIAN_POINT('Ctrl Pts',(2.11012443807661,1.,0.610560911691114));
#23780=CARTESIAN_POINT('Ctrl Pts',(2.10749199615859,-1.,0.607711315456826));
#23781=CARTESIAN_POINT('Ctrl Pts',(2.10749199615859,1.,0.607711315456826));
#23782=CARTESIAN_POINT('Ctrl Pts',(2.10397049887709,-1.,0.603932030738212));
#23783=CARTESIAN_POINT('Ctrl Pts',(2.10397049887709,1.,0.603932030738212));
#23784=CARTESIAN_POINT('Ctrl Pts',(2.09954930865331,-1.,0.599241616422144));
#23785=CARTESIAN_POINT('Ctrl Pts',(2.09954930865331,1.,0.599241616422144));
#23786=CARTESIAN_POINT('Ctrl Pts',(2.09510876220501,-1.,0.594585006052824));
#23787=CARTESIAN_POINT('Ctrl Pts',(2.09510876220501,1.,0.594585006052824));
#23788=CARTESIAN_POINT('Ctrl Pts',(2.09064881812053,-1.,0.58996236540319));
#23789=CARTESIAN_POINT('Ctrl Pts',(2.09064881812053,1.,0.58996236540319));
#23790=CARTESIAN_POINT('Ctrl Pts',(2.086169437277,-1.,0.585373918990895));
#23791=CARTESIAN_POINT('Ctrl Pts',(2.086169437277,1.,0.585373918990895));
#23792=CARTESIAN_POINT('Ctrl Pts',(2.08167059018138,-1.,0.580819952107257));
#23793=CARTESIAN_POINT('Ctrl Pts',(2.08167059018138,1.,0.580819952107257));
#23794=CARTESIAN_POINT('Ctrl Pts',(2.07715226767361,-1.,0.576300797416275));
#23795=CARTESIAN_POINT('Ctrl Pts',(2.07715226767361,1.,0.576300797416275));
#23796=CARTESIAN_POINT('Ctrl Pts',(2.07261449292757,-1.,0.571816823242411));
#23797=CARTESIAN_POINT('Ctrl Pts',(2.07261449292757,1.,0.571816823242411));
#23798=CARTESIAN_POINT('Ctrl Pts',(2.06805732997383,-1.,0.56736842118123));
#23799=CARTESIAN_POINT('Ctrl Pts',(2.06805732997383,1.,0.56736842118123));
#23800=CARTESIAN_POINT('Ctrl Pts',(2.06348090160697,-1.,0.562955993082574));
#23801=CARTESIAN_POINT('Ctrl Pts',(2.06348090160697,1.,0.562955993082574));
#23802=CARTESIAN_POINT('Ctrl Pts',(2.05888537756571,-1.,0.558579940185468));
#23803=CARTESIAN_POINT('Ctrl Pts',(2.05888537756571,1.,0.558579940185468));
#23804=CARTESIAN_POINT('Ctrl Pts',(2.05427091604482,-1.,0.55424065746411));
#23805=CARTESIAN_POINT('Ctrl Pts',(2.05427091604482,1.,0.55424065746411));
#23806=CARTESIAN_POINT('Ctrl Pts',(2.04963761077974,-1.,0.549938525150342));
#23807=CARTESIAN_POINT('Ctrl Pts',(2.04963761077974,1.,0.549938525150342));
#23808=CARTESIAN_POINT('Ctrl Pts',(2.0449854471456,-1.,0.545673903817349));
#23809=CARTESIAN_POINT('Ctrl Pts',(2.0449854471456,1.,0.545673903817349));
#23810=CARTESIAN_POINT('Ctrl Pts',(2.0403142269048,-1.,0.54144712061552));
#23811=CARTESIAN_POINT('Ctrl Pts',(2.0403142269048,1.,0.54144712061552));
#23812=CARTESIAN_POINT('Ctrl Pts',(2.03562362953993,-1.,0.537258489833135));
#23813=CARTESIAN_POINT('Ctrl Pts',(2.03562362953993,1.,0.537258489833135));
#23814=CARTESIAN_POINT('Ctrl Pts',(2.03091336214401,-1.,0.533108355132905));
#23815=CARTESIAN_POINT('Ctrl Pts',(2.03091336214401,1.,0.533108355132905));
#23816=CARTESIAN_POINT('Ctrl Pts',(2.02618329083289,-1.,0.528997127241911));
#23817=CARTESIAN_POINT('Ctrl Pts',(2.02618329083289,1.,0.528997127241911));
#23818=CARTESIAN_POINT('Ctrl Pts',(2.02143356304712,-1.,0.524925318333519));
#23819=CARTESIAN_POINT('Ctrl Pts',(2.02143356304712,1.,0.524925318333519));
#23820=CARTESIAN_POINT('Ctrl Pts',(2.01666477917305,-1.,0.520893590399429));
#23821=CARTESIAN_POINT('Ctrl Pts',(2.01666477917305,1.,0.520893590399429));
#23822=CARTESIAN_POINT('Ctrl Pts',(2.01187773939257,-1.,0.516902681728733));
#23823=CARTESIAN_POINT('Ctrl Pts',(2.01187773939257,1.,0.516902681728733));
#23824=CARTESIAN_POINT('Ctrl Pts',(2.00707309946955,-1.,0.512953306961814));
#23825=CARTESIAN_POINT('Ctrl Pts',(2.00707309946955,1.,0.512953306961814));
#23826=CARTESIAN_POINT('Ctrl Pts',(2.00225107134733,-1.,0.509046069886152));
#23827=CARTESIAN_POINT('Ctrl Pts',(2.00225107134733,1.,0.509046069886152));
#23828=CARTESIAN_POINT('Ctrl Pts',(1.99741107463567,-1.,0.505181361323011));
#23829=CARTESIAN_POINT('Ctrl Pts',(1.99741107463567,1.,0.505181361323011));
#23830=CARTESIAN_POINT('Ctrl Pts',(1.9925514912615,-1.,0.501359287727129));
#23831=CARTESIAN_POINT('Ctrl Pts',(1.9925514912615,1.,0.501359287727129));
#23832=CARTESIAN_POINT('Ctrl Pts',(1.98767044752929,-1.,0.497579909545564));
#23833=CARTESIAN_POINT('Ctrl Pts',(1.98767044752929,1.,0.497579909545564));
#23834=CARTESIAN_POINT('Ctrl Pts',(1.9827665876182,-1.,0.493843476541493));
#23835=CARTESIAN_POINT('Ctrl Pts',(1.9827665876182,1.,0.493843476541493));
#23836=CARTESIAN_POINT('Ctrl Pts',(1.97783973019229,-1.,0.490150627860955));
#23837=CARTESIAN_POINT('Ctrl Pts',(1.97783973019229,1.,0.490150627860955));
#23838=CARTESIAN_POINT('Ctrl Pts',(1.97289186263272,-1.,0.486502692907661));
#23839=CARTESIAN_POINT('Ctrl Pts',(1.97289186263272,1.,0.486502692907661));
#23840=CARTESIAN_POINT('Ctrl Pts',(1.96792703422358,-1.,0.482901662120687));
#23841=CARTESIAN_POINT('Ctrl Pts',(1.96792703422358,1.,0.482901662120687));
#23842=CARTESIAN_POINT('Ctrl Pts',(1.96294933055938,-1.,0.479349583074846));
#23843=CARTESIAN_POINT('Ctrl Pts',(1.96294933055938,1.,0.479349583074846));
#23844=CARTESIAN_POINT('Ctrl Pts',(1.95796111148175,-1.,0.475848034683172));
#23845=CARTESIAN_POINT('Ctrl Pts',(1.95796111148175,1.,0.475848034683172));
#23846=CARTESIAN_POINT('Ctrl Pts',(1.95296148278136,-1.,0.47239767226408));
#23847=CARTESIAN_POINT('Ctrl Pts',(1.95296148278136,1.,0.47239767226408));
#23848=CARTESIAN_POINT('Ctrl Pts',(1.94794381136524,-1.,0.468997482913158));
#23849=CARTESIAN_POINT('Ctrl Pts',(1.94794381136524,1.,0.468997482913158));
#23850=CARTESIAN_POINT('Ctrl Pts',(1.94289794196205,-1.,0.465645462026065));
#23851=CARTESIAN_POINT('Ctrl Pts',(1.94289794196205,1.,0.465645462026065));
#23852=CARTESIAN_POINT('Ctrl Pts',(1.93781486640834,-1.,0.462340031009087));
#23853=CARTESIAN_POINT('Ctrl Pts',(1.93781486640834,1.,0.462340031009087));
#23854=CARTESIAN_POINT('Ctrl Pts',(1.93269066517936,-1.,0.459081234547932));
#23855=CARTESIAN_POINT('Ctrl Pts',(1.93269066517936,1.,0.459081234547932));
#23856=CARTESIAN_POINT('Ctrl Pts',(1.92753067150461,-1.,0.455872005174336));
#23857=CARTESIAN_POINT('Ctrl Pts',(1.92753067150461,1.,0.455872005174336));
#23858=CARTESIAN_POINT('Ctrl Pts',(1.9223538064847,-1.,0.452719478359356));
#23859=CARTESIAN_POINT('Ctrl Pts',(1.9223538064847,1.,0.452719478359356));
#23860=CARTESIAN_POINT('Ctrl Pts',(1.91718342555717,-1.,0.449632260106572));
#23861=CARTESIAN_POINT('Ctrl Pts',(1.91718342555717,1.,0.449632260106572));
#23862=CARTESIAN_POINT('Ctrl Pts',(1.91203699981095,-1.,0.446617343485651));
#23863=CARTESIAN_POINT('Ctrl Pts',(1.91203699981095,1.,0.446617343485651));
#23864=CARTESIAN_POINT('Ctrl Pts',(1.90691756144906,-1.,0.443677556849171));
#23865=CARTESIAN_POINT('Ctrl Pts',(1.90691756144906,1.,0.443677556849171));
#23866=CARTESIAN_POINT('Ctrl Pts',(1.90180124389137,-1.,0.440807833704161));
#23867=CARTESIAN_POINT('Ctrl Pts',(1.90180124389137,1.,0.440807833704161));
#23868=CARTESIAN_POINT('Ctrl Pts',(1.89663648956549,-1.,0.437995003948443));
#23869=CARTESIAN_POINT('Ctrl Pts',(1.89663648956549,1.,0.437995003948443));
#23870=CARTESIAN_POINT('Ctrl Pts',(1.89136993975585,-1.,0.43522566096358));
#23871=CARTESIAN_POINT('Ctrl Pts',(1.89136993975585,1.,0.43522566096358));
#23872=CARTESIAN_POINT('Ctrl Pts',(1.88596913666828,-1.,0.432493038548833));
#23873=CARTESIAN_POINT('Ctrl Pts',(1.88596913666828,1.,0.432493038548833));
#23874=CARTESIAN_POINT('Ctrl Pts',(1.88044229001778,-1.,0.429803062482217));
#23875=CARTESIAN_POINT('Ctrl Pts',(1.88044229001778,1.,0.429803062482217));
#23876=CARTESIAN_POINT('Ctrl Pts',(1.87486989291333,-1.,0.427183828518743));
#23877=CARTESIAN_POINT('Ctrl Pts',(1.87486989291333,1.,0.427183828518743));
#23878=CARTESIAN_POINT('Ctrl Pts',(1.8693780394412,-1.,0.424678177290876));
#23879=CARTESIAN_POINT('Ctrl Pts',(1.8693780394412,1.,0.424678177290876));
#23880=CARTESIAN_POINT('Ctrl Pts',(1.86408083333863,-1.,0.422327307417885));
#23881=CARTESIAN_POINT('Ctrl Pts',(1.86408083333863,1.,0.422327307417885));
#23882=CARTESIAN_POINT('Ctrl Pts',(1.8590328109667,-1.,0.420157287975583));
#23883=CARTESIAN_POINT('Ctrl Pts',(1.8590328109667,1.,0.420157287975583));
#23884=CARTESIAN_POINT('Ctrl Pts',(1.8541763285645,-1.,0.418164129144046));
#23885=CARTESIAN_POINT('Ctrl Pts',(1.8541763285645,1.,0.418164129144046));
#23886=CARTESIAN_POINT('Ctrl Pts',(1.84929312930314,-1.,0.416300022039885));
#23887=CARTESIAN_POINT('Ctrl Pts',(1.84929312930314,1.,0.416300022039885));
#23888=CARTESIAN_POINT('Ctrl Pts',(1.84405757074218,-1.,0.414487438255542));
#23889=CARTESIAN_POINT('Ctrl Pts',(1.84405757074218,1.,0.414487438255542));
#23890=CARTESIAN_POINT('Ctrl Pts',(1.8380895347617,-1.,0.412633125322945));
#23891=CARTESIAN_POINT('Ctrl Pts',(1.8380895347617,1.,0.412633125322945));
#23892=CARTESIAN_POINT('Ctrl Pts',(1.83100408895047,-1.,0.410641256301276));
#23893=CARTESIAN_POINT('Ctrl Pts',(1.83100408895047,1.,0.410641256301276));
#23894=CARTESIAN_POINT('Ctrl Pts',(1.82247022677562,-1.,0.408428948106228));
#23895=CARTESIAN_POINT('Ctrl Pts',(1.82247022677562,1.,0.408428948106228));
#23896=CARTESIAN_POINT('Ctrl Pts',(1.81223801812013,-1.,0.405933518407176));
#23897=CARTESIAN_POINT('Ctrl Pts',(1.81223801812013,1.,0.405933518407176));
#23898=CARTESIAN_POINT('Ctrl Pts',(1.80012077173238,-1.,0.403107976163396));
#23899=CARTESIAN_POINT('Ctrl Pts',(1.80012077173238,1.,0.403107976163396));
#23900=CARTESIAN_POINT('Ctrl Pts',(1.78598826343754,-1.,0.399919403774156));
#23901=CARTESIAN_POINT('Ctrl Pts',(1.78598826343754,1.,0.399919403774156));
#23902=CARTESIAN_POINT('Ctrl Pts',(1.76975560043442,-1.,0.396346196110688));
#23903=CARTESIAN_POINT('Ctrl Pts',(1.76975560043442,1.,0.396346196110688));
#23904=CARTESIAN_POINT('Ctrl Pts',(1.75137405310193,-1.,0.392375812285396));
#23905=CARTESIAN_POINT('Ctrl Pts',(1.75137405310193,1.,0.392375812285396));
#23906=CARTESIAN_POINT('Ctrl Pts',(1.73493170972829,-1.,0.388877023502615));
#23907=CARTESIAN_POINT('Ctrl Pts',(1.73493170972829,1.,0.388877023502615));
#23908=CARTESIAN_POINT('Ctrl Pts',(1.72162022244582,-1.,0.386070790323281));
#23909=CARTESIAN_POINT('Ctrl Pts',(1.72162022244582,1.,0.386070790323281));
#23910=CARTESIAN_POINT('Ctrl Pts',(1.71231062891398,-1.,0.384119047314215));
#23911=CARTESIAN_POINT('Ctrl Pts',(1.71231062891398,1.,0.384119047314215));
#23912=CARTESIAN_POINT('Ctrl Pts',(1.7075470150345,-1.,0.383122945602004));
#23913=CARTESIAN_POINT('Ctrl Pts',(1.7075470150345,1.,0.383122945602004));
#23914=CARTESIAN_POINT('',(1.7075470150345,1.,0.383122945602004));
#23915=CARTESIAN_POINT('',(1.7075470150345,0.,0.383122945602005));
#23916=CARTESIAN_POINT('',(2.11275013067528,1.,0.613422273260091));
#23917=CARTESIAN_POINT('Ctrl Pts',(2.11275013067528,1.,0.613422273260091));
#23918=CARTESIAN_POINT('Ctrl Pts',(2.11187554260142,1.,0.61246736556225));
#23919=CARTESIAN_POINT('Ctrl Pts',(2.11012443807661,1.,0.610560911691114));
#23920=CARTESIAN_POINT('Ctrl Pts',(2.10749199615859,1.,0.607711315456826));
#23921=CARTESIAN_POINT('Ctrl Pts',(2.10397049887709,1.,0.603932030738212));
#23922=CARTESIAN_POINT('Ctrl Pts',(2.09954930865331,1.,0.599241616422144));
#23923=CARTESIAN_POINT('Ctrl Pts',(2.09510876220501,1.,0.594585006052824));
#23924=CARTESIAN_POINT('Ctrl Pts',(2.09064881812053,1.,0.58996236540319));
#23925=CARTESIAN_POINT('Ctrl Pts',(2.086169437277,1.,0.585373918990895));
#23926=CARTESIAN_POINT('Ctrl Pts',(2.08167059018138,1.,0.580819952107257));
#23927=CARTESIAN_POINT('Ctrl Pts',(2.07715226767361,1.,0.576300797416275));
#23928=CARTESIAN_POINT('Ctrl Pts',(2.07261449292757,1.,0.571816823242411));
#23929=CARTESIAN_POINT('Ctrl Pts',(2.06805732997383,1.,0.56736842118123));
#23930=CARTESIAN_POINT('Ctrl Pts',(2.06348090160697,1.,0.562955993082574));
#23931=CARTESIAN_POINT('Ctrl Pts',(2.05888537756571,1.,0.558579940185468));
#23932=CARTESIAN_POINT('Ctrl Pts',(2.05427091604482,1.,0.55424065746411));
#23933=CARTESIAN_POINT('Ctrl Pts',(2.04963761077974,1.,0.549938525150342));
#23934=CARTESIAN_POINT('Ctrl Pts',(2.0449854471456,1.,0.545673903817349));
#23935=CARTESIAN_POINT('Ctrl Pts',(2.0403142269048,1.,0.54144712061552));
#23936=CARTESIAN_POINT('Ctrl Pts',(2.03562362953993,1.,0.537258489833135));
#23937=CARTESIAN_POINT('Ctrl Pts',(2.03091336214401,1.,0.533108355132905));
#23938=CARTESIAN_POINT('Ctrl Pts',(2.02618329083289,1.,0.528997127241911));
#23939=CARTESIAN_POINT('Ctrl Pts',(2.02143356304712,1.,0.524925318333519));
#23940=CARTESIAN_POINT('Ctrl Pts',(2.01666477917305,1.,0.520893590399429));
#23941=CARTESIAN_POINT('Ctrl Pts',(2.01187773939257,1.,0.516902681728733));
#23942=CARTESIAN_POINT('Ctrl Pts',(2.00707309946955,1.,0.512953306961814));
#23943=CARTESIAN_POINT('Ctrl Pts',(2.00225107134733,1.,0.509046069886152));
#23944=CARTESIAN_POINT('Ctrl Pts',(1.99741107463567,1.,0.505181361323011));
#23945=CARTESIAN_POINT('Ctrl Pts',(1.9925514912615,1.,0.501359287727129));
#23946=CARTESIAN_POINT('Ctrl Pts',(1.98767044752929,1.,0.497579909545564));
#23947=CARTESIAN_POINT('Ctrl Pts',(1.9827665876182,1.,0.493843476541493));
#23948=CARTESIAN_POINT('Ctrl Pts',(1.97783973019229,1.,0.490150627860955));
#23949=CARTESIAN_POINT('Ctrl Pts',(1.97289186263272,1.,0.486502692907661));
#23950=CARTESIAN_POINT('Ctrl Pts',(1.96792703422358,1.,0.482901662120687));
#23951=CARTESIAN_POINT('Ctrl Pts',(1.96294933055938,1.,0.479349583074846));
#23952=CARTESIAN_POINT('Ctrl Pts',(1.95796111148175,1.,0.475848034683172));
#23953=CARTESIAN_POINT('Ctrl Pts',(1.95296148278136,1.,0.47239767226408));
#23954=CARTESIAN_POINT('Ctrl Pts',(1.94794381136524,1.,0.468997482913158));
#23955=CARTESIAN_POINT('Ctrl Pts',(1.94289794196205,1.,0.465645462026065));
#23956=CARTESIAN_POINT('Ctrl Pts',(1.93781486640834,1.,0.462340031009087));
#23957=CARTESIAN_POINT('Ctrl Pts',(1.93269066517936,1.,0.459081234547932));
#23958=CARTESIAN_POINT('Ctrl Pts',(1.92753067150461,1.,0.455872005174336));
#23959=CARTESIAN_POINT('Ctrl Pts',(1.9223538064847,1.,0.452719478359356));
#23960=CARTESIAN_POINT('Ctrl Pts',(1.91718342555717,1.,0.449632260106572));
#23961=CARTESIAN_POINT('Ctrl Pts',(1.91203699981095,1.,0.446617343485651));
#23962=CARTESIAN_POINT('Ctrl Pts',(1.90691756144906,1.,0.443677556849171));
#23963=CARTESIAN_POINT('Ctrl Pts',(1.90180124389137,1.,0.440807833704161));
#23964=CARTESIAN_POINT('Ctrl Pts',(1.89663648956549,1.,0.437995003948443));
#23965=CARTESIAN_POINT('Ctrl Pts',(1.89136993975585,1.,0.43522566096358));
#23966=CARTESIAN_POINT('Ctrl Pts',(1.88596913666828,1.,0.432493038548833));
#23967=CARTESIAN_POINT('Ctrl Pts',(1.88044229001778,1.,0.429803062482217));
#23968=CARTESIAN_POINT('Ctrl Pts',(1.87486989291333,1.,0.427183828518743));
#23969=CARTESIAN_POINT('Ctrl Pts',(1.8693780394412,1.,0.424678177290876));
#23970=CARTESIAN_POINT('Ctrl Pts',(1.86408083333863,1.,0.422327307417885));
#23971=CARTESIAN_POINT('Ctrl Pts',(1.8590328109667,1.,0.420157287975583));
#23972=CARTESIAN_POINT('Ctrl Pts',(1.8541763285645,1.,0.418164129144046));
#23973=CARTESIAN_POINT('Ctrl Pts',(1.84929312930314,1.,0.416300022039885));
#23974=CARTESIAN_POINT('Ctrl Pts',(1.84405757074218,1.,0.414487438255542));
#23975=CARTESIAN_POINT('Ctrl Pts',(1.8380895347617,1.,0.412633125322945));
#23976=CARTESIAN_POINT('Ctrl Pts',(1.83100408895047,1.,0.410641256301276));
#23977=CARTESIAN_POINT('Ctrl Pts',(1.82247022677562,1.,0.408428948106228));
#23978=CARTESIAN_POINT('Ctrl Pts',(1.81223801812013,1.,0.405933518407176));
#23979=CARTESIAN_POINT('Ctrl Pts',(1.80012077173238,1.,0.403107976163396));
#23980=CARTESIAN_POINT('Ctrl Pts',(1.78598826343754,1.,0.399919403774156));
#23981=CARTESIAN_POINT('Ctrl Pts',(1.76975560043442,1.,0.396346196110688));
#23982=CARTESIAN_POINT('Ctrl Pts',(1.75137405310193,1.,0.392375812285396));
#23983=CARTESIAN_POINT('Ctrl Pts',(1.73493170972829,1.,0.388877023502615));
#23984=CARTESIAN_POINT('Ctrl Pts',(1.72162022244582,1.,0.386070790323281));
#23985=CARTESIAN_POINT('Ctrl Pts',(1.71231062891398,1.,0.384119047314215));
#23986=CARTESIAN_POINT('Ctrl Pts',(1.7075470150345,1.,0.383122945602004));
#23987=CARTESIAN_POINT('',(2.11275013067528,0.,0.613422273260091));
#23988=CARTESIAN_POINT('Origin',(2.0698113262342,0.,0.745574324794401));
#23989=CARTESIAN_POINT('',(2.0698113262342,1.,0.745574324794401));
#23990=CARTESIAN_POINT('',(2.11275013067528,1.,0.613422273260091));
#23991=CARTESIAN_POINT('',(2.0698113262342,0.,0.745574324794401));
#23992=CARTESIAN_POINT('Ctrl Pts',(1.60662857109684,-1.,0.693717979106306));
#23993=CARTESIAN_POINT('Ctrl Pts',(1.60662857109684,1.,0.693717979106306));
#23994=CARTESIAN_POINT('Ctrl Pts',(1.61106790958151,-1.,0.695712097881194));
#23995=CARTESIAN_POINT('Ctrl Pts',(1.61106790958151,1.,0.695712097881194));
#23996=CARTESIAN_POINT('Ctrl Pts',(1.61974673472612,-1.,0.699605146405088));
#23997=CARTESIAN_POINT('Ctrl Pts',(1.61974673472612,1.,0.699605146405088));
#23998=CARTESIAN_POINT('Ctrl Pts',(1.63216541664676,-1.,0.705159151988319));
#23999=CARTESIAN_POINT('Ctrl Pts',(1.63216541664676,1.,0.705159151988319));
#24000=CARTESIAN_POINT('Ctrl Pts',(1.64752408832016,-1.,0.711993139355394));
#24001=CARTESIAN_POINT('Ctrl Pts',(1.64752408832016,1.,0.711993139355394));
#24002=CARTESIAN_POINT('Ctrl Pts',(1.6647288055568,-1.,0.719585433804282));
#24003=CARTESIAN_POINT('Ctrl Pts',(1.6647288055568,1.,0.719585433804282));
#24004=CARTESIAN_POINT('Ctrl Pts',(1.67996158455503,-1.,0.726235967997433));
#24005=CARTESIAN_POINT('Ctrl Pts',(1.67996158455503,1.,0.726235967997433));
#24006=CARTESIAN_POINT('Ctrl Pts',(1.69326921975743,-1.,0.731963238697195));
#24007=CARTESIAN_POINT('Ctrl Pts',(1.69326921975743,1.,0.731963238697195));
#24008=CARTESIAN_POINT('Ctrl Pts',(1.70473309006121,-1.,0.736799665724771));
#24009=CARTESIAN_POINT('Ctrl Pts',(1.70473309006121,1.,0.736799665724771));
#24010=CARTESIAN_POINT('Ctrl Pts',(1.71447789751927,-1.,0.740795162032088));
#24011=CARTESIAN_POINT('Ctrl Pts',(1.71447789751927,1.,0.740795162032088));
#24012=CARTESIAN_POINT('Ctrl Pts',(1.7226822991693,-1.,0.744021445433765));
#24013=CARTESIAN_POINT('Ctrl Pts',(1.7226822991693,1.,0.744021445433765));
#24014=CARTESIAN_POINT('Ctrl Pts',(1.72958533647399,-1.,0.746574710096437));
#24015=CARTESIAN_POINT('Ctrl Pts',(1.72958533647399,1.,0.746574710096437));
#24016=CARTESIAN_POINT('Ctrl Pts',(1.73550351679848,-1.,0.748582462954855));
#24017=CARTESIAN_POINT('Ctrl Pts',(1.73550351679848,1.,0.748582462954855));
#24018=CARTESIAN_POINT('Ctrl Pts',(1.74080458266705,-1.,0.750193435979541));
#24019=CARTESIAN_POINT('Ctrl Pts',(1.74080458266705,1.,0.750193435979541));
#24020=CARTESIAN_POINT('Ctrl Pts',(1.74585086852298,-1.,0.751555614163629));
#24021=CARTESIAN_POINT('Ctrl Pts',(1.74585086852298,1.,0.751555614163629));
#24022=CARTESIAN_POINT('Ctrl Pts',(1.75095139468809,-1.,0.752797683531377));
#24023=CARTESIAN_POINT('Ctrl Pts',(1.75095139468809,1.,0.752797683531377));
#24024=CARTESIAN_POINT('Ctrl Pts',(1.75631083600175,-1.,0.75400925402848));
#24025=CARTESIAN_POINT('Ctrl Pts',(1.75631083600175,1.,0.75400925402848));
#24026=CARTESIAN_POINT('Ctrl Pts',(1.7619781724032,-1.,0.755220979975262));
#24027=CARTESIAN_POINT('Ctrl Pts',(1.7619781724032,1.,0.755220979975262));
#24028=CARTESIAN_POINT('Ctrl Pts',(1.76789396003141,-1.,0.756421896028403));
#24029=CARTESIAN_POINT('Ctrl Pts',(1.76789396003141,1.,0.756421896028403));
#24030=CARTESIAN_POINT('Ctrl Pts',(1.77394167108342,-1.,0.757578264077238));
#24031=CARTESIAN_POINT('Ctrl Pts',(1.77394167108342,1.,0.757578264077238));
#24032=CARTESIAN_POINT('Ctrl Pts',(1.77999411220912,-1.,0.75865062667738));
#24033=CARTESIAN_POINT('Ctrl Pts',(1.77999411220912,1.,0.75865062667738));
#24034=CARTESIAN_POINT('Ctrl Pts',(1.78596964884526,-1.,0.759614401109868));
#24035=CARTESIAN_POINT('Ctrl Pts',(1.78596964884526,1.,0.759614401109868));
#24036=CARTESIAN_POINT('Ctrl Pts',(1.79185815610802,-1.,0.760469555880425));
#24037=CARTESIAN_POINT('Ctrl Pts',(1.79185815610802,1.,0.760469555880425));
#24038=CARTESIAN_POINT('Ctrl Pts',(1.79768986997735,-1.,0.761229695230359));
#24039=CARTESIAN_POINT('Ctrl Pts',(1.79768986997735,1.,0.761229695230359));
#24040=CARTESIAN_POINT('Ctrl Pts',(1.80351583877334,-1.,0.761915336443516));
#24041=CARTESIAN_POINT('Ctrl Pts',(1.80351583877334,1.,0.761915336443516));
#24042=CARTESIAN_POINT('Ctrl Pts',(1.80938551463989,-1.,0.762546129464036));
#24043=CARTESIAN_POINT('Ctrl Pts',(1.80938551463989,1.,0.762546129464036));
#24044=CARTESIAN_POINT('Ctrl Pts',(1.81532118405566,-1.,0.763132003836783));
#24045=CARTESIAN_POINT('Ctrl Pts',(1.81532118405566,1.,0.763132003836783));
#24046=CARTESIAN_POINT('Ctrl Pts',(1.82131873145297,-1.,0.763673465462854));
#24047=CARTESIAN_POINT('Ctrl Pts',(1.82131873145297,1.,0.763673465462854));
#24048=CARTESIAN_POINT('Ctrl Pts',(1.8273599120008,-1.,0.764165902606056));
#24049=CARTESIAN_POINT('Ctrl Pts',(1.8273599120008,1.,0.764165902606056));
#24050=CARTESIAN_POINT('Ctrl Pts',(1.8334207722714,-1.,0.764602549687846));
#24051=CARTESIAN_POINT('Ctrl Pts',(1.8334207722714,1.,0.764602549687846));
#24052=CARTESIAN_POINT('Ctrl Pts',(1.83948181064823,-1.,0.764978057881688));
#24053=CARTESIAN_POINT('Ctrl Pts',(1.83948181064823,1.,0.764978057881688));
#24054=CARTESIAN_POINT('Ctrl Pts',(1.8455369887591,-1.,0.765291664861972));
#24055=CARTESIAN_POINT('Ctrl Pts',(1.8455369887591,1.,0.765291664861972));
#24056=CARTESIAN_POINT('Ctrl Pts',(1.85158945130054,-1.,0.765545710619023));
#24057=CARTESIAN_POINT('Ctrl Pts',(1.85158945130054,1.,0.765545710619023));
#24058=CARTESIAN_POINT('Ctrl Pts',(1.85764741390391,-1.,0.765744212909305));
#24059=CARTESIAN_POINT('Ctrl Pts',(1.85764741390391,1.,0.765744212909305));
#24060=CARTESIAN_POINT('Ctrl Pts',(1.86372027063314,-1.,0.765891519092557));
#24061=CARTESIAN_POINT('Ctrl Pts',(1.86372027063314,1.,0.765891519092557));
#24062=CARTESIAN_POINT('Ctrl Pts',(1.86981398314345,-1.,0.765990708546112));
#24063=CARTESIAN_POINT('Ctrl Pts',(1.86981398314345,1.,0.765990708546112));
#24064=CARTESIAN_POINT('Ctrl Pts',(1.87592888967886,-1.,0.766042837036759));
#24065=CARTESIAN_POINT('Ctrl Pts',(1.87592888967886,1.,0.766042837036759));
#24066=CARTESIAN_POINT('Ctrl Pts',(1.88206215302561,-1.,0.766047794851869));
#24067=CARTESIAN_POINT('Ctrl Pts',(1.88206215302561,1.,0.766047794851869));
#24068=CARTESIAN_POINT('Ctrl Pts',(1.88820926433409,-1.,0.76600483706209));
#24069=CARTESIAN_POINT('Ctrl Pts',(1.88820926433409,1.,0.76600483706209));
#24070=CARTESIAN_POINT('Ctrl Pts',(1.89436577771389,-1.,0.765913193856979));
#24071=CARTESIAN_POINT('Ctrl Pts',(1.89436577771389,1.,0.765913193856979));
#24072=CARTESIAN_POINT('Ctrl Pts',(1.90052930393599,-1.,0.765772772593395));
#24073=CARTESIAN_POINT('Ctrl Pts',(1.90052930393599,1.,0.765772772593395));
#24074=CARTESIAN_POINT('Ctrl Pts',(1.90669961402362,-1.,0.765584196937937));
#24075=CARTESIAN_POINT('Ctrl Pts',(1.90669961402362,1.,0.765584196937937));
#24076=CARTESIAN_POINT('Ctrl Pts',(1.91287765805174,-1.,0.765348465884739));
#24077=CARTESIAN_POINT('Ctrl Pts',(1.91287765805174,1.,0.765348465884739));
#24078=CARTESIAN_POINT('Ctrl Pts',(1.91906491634197,-1.,0.765066729667095));
#24079=CARTESIAN_POINT('Ctrl Pts',(1.91906491634197,1.,0.765066729667095));
#24080=CARTESIAN_POINT('Ctrl Pts',(1.92526263537041,-1.,0.764740025488189));
#24081=CARTESIAN_POINT('Ctrl Pts',(1.92526263537041,1.,0.764740025488189));
#24082=CARTESIAN_POINT('Ctrl Pts',(1.93147105496367,-1.,0.76436901067389));
#24083=CARTESIAN_POINT('Ctrl Pts',(1.93147105496367,1.,0.76436901067389));
#24084=CARTESIAN_POINT('Ctrl Pts',(1.93768964875867,-1.,0.763954049121394));
#24085=CARTESIAN_POINT('Ctrl Pts',(1.93768964875867,1.,0.763954049121394));
#24086=CARTESIAN_POINT('Ctrl Pts',(1.94391746617626,-1.,0.763495333538581));
#24087=CARTESIAN_POINT('Ctrl Pts',(1.94391746617626,1.,0.763495333538581));
#24088=CARTESIAN_POINT('Ctrl Pts',(1.95015342590025,-1.,0.762992990878774));
#24089=CARTESIAN_POINT('Ctrl Pts',(1.95015342590025,1.,0.762992990878774));
#24090=CARTESIAN_POINT('Ctrl Pts',(1.95639665309893,-1.,0.762447203806264));
#24091=CARTESIAN_POINT('Ctrl Pts',(1.95639665309893,1.,0.762447203806264));
#24092=CARTESIAN_POINT('Ctrl Pts',(1.96264672744229,-1.,0.761858300014575));
#24093=CARTESIAN_POINT('Ctrl Pts',(1.96264672744229,1.,0.761858300014575));
#24094=CARTESIAN_POINT('Ctrl Pts',(1.96890351582545,-1.,0.761226690483986));
#24095=CARTESIAN_POINT('Ctrl Pts',(1.96890351582545,1.,0.761226690483986));
#24096=CARTESIAN_POINT('Ctrl Pts',(1.97516705321521,-1.,0.760552825409856));
#24097=CARTESIAN_POINT('Ctrl Pts',(1.97516705321521,1.,0.760552825409856));
#24098=CARTESIAN_POINT('Ctrl Pts',(1.98143741418156,-1.,0.759837147452135));
#24099=CARTESIAN_POINT('Ctrl Pts',(1.98143741418156,1.,0.759837147452135));
#24100=CARTESIAN_POINT('Ctrl Pts',(1.98771456680806,-1.,0.759080037802243));
#24101=CARTESIAN_POINT('Ctrl Pts',(1.98771456680806,1.,0.759080037802243));
#24102=CARTESIAN_POINT('Ctrl Pts',(1.9939983109871,-1.,0.758281796766377));
#24103=CARTESIAN_POINT('Ctrl Pts',(1.9939983109871,1.,0.758281796766377));
#24104=CARTESIAN_POINT('Ctrl Pts',(2.00028834739072,-1.,0.757442676862342));
#24105=CARTESIAN_POINT('Ctrl Pts',(2.00028834739072,1.,0.757442676862342));
#24106=CARTESIAN_POINT('Ctrl Pts',(2.00658431587682,-1.,0.756562904646496));
#24107=CARTESIAN_POINT('Ctrl Pts',(2.00658431587682,1.,0.756562904646496));
#24108=CARTESIAN_POINT('Ctrl Pts',(2.01288584328149,-1.,0.755642704958101));
#24109=CARTESIAN_POINT('Ctrl Pts',(2.01288584328149,1.,0.755642704958101));
#24110=CARTESIAN_POINT('Ctrl Pts',(2.01919259406003,-1.,0.75468233072352));
#24111=CARTESIAN_POINT('Ctrl Pts',(2.01919259406003,1.,0.75468233072352));
#24112=CARTESIAN_POINT('Ctrl Pts',(2.02550428623587,-1.,0.753682061113766));
#24113=CARTESIAN_POINT('Ctrl Pts',(2.02550428623587,1.,0.753682061113766));
#24114=CARTESIAN_POINT('Ctrl Pts',(2.03182068456467,-1.,0.752642180488104));
#24115=CARTESIAN_POINT('Ctrl Pts',(2.03182068456467,1.,0.752642180488104));
#24116=CARTESIAN_POINT('Ctrl Pts',(2.03814160092173,-1.,0.751562963361384));
#24117=CARTESIAN_POINT('Ctrl Pts',(2.03814160092173,1.,0.751562963361384));
#24118=CARTESIAN_POINT('Ctrl Pts',(2.04446689147754,-1.,0.750444657874758));
#24119=CARTESIAN_POINT('Ctrl Pts',(2.04446689147754,1.,0.750444657874758));
#24120=CARTESIAN_POINT('Ctrl Pts',(2.05079645591606,-1.,0.749287468663053));
#24121=CARTESIAN_POINT('Ctrl Pts',(2.05079645591606,1.,0.749287468663053));
#24122=CARTESIAN_POINT('Ctrl Pts',(2.05713023030263,-1.,0.748091554181101));
#24123=CARTESIAN_POINT('Ctrl Pts',(2.05713023030263,1.,0.748091554181101));
#24124=CARTESIAN_POINT('Ctrl Pts',(2.06220058927162,-1.,0.747103932785504));
#24125=CARTESIAN_POINT('Ctrl Pts',(2.06220058927162,1.,0.747103932785504));
#24126=CARTESIAN_POINT('Ctrl Pts',(2.06600523016401,-1.,0.746345871542696));
#24127=CARTESIAN_POINT('Ctrl Pts',(2.06600523016401,1.,0.746345871542696));
#24128=CARTESIAN_POINT('Ctrl Pts',(2.06854248895575,-1.,0.74583279137781));
#24129=CARTESIAN_POINT('Ctrl Pts',(2.06854248895575,1.,0.74583279137781));
#24130=CARTESIAN_POINT('Ctrl Pts',(2.0698113262342,-1.,0.745574324794401));
#24131=CARTESIAN_POINT('Ctrl Pts',(2.0698113262342,1.,0.745574324794401));
#24132=CARTESIAN_POINT('',(1.60662857109684,1.,0.693717979106306));
#24133=CARTESIAN_POINT('Ctrl Pts',(1.60662857109684,1.,0.693717979106306));
#24134=CARTESIAN_POINT('Ctrl Pts',(1.61106790958151,1.,0.695712097881194));
#24135=CARTESIAN_POINT('Ctrl Pts',(1.61974673472612,1.,0.699605146405088));
#24136=CARTESIAN_POINT('Ctrl Pts',(1.63216541664676,1.,0.705159151988319));
#24137=CARTESIAN_POINT('Ctrl Pts',(1.64752408832016,1.,0.711993139355394));
#24138=CARTESIAN_POINT('Ctrl Pts',(1.6647288055568,1.,0.719585433804282));
#24139=CARTESIAN_POINT('Ctrl Pts',(1.67996158455503,1.,0.726235967997433));
#24140=CARTESIAN_POINT('Ctrl Pts',(1.69326921975743,1.,0.731963238697195));
#24141=CARTESIAN_POINT('Ctrl Pts',(1.70473309006121,1.,0.736799665724771));
#24142=CARTESIAN_POINT('Ctrl Pts',(1.71447789751927,1.,0.740795162032088));
#24143=CARTESIAN_POINT('Ctrl Pts',(1.7226822991693,1.,0.744021445433765));
#24144=CARTESIAN_POINT('Ctrl Pts',(1.72958533647399,1.,0.746574710096437));
#24145=CARTESIAN_POINT('Ctrl Pts',(1.73550351679848,1.,0.748582462954855));
#24146=CARTESIAN_POINT('Ctrl Pts',(1.74080458266705,1.,0.750193435979541));
#24147=CARTESIAN_POINT('Ctrl Pts',(1.74585086852298,1.,0.751555614163629));
#24148=CARTESIAN_POINT('Ctrl Pts',(1.75095139468809,1.,0.752797683531377));
#24149=CARTESIAN_POINT('Ctrl Pts',(1.75631083600175,1.,0.75400925402848));
#24150=CARTESIAN_POINT('Ctrl Pts',(1.7619781724032,1.,0.755220979975262));
#24151=CARTESIAN_POINT('Ctrl Pts',(1.76789396003141,1.,0.756421896028403));
#24152=CARTESIAN_POINT('Ctrl Pts',(1.77394167108342,1.,0.757578264077238));
#24153=CARTESIAN_POINT('Ctrl Pts',(1.77999411220912,1.,0.75865062667738));
#24154=CARTESIAN_POINT('Ctrl Pts',(1.78596964884526,1.,0.759614401109868));
#24155=CARTESIAN_POINT('Ctrl Pts',(1.79185815610802,1.,0.760469555880425));
#24156=CARTESIAN_POINT('Ctrl Pts',(1.79768986997735,1.,0.761229695230359));
#24157=CARTESIAN_POINT('Ctrl Pts',(1.80351583877334,1.,0.761915336443516));
#24158=CARTESIAN_POINT('Ctrl Pts',(1.80938551463989,1.,0.762546129464036));
#24159=CARTESIAN_POINT('Ctrl Pts',(1.81532118405566,1.,0.763132003836783));
#24160=CARTESIAN_POINT('Ctrl Pts',(1.82131873145297,1.,0.763673465462854));
#24161=CARTESIAN_POINT('Ctrl Pts',(1.8273599120008,1.,0.764165902606056));
#24162=CARTESIAN_POINT('Ctrl Pts',(1.8334207722714,1.,0.764602549687846));
#24163=CARTESIAN_POINT('Ctrl Pts',(1.83948181064823,1.,0.764978057881688));
#24164=CARTESIAN_POINT('Ctrl Pts',(1.8455369887591,1.,0.765291664861972));
#24165=CARTESIAN_POINT('Ctrl Pts',(1.85158945130054,1.,0.765545710619023));
#24166=CARTESIAN_POINT('Ctrl Pts',(1.85764741390391,1.,0.765744212909305));
#24167=CARTESIAN_POINT('Ctrl Pts',(1.86372027063314,1.,0.765891519092557));
#24168=CARTESIAN_POINT('Ctrl Pts',(1.86981398314345,1.,0.765990708546112));
#24169=CARTESIAN_POINT('Ctrl Pts',(1.87592888967886,1.,0.766042837036759));
#24170=CARTESIAN_POINT('Ctrl Pts',(1.88206215302561,1.,0.766047794851869));
#24171=CARTESIAN_POINT('Ctrl Pts',(1.88820926433409,1.,0.76600483706209));
#24172=CARTESIAN_POINT('Ctrl Pts',(1.89436577771389,1.,0.765913193856979));
#24173=CARTESIAN_POINT('Ctrl Pts',(1.90052930393599,1.,0.765772772593395));
#24174=CARTESIAN_POINT('Ctrl Pts',(1.90669961402362,1.,0.765584196937937));
#24175=CARTESIAN_POINT('Ctrl Pts',(1.91287765805174,1.,0.765348465884739));
#24176=CARTESIAN_POINT('Ctrl Pts',(1.91906491634197,1.,0.765066729667095));
#24177=CARTESIAN_POINT('Ctrl Pts',(1.92526263537041,1.,0.764740025488189));
#24178=CARTESIAN_POINT('Ctrl Pts',(1.93147105496367,1.,0.76436901067389));
#24179=CARTESIAN_POINT('Ctrl Pts',(1.93768964875867,1.,0.763954049121394));
#24180=CARTESIAN_POINT('Ctrl Pts',(1.94391746617626,1.,0.763495333538581));
#24181=CARTESIAN_POINT('Ctrl Pts',(1.95015342590025,1.,0.762992990878774));
#24182=CARTESIAN_POINT('Ctrl Pts',(1.95639665309893,1.,0.762447203806264));
#24183=CARTESIAN_POINT('Ctrl Pts',(1.96264672744229,1.,0.761858300014575));
#24184=CARTESIAN_POINT('Ctrl Pts',(1.96890351582545,1.,0.761226690483986));
#24185=CARTESIAN_POINT('Ctrl Pts',(1.97516705321521,1.,0.760552825409856));
#24186=CARTESIAN_POINT('Ctrl Pts',(1.98143741418156,1.,0.759837147452135));
#24187=CARTESIAN_POINT('Ctrl Pts',(1.98771456680806,1.,0.759080037802243));
#24188=CARTESIAN_POINT('Ctrl Pts',(1.9939983109871,1.,0.758281796766377));
#24189=CARTESIAN_POINT('Ctrl Pts',(2.00028834739072,1.,0.757442676862342));
#24190=CARTESIAN_POINT('Ctrl Pts',(2.00658431587682,1.,0.756562904646496));
#24191=CARTESIAN_POINT('Ctrl Pts',(2.01288584328149,1.,0.755642704958101));
#24192=CARTESIAN_POINT('Ctrl Pts',(2.01919259406003,1.,0.75468233072352));
#24193=CARTESIAN_POINT('Ctrl Pts',(2.02550428623587,1.,0.753682061113766));
#24194=CARTESIAN_POINT('Ctrl Pts',(2.03182068456467,1.,0.752642180488104));
#24195=CARTESIAN_POINT('Ctrl Pts',(2.03814160092173,1.,0.751562963361384));
#24196=CARTESIAN_POINT('Ctrl Pts',(2.04446689147754,1.,0.750444657874758));
#24197=CARTESIAN_POINT('Ctrl Pts',(2.05079645591606,1.,0.749287468663053));
#24198=CARTESIAN_POINT('Ctrl Pts',(2.05713023030263,1.,0.748091554181101));
#24199=CARTESIAN_POINT('Ctrl Pts',(2.06220058927162,1.,0.747103932785504));
#24200=CARTESIAN_POINT('Ctrl Pts',(2.06600523016401,1.,0.746345871542696));
#24201=CARTESIAN_POINT('Ctrl Pts',(2.06854248895575,1.,0.74583279137781));
#24202=CARTESIAN_POINT('Ctrl Pts',(2.0698113262342,1.,0.745574324794401));
#24203=CARTESIAN_POINT('',(1.60662857109684,0.,0.693717979106305));
#24204=CARTESIAN_POINT('Origin',(0.,0.,0.));
#24205=CARTESIAN_POINT('',(1.5055822144029,1.,0.892032620296856));
#24206=CARTESIAN_POINT('Origin',(0.,1.,0.));
#24207=CARTESIAN_POINT('',(1.5055822144029,0.,0.892032620296855));
#24208=CARTESIAN_POINT('Ctrl Pts',(1.81978687191668,-1.,1.23627494547115));
#24209=CARTESIAN_POINT('Ctrl Pts',(1.81978687191668,1.,1.23627494547115));
#24210=CARTESIAN_POINT('Ctrl Pts',(1.81925017193666,-1.,1.23509651170476));
#24211=CARTESIAN_POINT('Ctrl Pts',(1.81925017193666,1.,1.23509651170476));
#24212=CARTESIAN_POINT('Ctrl Pts',(1.81817389921279,-1.,1.2327422452705));
#24213=CARTESIAN_POINT('Ctrl Pts',(1.81817389921279,1.,1.2327422452705));
#24214=CARTESIAN_POINT('Ctrl Pts',(1.8165508718364,-1.,1.2292186489137));
#24215=CARTESIAN_POINT('Ctrl Pts',(1.8165508718364,1.,1.2292186489137));
#24216=CARTESIAN_POINT('Ctrl Pts',(1.81436959210434,-1.,1.2245361330495));
#24217=CARTESIAN_POINT('Ctrl Pts',(1.81436959210434,1.,1.2245361330495));
#24218=CARTESIAN_POINT('Ctrl Pts',(1.81161420806656,-1.,1.21870906103557));
#24219=CARTESIAN_POINT('Ctrl Pts',(1.81161420806656,1.,1.21870906103557));
#24220=CARTESIAN_POINT('Ctrl Pts',(1.80882996917129,-1.,1.21290815708314));
#24221=CARTESIAN_POINT('Ctrl Pts',(1.80882996917129,1.,1.21290815708314));
#24222=CARTESIAN_POINT('Ctrl Pts',(1.80601678480707,-1.,1.20713356605475));
#24223=CARTESIAN_POINT('Ctrl Pts',(1.80601678480707,1.,1.20713356605475));
#24224=CARTESIAN_POINT('Ctrl Pts',(1.80317454838603,-1.,1.20138548938974));
#24225=CARTESIAN_POINT('Ctrl Pts',(1.80317454838603,1.,1.20138548938974));
#24226=CARTESIAN_POINT('Ctrl Pts',(1.80030314369879,-1.,1.19566418930242));
#24227=CARTESIAN_POINT('Ctrl Pts',(1.80030314369879,1.,1.19566418930242));
#24228=CARTESIAN_POINT('Ctrl Pts',(1.79740245923478,-1.,1.18996997934445));
#24229=CARTESIAN_POINT('Ctrl Pts',(1.79740245923478,1.,1.18996997934445));
#24230=CARTESIAN_POINT('Ctrl Pts',(1.79447240321515,-1.,1.18430321697432));
#24231=CARTESIAN_POINT('Ctrl Pts',(1.79447240321515,1.,1.18430321697432));
#24232=CARTESIAN_POINT('Ctrl Pts',(1.79151291552689,-1.,1.17866429440809));
#24233=CARTESIAN_POINT('Ctrl Pts',(1.79151291552689,1.,1.17866429440809));
#24234=CARTESIAN_POINT('Ctrl Pts',(1.78852398877616,-1.,1.17305363177328));
#24235=CARTESIAN_POINT('Ctrl Pts',(1.78852398877616,1.,1.17305363177328));
#24236=CARTESIAN_POINT('Ctrl Pts',(1.78550566040443,-1.,1.16747166312303));
#24237=CARTESIAN_POINT('Ctrl Pts',(1.78550566040443,1.,1.16747166312303));
#24238=CARTESIAN_POINT('Ctrl Pts',(1.78245795881009,-1.,1.16191881298499));
#24239=CARTESIAN_POINT('Ctrl Pts',(1.78245795881009,1.,1.16191881298499));
#24240=CARTESIAN_POINT('Ctrl Pts',(1.77938085564275,-1.,1.15639547194698));
#24241=CARTESIAN_POINT('Ctrl Pts',(1.77938085564275,1.,1.15639547194698));
#24242=CARTESIAN_POINT('Ctrl Pts',(1.7762742255701,-1.,1.15090197841515));
#24243=CARTESIAN_POINT('Ctrl Pts',(1.7762742255701,1.,1.15090197841515));
#24244=CARTESIAN_POINT('Ctrl Pts',(1.77313777896194,-1.,1.1454385822692));
#24245=CARTESIAN_POINT('Ctrl Pts',(1.77313777896194,1.,1.1454385822692));
#24246=CARTESIAN_POINT('Ctrl Pts',(1.76997111386769,-1.,1.14000548336975));
#24247=CARTESIAN_POINT('Ctrl Pts',(1.76997111386769,1.,1.14000548336975));
#24248=CARTESIAN_POINT('Ctrl Pts',(1.76677384551862,-1.,1.1346029180462));
#24249=CARTESIAN_POINT('Ctrl Pts',(1.76677384551862,1.,1.1346029180462));
#24250=CARTESIAN_POINT('Ctrl Pts',(1.7635457196617,-1.,1.12923123555075));
#24251=CARTESIAN_POINT('Ctrl Pts',(1.7635457196617,1.,1.12923123555075));
#24252=CARTESIAN_POINT('Ctrl Pts',(1.76028671825096,-1.,1.12389096855086));
#24253=CARTESIAN_POINT('Ctrl Pts',(1.76028671825096,1.,1.12389096855086));
#24254=CARTESIAN_POINT('Ctrl Pts',(1.75699720772105,-1.,1.11858293216763));
#24255=CARTESIAN_POINT('Ctrl Pts',(1.75699720772105,1.,1.11858293216763));
#24256=CARTESIAN_POINT('Ctrl Pts',(1.7536777209463,-1.,1.11330807582551));
#24257=CARTESIAN_POINT('Ctrl Pts',(1.7536777209463,1.,1.11330807582551));
#24258=CARTESIAN_POINT('Ctrl Pts',(1.7503286607592,-1.,1.10806728183007));
#24259=CARTESIAN_POINT('Ctrl Pts',(1.7503286607592,1.,1.10806728183007));
#24260=CARTESIAN_POINT('Ctrl Pts',(1.74695004214923,-1.,1.10286118991143));
#24261=CARTESIAN_POINT('Ctrl Pts',(1.74695004214923,1.,1.10286118991143));
#24262=CARTESIAN_POINT('Ctrl Pts',(1.74354119236208,-1.,1.09768999241226));
#24263=CARTESIAN_POINT('Ctrl Pts',(1.74354119236208,1.,1.09768999241226));
#24264=CARTESIAN_POINT('Ctrl Pts',(1.74010053962247,-1.,1.09255329056493));
#24265=CARTESIAN_POINT('Ctrl Pts',(1.74010053962247,1.,1.09255329056493));
#24266=CARTESIAN_POINT('Ctrl Pts',(1.73662628326091,-1.,1.08745056285427));
#24267=CARTESIAN_POINT('Ctrl Pts',(1.73662628326091,1.,1.08745056285427));
#24268=CARTESIAN_POINT('Ctrl Pts',(1.73311705663407,-1.,1.08238162784749));
#24269=CARTESIAN_POINT('Ctrl Pts',(1.73311705663407,1.,1.08238162784749));
#24270=CARTESIAN_POINT('Ctrl Pts',(1.72957248977424,-1.,1.0773470373727));
#24271=CARTESIAN_POINT('Ctrl Pts',(1.72957248977424,1.,1.0773470373727));
#24272=CARTESIAN_POINT('Ctrl Pts',(1.72599406198488,-1.,1.07234866990252));
#24273=CARTESIAN_POINT('Ctrl Pts',(1.72599406198488,1.,1.07234866990252));
#24274=CARTESIAN_POINT('Ctrl Pts',(1.72238500928453,-1.,1.06738966975462));
#24275=CARTESIAN_POINT('Ctrl Pts',(1.72238500928453,1.,1.06738966975462));
#24276=CARTESIAN_POINT('Ctrl Pts',(1.71874858456904,-1.,1.06247324680647));
#24277=CARTESIAN_POINT('Ctrl Pts',(1.71874858456904,1.,1.06247324680647));
#24278=CARTESIAN_POINT('Ctrl Pts',(1.7150865442702,-1.,1.05760163192479));
#24279=CARTESIAN_POINT('Ctrl Pts',(1.7150865442702,1.,1.05760163192479));
#24280=CARTESIAN_POINT('Ctrl Pts',(1.71139783543989,-1.,1.05277517202855));
#24281=CARTESIAN_POINT('Ctrl Pts',(1.71139783543989,1.,1.05277517202855));
#24282=CARTESIAN_POINT('Ctrl Pts',(1.70767646263649,-1.,1.04799085404995));
#24283=CARTESIAN_POINT('Ctrl Pts',(1.70767646263649,1.,1.04799085404995));
#24284=CARTESIAN_POINT('Ctrl Pts',(1.70391338707982,-1.,1.04324363334554));
#24285=CARTESIAN_POINT('Ctrl Pts',(1.70391338707982,1.,1.04324363334554));
#24286=CARTESIAN_POINT('Ctrl Pts',(1.70010052930962,-1.,1.03852922490789));
#24287=CARTESIAN_POINT('Ctrl Pts',(1.70010052930962,1.,1.03852922490789));
#24288=CARTESIAN_POINT('Ctrl Pts',(1.69623414782771,-1.,1.03384646003588));
#24289=CARTESIAN_POINT('Ctrl Pts',(1.69623414782771,1.,1.03384646003588));
#24290=CARTESIAN_POINT('Ctrl Pts',(1.69231840863458,-1.,1.02919977579147));
#24291=CARTESIAN_POINT('Ctrl Pts',(1.69231840863458,1.,1.02919977579147));
#24292=CARTESIAN_POINT('Ctrl Pts',(1.68836910178447,-1.,1.02460180535255));
#24293=CARTESIAN_POINT('Ctrl Pts',(1.68836910178447,1.,1.02460180535255));
#24294=CARTESIAN_POINT('Ctrl Pts',(1.68440578021706,-1.,1.02006795074201));
#24295=CARTESIAN_POINT('Ctrl Pts',(1.68440578021706,1.,1.02006795074201));
#24296=CARTESIAN_POINT('Ctrl Pts',(1.68044289894798,-1.,1.01561026162773));
#24297=CARTESIAN_POINT('Ctrl Pts',(1.68044289894798,1.,1.01561026162773));
#24298=CARTESIAN_POINT('Ctrl Pts',(1.67648246776464,-1.,1.01123236493511));
#24299=CARTESIAN_POINT('Ctrl Pts',(1.67648246776464,1.,1.01123236493511));
#24300=CARTESIAN_POINT('Ctrl Pts',(1.67250335383293,-1.,1.00692206696414));
#24301=CARTESIAN_POINT('Ctrl Pts',(1.67250335383293,1.,1.00692206696414));
#24302=CARTESIAN_POINT('Ctrl Pts',(1.66846059277303,-1.,1.00265091003727));
#24303=CARTESIAN_POINT('Ctrl Pts',(1.66846059277303,1.,1.00265091003727));
#24304=CARTESIAN_POINT('Ctrl Pts',(1.66430758030376,-1.,0.998389654952758));
#24305=CARTESIAN_POINT('Ctrl Pts',(1.66430758030376,1.,0.998389654952758));
#24306=CARTESIAN_POINT('Ctrl Pts',(1.66001553809947,-1.,0.994121836661306));
#24307=CARTESIAN_POINT('Ctrl Pts',(1.66001553809947,1.,0.994121836661306));
#24308=CARTESIAN_POINT('Ctrl Pts',(1.65559044289699,-1.,0.989855627854165));
#24309=CARTESIAN_POINT('Ctrl Pts',(1.65559044289699,1.,0.989855627854165));
#24310=CARTESIAN_POINT('Ctrl Pts',(1.65110016612638,-1.,0.985642622920821));
#24311=CARTESIAN_POINT('Ctrl Pts',(1.65110016612638,1.,0.985642622920821));
#24312=CARTESIAN_POINT('Ctrl Pts',(1.64665139190656,-1.,0.981562530939489));
#24313=CARTESIAN_POINT('Ctrl Pts',(1.64665139190656,1.,0.981562530939489));
#24314=CARTESIAN_POINT('Ctrl Pts',(1.64233990826687,-1.,0.977689794119417));
#24315=CARTESIAN_POINT('Ctrl Pts',(1.64233990826687,1.,0.977689794119417));
#24316=CARTESIAN_POINT('Ctrl Pts',(1.63820952658144,-1.,0.974066058287419));
#24317=CARTESIAN_POINT('Ctrl Pts',(1.63820952658144,1.,0.974066058287419));
#24318=CARTESIAN_POINT('Ctrl Pts',(1.63420665729798,-1.,0.970669715997509));
#24319=CARTESIAN_POINT('Ctrl Pts',(1.63420665729798,1.,0.970669715997509));
#24320=CARTESIAN_POINT('Ctrl Pts',(1.63013849959461,-1.,0.967387853230345));
#24321=CARTESIAN_POINT('Ctrl Pts',(1.63013849959461,1.,0.967387853230345));
#24322=CARTESIAN_POINT('Ctrl Pts',(1.62571930670187,-1.,0.964046107040536));
#24323=CARTESIAN_POINT('Ctrl Pts',(1.62571930670187,1.,0.964046107040536));
#24324=CARTESIAN_POINT('Ctrl Pts',(1.62061638140221,-1.,0.960438326101729));
#24325=CARTESIAN_POINT('Ctrl Pts',(1.62061638140221,1.,0.960438326101729));
#24326=CARTESIAN_POINT('Ctrl Pts',(1.61449324337085,-1.,0.956354422920671));
#24327=CARTESIAN_POINT('Ctrl Pts',(1.61449324337085,1.,0.956354422920671));
#24328=CARTESIAN_POINT('Ctrl Pts',(1.60706069896936,-1.,0.951613284356035));
#24329=CARTESIAN_POINT('Ctrl Pts',(1.60706069896936,1.,0.951613284356035));
#24330=CARTESIAN_POINT('Ctrl Pts',(1.59810042043673,-1.,0.946078063315257));
#24331=CARTESIAN_POINT('Ctrl Pts',(1.59810042043673,1.,0.946078063315257));
#24332=CARTESIAN_POINT('Ctrl Pts',(1.58744937487176,-1.,0.939646377893399));
#24333=CARTESIAN_POINT('Ctrl Pts',(1.58744937487176,1.,0.939646377893399));
#24334=CARTESIAN_POINT('Ctrl Pts',(1.57499388382243,-1.,0.932246680108685));
#24335=CARTESIAN_POINT('Ctrl Pts',(1.57499388382243,1.,0.932246680108685));
#24336=CARTESIAN_POINT('Ctrl Pts',(1.56065988578893,-1.,0.923832188944341));
#24337=CARTESIAN_POINT('Ctrl Pts',(1.56065988578893,1.,0.923832188944341));
#24338=CARTESIAN_POINT('Ctrl Pts',(1.54440491149498,-1.,0.914375919026456));
#24339=CARTESIAN_POINT('Ctrl Pts',(1.54440491149498,1.,0.914375919026456));
#24340=CARTESIAN_POINT('Ctrl Pts',(1.52984849887993,-1.,0.905967409625651));
#24341=CARTESIAN_POINT('Ctrl Pts',(1.52984849887993,1.,0.905967409625651));
#24342=CARTESIAN_POINT('Ctrl Pts',(1.51805569590094,-1.,0.899185047483511));
#24343=CARTESIAN_POINT('Ctrl Pts',(1.51805569590094,1.,0.899185047483511));
#24344=CARTESIAN_POINT('Ctrl Pts',(1.50980486806688,-1.,0.894452006964544));
#24345=CARTESIAN_POINT('Ctrl Pts',(1.50980486806688,1.,0.894452006964544));
#24346=CARTESIAN_POINT('Ctrl Pts',(1.5055822144029,-1.,0.892032620296856));
#24347=CARTESIAN_POINT('Ctrl Pts',(1.5055822144029,1.,0.892032620296856));
#24348=CARTESIAN_POINT('',(1.81978687191668,1.,1.23627494547115));
#24349=CARTESIAN_POINT('Ctrl Pts',(1.81978687191668,1.,1.23627494547115));
#24350=CARTESIAN_POINT('Ctrl Pts',(1.81925017193666,1.,1.23509651170476));
#24351=CARTESIAN_POINT('Ctrl Pts',(1.81817389921279,1.,1.2327422452705));
#24352=CARTESIAN_POINT('Ctrl Pts',(1.8165508718364,1.,1.2292186489137));
#24353=CARTESIAN_POINT('Ctrl Pts',(1.81436959210434,1.,1.2245361330495));
#24354=CARTESIAN_POINT('Ctrl Pts',(1.81161420806656,1.,1.21870906103557));
#24355=CARTESIAN_POINT('Ctrl Pts',(1.80882996917129,1.,1.21290815708314));
#24356=CARTESIAN_POINT('Ctrl Pts',(1.80601678480707,1.,1.20713356605475));
#24357=CARTESIAN_POINT('Ctrl Pts',(1.80317454838603,1.,1.20138548938974));
#24358=CARTESIAN_POINT('Ctrl Pts',(1.80030314369879,1.,1.19566418930242));
#24359=CARTESIAN_POINT('Ctrl Pts',(1.79740245923478,1.,1.18996997934445));
#24360=CARTESIAN_POINT('Ctrl Pts',(1.79447240321515,1.,1.18430321697432));
#24361=CARTESIAN_POINT('Ctrl Pts',(1.79151291552689,1.,1.17866429440809));
#24362=CARTESIAN_POINT('Ctrl Pts',(1.78852398877616,1.,1.17305363177328));
#24363=CARTESIAN_POINT('Ctrl Pts',(1.78550566040443,1.,1.16747166312303));
#24364=CARTESIAN_POINT('Ctrl Pts',(1.78245795881009,1.,1.16191881298499));
#24365=CARTESIAN_POINT('Ctrl Pts',(1.77938085564275,1.,1.15639547194698));
#24366=CARTESIAN_POINT('Ctrl Pts',(1.7762742255701,1.,1.15090197841515));
#24367=CARTESIAN_POINT('Ctrl Pts',(1.77313777896194,1.,1.1454385822692));
#24368=CARTESIAN_POINT('Ctrl Pts',(1.76997111386769,1.,1.14000548336975));
#24369=CARTESIAN_POINT('Ctrl Pts',(1.76677384551862,1.,1.1346029180462));
#24370=CARTESIAN_POINT('Ctrl Pts',(1.7635457196617,1.,1.12923123555075));
#24371=CARTESIAN_POINT('Ctrl Pts',(1.76028671825096,1.,1.12389096855086));
#24372=CARTESIAN_POINT('Ctrl Pts',(1.75699720772105,1.,1.11858293216763));
#24373=CARTESIAN_POINT('Ctrl Pts',(1.7536777209463,1.,1.11330807582551));
#24374=CARTESIAN_POINT('Ctrl Pts',(1.7503286607592,1.,1.10806728183007));
#24375=CARTESIAN_POINT('Ctrl Pts',(1.74695004214923,1.,1.10286118991143));
#24376=CARTESIAN_POINT('Ctrl Pts',(1.74354119236208,1.,1.09768999241226));
#24377=CARTESIAN_POINT('Ctrl Pts',(1.74010053962247,1.,1.09255329056493));
#24378=CARTESIAN_POINT('Ctrl Pts',(1.73662628326091,1.,1.08745056285427));
#24379=CARTESIAN_POINT('Ctrl Pts',(1.73311705663407,1.,1.08238162784749));
#24380=CARTESIAN_POINT('Ctrl Pts',(1.72957248977424,1.,1.0773470373727));
#24381=CARTESIAN_POINT('Ctrl Pts',(1.72599406198488,1.,1.07234866990252));
#24382=CARTESIAN_POINT('Ctrl Pts',(1.72238500928453,1.,1.06738966975462));
#24383=CARTESIAN_POINT('Ctrl Pts',(1.71874858456904,1.,1.06247324680647));
#24384=CARTESIAN_POINT('Ctrl Pts',(1.7150865442702,1.,1.05760163192479));
#24385=CARTESIAN_POINT('Ctrl Pts',(1.71139783543989,1.,1.05277517202855));
#24386=CARTESIAN_POINT('Ctrl Pts',(1.70767646263649,1.,1.04799085404995));
#24387=CARTESIAN_POINT('Ctrl Pts',(1.70391338707982,1.,1.04324363334554));
#24388=CARTESIAN_POINT('Ctrl Pts',(1.70010052930962,1.,1.03852922490789));
#24389=CARTESIAN_POINT('Ctrl Pts',(1.69623414782771,1.,1.03384646003588));
#24390=CARTESIAN_POINT('Ctrl Pts',(1.69231840863458,1.,1.02919977579147));
#24391=CARTESIAN_POINT('Ctrl Pts',(1.68836910178447,1.,1.02460180535255));
#24392=CARTESIAN_POINT('Ctrl Pts',(1.68440578021706,1.,1.02006795074201));
#24393=CARTESIAN_POINT('Ctrl Pts',(1.68044289894798,1.,1.01561026162773));
#24394=CARTESIAN_POINT('Ctrl Pts',(1.67648246776464,1.,1.01123236493511));
#24395=CARTESIAN_POINT('Ctrl Pts',(1.67250335383293,1.,1.00692206696414));
#24396=CARTESIAN_POINT('Ctrl Pts',(1.66846059277303,1.,1.00265091003727));
#24397=CARTESIAN_POINT('Ctrl Pts',(1.66430758030376,1.,0.998389654952758));
#24398=CARTESIAN_POINT('Ctrl Pts',(1.66001553809947,1.,0.994121836661306));
#24399=CARTESIAN_POINT('Ctrl Pts',(1.65559044289699,1.,0.989855627854165));
#24400=CARTESIAN_POINT('Ctrl Pts',(1.65110016612638,1.,0.985642622920821));
#24401=CARTESIAN_POINT('Ctrl Pts',(1.64665139190656,1.,0.981562530939489));
#24402=CARTESIAN_POINT('Ctrl Pts',(1.64233990826687,1.,0.977689794119417));
#24403=CARTESIAN_POINT('Ctrl Pts',(1.63820952658144,1.,0.974066058287419));
#24404=CARTESIAN_POINT('Ctrl Pts',(1.63420665729798,1.,0.970669715997509));
#24405=CARTESIAN_POINT('Ctrl Pts',(1.63013849959461,1.,0.967387853230345));
#24406=CARTESIAN_POINT('Ctrl Pts',(1.62571930670187,1.,0.964046107040536));
#24407=CARTESIAN_POINT('Ctrl Pts',(1.62061638140221,1.,0.960438326101729));
#24408=CARTESIAN_POINT('Ctrl Pts',(1.61449324337085,1.,0.956354422920671));
#24409=CARTESIAN_POINT('Ctrl Pts',(1.60706069896936,1.,0.951613284356035));
#24410=CARTESIAN_POINT('Ctrl Pts',(1.59810042043673,1.,0.946078063315257));
#24411=CARTESIAN_POINT('Ctrl Pts',(1.58744937487176,1.,0.939646377893399));
#24412=CARTESIAN_POINT('Ctrl Pts',(1.57499388382243,1.,0.932246680108685));
#24413=CARTESIAN_POINT('Ctrl Pts',(1.56065988578893,1.,0.923832188944341));
#24414=CARTESIAN_POINT('Ctrl Pts',(1.54440491149498,1.,0.914375919026456));
#24415=CARTESIAN_POINT('Ctrl Pts',(1.52984849887993,1.,0.905967409625651));
#24416=CARTESIAN_POINT('Ctrl Pts',(1.51805569590094,1.,0.899185047483511));
#24417=CARTESIAN_POINT('Ctrl Pts',(1.50980486806688,1.,0.894452006964544));
#24418=CARTESIAN_POINT('Ctrl Pts',(1.5055822144029,1.,0.892032620296856));
#24419=CARTESIAN_POINT('',(1.81978687191668,0.,1.23627494547115));
#24420=CARTESIAN_POINT('Origin',(1.73811241238545,0.,1.34869019493419));
#24421=CARTESIAN_POINT('',(1.73811241238545,1.,1.34869019493419));
#24422=CARTESIAN_POINT('',(1.81978687191668,1.,1.23627494547115));
#24423=CARTESIAN_POINT('',(1.73811241238545,0.,1.34869019493419));
#24424=CARTESIAN_POINT('Ctrl Pts',(1.31362392696032,-1.,1.15624053661742));
#24425=CARTESIAN_POINT('Ctrl Pts',(1.31362392696032,1.,1.15624053661742));
#24426=CARTESIAN_POINT('Ctrl Pts',(1.31722977216397,-1.,1.15950888730809));
#24427=CARTESIAN_POINT('Ctrl Pts',(1.31722977216397,1.,1.15950888730809));
#24428=CARTESIAN_POINT('Ctrl Pts',(1.32428080721772,-1.,1.16589330093588));
#24429=CARTESIAN_POINT('Ctrl Pts',(1.32428080721772,1.,1.16589330093588));
#24430=CARTESIAN_POINT('Ctrl Pts',(1.33437539347008,-1.,1.17501305789857));
#24431=CARTESIAN_POINT('Ctrl Pts',(1.33437539347008,1.,1.17501305789857));
#24432=CARTESIAN_POINT('Ctrl Pts',(1.34687054001093,-1.,1.18625865667441));
#24433=CARTESIAN_POINT('Ctrl Pts',(1.34687054001093,1.,1.18625865667441));
#24434=CARTESIAN_POINT('Ctrl Pts',(1.36088705043885,-1.,1.1987959077932));
#24435=CARTESIAN_POINT('Ctrl Pts',(1.36088705043885,1.,1.1987959077932));
#24436=CARTESIAN_POINT('Ctrl Pts',(1.37331915607905,-1.,1.20982812925645));
#24437=CARTESIAN_POINT('Ctrl Pts',(1.37331915607905,1.,1.20982812925645));
#24438=CARTESIAN_POINT('Ctrl Pts',(1.38420564527715,-1.,1.21938737280852));
#24439=CARTESIAN_POINT('Ctrl Pts',(1.38420564527715,1.,1.21938737280852));
#24440=CARTESIAN_POINT('Ctrl Pts',(1.39361389568796,-1.,1.22752961899387));
#24441=CARTESIAN_POINT('Ctrl Pts',(1.39361389568796,1.,1.22752961899387));
#24442=CARTESIAN_POINT('Ctrl Pts',(1.40164708206106,-1.,1.23434087290423));
#24443=CARTESIAN_POINT('Ctrl Pts',(1.40164708206106,1.,1.23434087290423));
#24444=CARTESIAN_POINT('Ctrl Pts',(1.40845295531283,-1.,1.23994455029534));
#24445=CARTESIAN_POINT('Ctrl Pts',(1.40845295531283,1.,1.23994455029534));
#24446=CARTESIAN_POINT('Ctrl Pts',(1.41422913175179,-1.,1.24450600513056));
#24447=CARTESIAN_POINT('Ctrl Pts',(1.41422913175179,1.,1.24450600513056));
#24448=CARTESIAN_POINT('Ctrl Pts',(1.41923722596025,-1.,1.24824430986571));
#24449=CARTESIAN_POINT('Ctrl Pts',(1.41923722596025,1.,1.24824430986571));
#24450=CARTESIAN_POINT('Ctrl Pts',(1.42378102115575,-1.,1.2514145557001));
#24451=CARTESIAN_POINT('Ctrl Pts',(1.42378102115575,1.,1.2514145557001));
#24452=CARTESIAN_POINT('Ctrl Pts',(1.42815938799387,-1.,1.25426945222639));
#24453=CARTESIAN_POINT('Ctrl Pts',(1.42815938799387,1.,1.25426945222639));
#24454=CARTESIAN_POINT('Ctrl Pts',(1.43262645609691,-1.,1.25702687965755));
#24455=CARTESIAN_POINT('Ctrl Pts',(1.43262645609691,1.,1.25702687965755));
#24456=CARTESIAN_POINT('Ctrl Pts',(1.43734919180847,-1.,1.25983531012005));
#24457=CARTESIAN_POINT('Ctrl Pts',(1.43734919180847,1.,1.25983531012005));
#24458=CARTESIAN_POINT('Ctrl Pts',(1.44236470511303,-1.,1.26273903323859));
#24459=CARTESIAN_POINT('Ctrl Pts',(1.44236470511303,1.,1.26273903323859));
#24460=CARTESIAN_POINT('Ctrl Pts',(1.44761985001662,-1.,1.26570925118868));
#24461=CARTESIAN_POINT('Ctrl Pts',(1.44761985001662,1.,1.26570925118868));
#24462=CARTESIAN_POINT('Ctrl Pts',(1.45301422764247,-1.,1.2686778680489));
#24463=CARTESIAN_POINT('Ctrl Pts',(1.45301422764247,1.,1.2686778680489));
#24464=CARTESIAN_POINT('Ctrl Pts',(1.45843906294697,-1.,1.27156805265289));
#24465=CARTESIAN_POINT('Ctrl Pts',(1.45843906294697,1.,1.27156805265289));
#24466=CARTESIAN_POINT('Ctrl Pts',(1.46382431332476,-1.,1.27433119897822));
#24467=CARTESIAN_POINT('Ctrl Pts',(1.46382431332476,1.,1.27433119897822));
#24468=CARTESIAN_POINT('Ctrl Pts',(1.46916035917133,-1.,1.2769641483109));
#24469=CARTESIAN_POINT('Ctrl Pts',(1.46916035917133,1.,1.2769641483109));
#24470=CARTESIAN_POINT('Ctrl Pts',(1.4744717526707,-1.,1.2794891824849));
#24471=CARTESIAN_POINT('Ctrl Pts',(1.4744717526707,1.,1.2794891824849));
#24472=CARTESIAN_POINT('Ctrl Pts',(1.47980070347095,-1.,1.28194158939517));
#24473=CARTESIAN_POINT('Ctrl Pts',(1.47980070347095,1.,1.28194158939517));
#24474=CARTESIAN_POINT('Ctrl Pts',(1.4851881711891,-1.,1.28435533880201));
#24475=CARTESIAN_POINT('Ctrl Pts',(1.4851881711891,1.,1.28435533880201));
#24476=CARTESIAN_POINT('Ctrl Pts',(1.4906522831278,-1.,1.2867467611644));
#24477=CARTESIAN_POINT('Ctrl Pts',(1.4906522831278,1.,1.2867467611644));
#24478=CARTESIAN_POINT('Ctrl Pts',(1.49618896881754,-1.,1.28911506584254));
#24479=CARTESIAN_POINT('Ctrl Pts',(1.49618896881754,1.,1.28911506584254));
#24480=CARTESIAN_POINT('Ctrl Pts',(1.50178230149776,-1.,1.29145022885181));
#24481=CARTESIAN_POINT('Ctrl Pts',(1.50178230149776,1.,1.29145022885181));
#24482=CARTESIAN_POINT('Ctrl Pts',(1.50741159078365,-1.,1.29373841372842));
#24483=CARTESIAN_POINT('Ctrl Pts',(1.50741159078365,1.,1.29373841372842));
#24484=CARTESIAN_POINT('Ctrl Pts',(1.51305994241402,-1.,1.29596850710509));
#24485=CARTESIAN_POINT('Ctrl Pts',(1.51305994241402,1.,1.29596850710509));
#24486=CARTESIAN_POINT('Ctrl Pts',(1.51872184912724,-1.,1.29813791800747));
#24487=CARTESIAN_POINT('Ctrl Pts',(1.51872184912724,1.,1.29813791800747));
#24488=CARTESIAN_POINT('Ctrl Pts',(1.52439957861062,-1.,1.30024984366328));
#24489=CARTESIAN_POINT('Ctrl Pts',(1.52439957861062,1.,1.30024984366328));
#24490=CARTESIAN_POINT('Ctrl Pts',(1.53009970283891,-1.,1.30231064395568));
#24491=CARTESIAN_POINT('Ctrl Pts',(1.53009970283891,1.,1.30231064395568));
#24492=CARTESIAN_POINT('Ctrl Pts',(1.53582981268977,-1.,1.30432735639489));
#24493=CARTESIAN_POINT('Ctrl Pts',(1.53582981268977,1.,1.30432735639489));
#24494=CARTESIAN_POINT('Ctrl Pts',(1.54159462645432,-1.,1.30630475189556));
#24495=CARTESIAN_POINT('Ctrl Pts',(1.54159462645432,1.,1.30630475189556));
#24496=CARTESIAN_POINT('Ctrl Pts',(1.54739413957185,-1.,1.30824393907473));
#24497=CARTESIAN_POINT('Ctrl Pts',(1.54739413957185,1.,1.30824393907473));
#24498=CARTESIAN_POINT('Ctrl Pts',(1.55322568759481,-1.,1.31014393684222));
#24499=CARTESIAN_POINT('Ctrl Pts',(1.55322568759481,1.,1.31014393684222));
#24500=CARTESIAN_POINT('Ctrl Pts',(1.55908521254821,-1.,1.31200264341696));
#24501=CARTESIAN_POINT('Ctrl Pts',(1.55908521254821,1.,1.31200264341696));
#24502=CARTESIAN_POINT('Ctrl Pts',(1.56496872402353,-1.,1.31381795281002));
#24503=CARTESIAN_POINT('Ctrl Pts',(1.56496872402353,1.,1.31381795281002));
#24504=CARTESIAN_POINT('Ctrl Pts',(1.57087397835723,-1.,1.31558903860016));
#24505=CARTESIAN_POINT('Ctrl Pts',(1.57087397835723,1.,1.31558903860016));
#24506=CARTESIAN_POINT('Ctrl Pts',(1.5768005650559,-1.,1.31731642317187));
#24507=CARTESIAN_POINT('Ctrl Pts',(1.5768005650559,1.,1.31731642317187));
#24508=CARTESIAN_POINT('Ctrl Pts',(1.58274907898834,-1.,1.31900135021432));
#24509=CARTESIAN_POINT('Ctrl Pts',(1.58274907898834,1.,1.31900135021432));
#24510=CARTESIAN_POINT('Ctrl Pts',(1.58872057258245,-1.,1.32064537110892));
#24511=CARTESIAN_POINT('Ctrl Pts',(1.58872057258245,1.,1.32064537110892));
#24512=CARTESIAN_POINT('Ctrl Pts',(1.59471591079403,-1.,1.32224985747682));
#24513=CARTESIAN_POINT('Ctrl Pts',(1.59471591079403,1.,1.32224985747682));
#24514=CARTESIAN_POINT('Ctrl Pts',(1.60073511858687,-1.,1.32381550858256));
#24515=CARTESIAN_POINT('Ctrl Pts',(1.60073511858687,1.,1.32381550858256));
#24516=CARTESIAN_POINT('Ctrl Pts',(1.60677758290954,-1.,1.32534250785782));
#24517=CARTESIAN_POINT('Ctrl Pts',(1.60677758290954,1.,1.32534250785782));
#24518=CARTESIAN_POINT('Ctrl Pts',(1.6128423401575,-1.,1.32683074483356));
#24519=CARTESIAN_POINT('Ctrl Pts',(1.6128423401575,1.,1.32683074483356));
#24520=CARTESIAN_POINT('Ctrl Pts',(1.61892832270724,-1.,1.32828000610449));
#24521=CARTESIAN_POINT('Ctrl Pts',(1.61892832270724,1.,1.32828000610449));
#24522=CARTESIAN_POINT('Ctrl Pts',(1.62503464209797,-1.,1.3296901950568));
#24523=CARTESIAN_POINT('Ctrl Pts',(1.62503464209797,1.,1.3296901950568));
#24524=CARTESIAN_POINT('Ctrl Pts',(1.63116079730923,-1.,1.33106149345645));
#24525=CARTESIAN_POINT('Ctrl Pts',(1.63116079730923,1.,1.33106149345645));
#24526=CARTESIAN_POINT('Ctrl Pts',(1.63730653475089,-1.,1.33239425103724));
#24527=CARTESIAN_POINT('Ctrl Pts',(1.63730653475089,1.,1.33239425103724));
#24528=CARTESIAN_POINT('Ctrl Pts',(1.6434717485603,-1.,1.33368890676572));
#24529=CARTESIAN_POINT('Ctrl Pts',(1.6434717485603,1.,1.33368890676572));
#24530=CARTESIAN_POINT('Ctrl Pts',(1.6496563728683,-1.,1.33494590467993));
#24531=CARTESIAN_POINT('Ctrl Pts',(1.6496563728683,1.,1.33494590467993));
#24532=CARTESIAN_POINT('Ctrl Pts',(1.65586025952593,-1.,1.33616559745172));
#24533=CARTESIAN_POINT('Ctrl Pts',(1.65586025952593,1.,1.33616559745172));
#24534=CARTESIAN_POINT('Ctrl Pts',(1.66208312541983,-1.,1.33734820885262));
#24535=CARTESIAN_POINT('Ctrl Pts',(1.66208312541983,1.,1.33734820885262));
#24536=CARTESIAN_POINT('Ctrl Pts',(1.66832460783989,-1.,1.33849388654388));
#24537=CARTESIAN_POINT('Ctrl Pts',(1.66832460783989,1.,1.33849388654388));
#24538=CARTESIAN_POINT('Ctrl Pts',(1.67458429426086,-1.,1.3396027347034));
#24539=CARTESIAN_POINT('Ctrl Pts',(1.67458429426086,1.,1.3396027347034));
#24540=CARTESIAN_POINT('Ctrl Pts',(1.68086176030362,-1.,1.34067485185203));
#24541=CARTESIAN_POINT('Ctrl Pts',(1.68086176030362,1.,1.34067485185203));
#24542=CARTESIAN_POINT('Ctrl Pts',(1.68715660868764,-1.,1.341710374848));
#24543=CARTESIAN_POINT('Ctrl Pts',(1.68715660868764,1.,1.341710374848));
#24544=CARTESIAN_POINT('Ctrl Pts',(1.6934684849687,-1.,1.34270948206319));
#24545=CARTESIAN_POINT('Ctrl Pts',(1.6934684849687,1.,1.34270948206319));
#24546=CARTESIAN_POINT('Ctrl Pts',(1.69979707754427,-1.,1.34367237124483));
#24547=CARTESIAN_POINT('Ctrl Pts',(1.69979707754427,1.,1.34367237124483));
#24548=CARTESIAN_POINT('Ctrl Pts',(1.70614212266738,-1.,1.34459924533831));
#24549=CARTESIAN_POINT('Ctrl Pts',(1.70614212266738,1.,1.34459924533831));
#24550=CARTESIAN_POINT('Ctrl Pts',(1.71250340686822,-1.,1.34549029589416));
#24551=CARTESIAN_POINT('Ctrl Pts',(1.71250340686822,1.,1.34549029589416));
#24552=CARTESIAN_POINT('Ctrl Pts',(1.7188807715049,-1.,1.34634568653227));
#24553=CARTESIAN_POINT('Ctrl Pts',(1.7188807715049,1.,1.34634568653227));
#24554=CARTESIAN_POINT('Ctrl Pts',(1.72527410680674,-1.,1.34716554819527));
#24555=CARTESIAN_POINT('Ctrl Pts',(1.72527410680674,1.,1.34716554819527));
#24556=CARTESIAN_POINT('Ctrl Pts',(1.7304014965394,-1.,1.34779309152035));
#24557=CARTESIAN_POINT('Ctrl Pts',(1.7304014965394,1.,1.34779309152035));
#24558=CARTESIAN_POINT('Ctrl Pts',(1.73425417885907,-1.,1.34824783112887));
#24559=CARTESIAN_POINT('Ctrl Pts',(1.73425417885907,1.,1.34824783112887));
#24560=CARTESIAN_POINT('Ctrl Pts',(1.73682580585691,-1.,1.34854391898045));
#24561=CARTESIAN_POINT('Ctrl Pts',(1.73682580585691,1.,1.34854391898045));
#24562=CARTESIAN_POINT('Ctrl Pts',(1.73811241238545,-1.,1.34869019493419));
#24563=CARTESIAN_POINT('Ctrl Pts',(1.73811241238545,1.,1.34869019493419));
#24564=CARTESIAN_POINT('',(1.31362392696032,1.,1.15624053661742));
#24565=CARTESIAN_POINT('Ctrl Pts',(1.31362392696032,1.,1.15624053661742));
#24566=CARTESIAN_POINT('Ctrl Pts',(1.31722977216397,1.,1.15950888730809));
#24567=CARTESIAN_POINT('Ctrl Pts',(1.32428080721772,1.,1.16589330093588));
#24568=CARTESIAN_POINT('Ctrl Pts',(1.33437539347008,1.,1.17501305789857));
#24569=CARTESIAN_POINT('Ctrl Pts',(1.34687054001093,1.,1.18625865667441));
#24570=CARTESIAN_POINT('Ctrl Pts',(1.36088705043885,1.,1.1987959077932));
#24571=CARTESIAN_POINT('Ctrl Pts',(1.37331915607905,1.,1.20982812925645));
#24572=CARTESIAN_POINT('Ctrl Pts',(1.38420564527715,1.,1.21938737280852));
#24573=CARTESIAN_POINT('Ctrl Pts',(1.39361389568796,1.,1.22752961899387));
#24574=CARTESIAN_POINT('Ctrl Pts',(1.40164708206106,1.,1.23434087290423));
#24575=CARTESIAN_POINT('Ctrl Pts',(1.40845295531283,1.,1.23994455029534));
#24576=CARTESIAN_POINT('Ctrl Pts',(1.41422913175179,1.,1.24450600513056));
#24577=CARTESIAN_POINT('Ctrl Pts',(1.41923722596025,1.,1.24824430986571));
#24578=CARTESIAN_POINT('Ctrl Pts',(1.42378102115575,1.,1.2514145557001));
#24579=CARTESIAN_POINT('Ctrl Pts',(1.42815938799387,1.,1.25426945222639));
#24580=CARTESIAN_POINT('Ctrl Pts',(1.43262645609691,1.,1.25702687965755));
#24581=CARTESIAN_POINT('Ctrl Pts',(1.43734919180847,1.,1.25983531012005));
#24582=CARTESIAN_POINT('Ctrl Pts',(1.44236470511303,1.,1.26273903323859));
#24583=CARTESIAN_POINT('Ctrl Pts',(1.44761985001662,1.,1.26570925118868));
#24584=CARTESIAN_POINT('Ctrl Pts',(1.45301422764247,1.,1.2686778680489));
#24585=CARTESIAN_POINT('Ctrl Pts',(1.45843906294697,1.,1.27156805265289));
#24586=CARTESIAN_POINT('Ctrl Pts',(1.46382431332476,1.,1.27433119897822));
#24587=CARTESIAN_POINT('Ctrl Pts',(1.46916035917133,1.,1.2769641483109));
#24588=CARTESIAN_POINT('Ctrl Pts',(1.4744717526707,1.,1.2794891824849));
#24589=CARTESIAN_POINT('Ctrl Pts',(1.47980070347095,1.,1.28194158939517));
#24590=CARTESIAN_POINT('Ctrl Pts',(1.4851881711891,1.,1.28435533880201));
#24591=CARTESIAN_POINT('Ctrl Pts',(1.4906522831278,1.,1.2867467611644));
#24592=CARTESIAN_POINT('Ctrl Pts',(1.49618896881754,1.,1.28911506584254));
#24593=CARTESIAN_POINT('Ctrl Pts',(1.50178230149776,1.,1.29145022885181));
#24594=CARTESIAN_POINT('Ctrl Pts',(1.50741159078365,1.,1.29373841372842));
#24595=CARTESIAN_POINT('Ctrl Pts',(1.51305994241402,1.,1.29596850710509));
#24596=CARTESIAN_POINT('Ctrl Pts',(1.51872184912724,1.,1.29813791800747));
#24597=CARTESIAN_POINT('Ctrl Pts',(1.52439957861062,1.,1.30024984366328));
#24598=CARTESIAN_POINT('Ctrl Pts',(1.53009970283891,1.,1.30231064395568));
#24599=CARTESIAN_POINT('Ctrl Pts',(1.53582981268977,1.,1.30432735639489));
#24600=CARTESIAN_POINT('Ctrl Pts',(1.54159462645432,1.,1.30630475189556));
#24601=CARTESIAN_POINT('Ctrl Pts',(1.54739413957185,1.,1.30824393907473));
#24602=CARTESIAN_POINT('Ctrl Pts',(1.55322568759481,1.,1.31014393684222));
#24603=CARTESIAN_POINT('Ctrl Pts',(1.55908521254821,1.,1.31200264341696));
#24604=CARTESIAN_POINT('Ctrl Pts',(1.56496872402353,1.,1.31381795281002));
#24605=CARTESIAN_POINT('Ctrl Pts',(1.57087397835723,1.,1.31558903860016));
#24606=CARTESIAN_POINT('Ctrl Pts',(1.5768005650559,1.,1.31731642317187));
#24607=CARTESIAN_POINT('Ctrl Pts',(1.58274907898834,1.,1.31900135021432));
#24608=CARTESIAN_POINT('Ctrl Pts',(1.58872057258245,1.,1.32064537110892));
#24609=CARTESIAN_POINT('Ctrl Pts',(1.59471591079403,1.,1.32224985747682));
#24610=CARTESIAN_POINT('Ctrl Pts',(1.60073511858687,1.,1.32381550858256));
#24611=CARTESIAN_POINT('Ctrl Pts',(1.60677758290954,1.,1.32534250785782));
#24612=CARTESIAN_POINT('Ctrl Pts',(1.6128423401575,1.,1.32683074483356));
#24613=CARTESIAN_POINT('Ctrl Pts',(1.61892832270724,1.,1.32828000610449));
#24614=CARTESIAN_POINT('Ctrl Pts',(1.62503464209797,1.,1.3296901950568));
#24615=CARTESIAN_POINT('Ctrl Pts',(1.63116079730923,1.,1.33106149345645));
#24616=CARTESIAN_POINT('Ctrl Pts',(1.63730653475089,1.,1.33239425103724));
#24617=CARTESIAN_POINT('Ctrl Pts',(1.6434717485603,1.,1.33368890676572));
#24618=CARTESIAN_POINT('Ctrl Pts',(1.6496563728683,1.,1.33494590467993));
#24619=CARTESIAN_POINT('Ctrl Pts',(1.65586025952593,1.,1.33616559745172));
#24620=CARTESIAN_POINT('Ctrl Pts',(1.66208312541983,1.,1.33734820885262));
#24621=CARTESIAN_POINT('Ctrl Pts',(1.66832460783989,1.,1.33849388654388));
#24622=CARTESIAN_POINT('Ctrl Pts',(1.67458429426086,1.,1.3396027347034));
#24623=CARTESIAN_POINT('Ctrl Pts',(1.68086176030362,1.,1.34067485185203));
#24624=CARTESIAN_POINT('Ctrl Pts',(1.68715660868764,1.,1.341710374848));
#24625=CARTESIAN_POINT('Ctrl Pts',(1.6934684849687,1.,1.34270948206319));
#24626=CARTESIAN_POINT('Ctrl Pts',(1.69979707754427,1.,1.34367237124483));
#24627=CARTESIAN_POINT('Ctrl Pts',(1.70614212266738,1.,1.34459924533831));
#24628=CARTESIAN_POINT('Ctrl Pts',(1.71250340686822,1.,1.34549029589416));
#24629=CARTESIAN_POINT('Ctrl Pts',(1.7188807715049,1.,1.34634568653227));
#24630=CARTESIAN_POINT('Ctrl Pts',(1.72527410680674,1.,1.34716554819527));
#24631=CARTESIAN_POINT('Ctrl Pts',(1.7304014965394,1.,1.34779309152035));
#24632=CARTESIAN_POINT('Ctrl Pts',(1.73425417885907,1.,1.34824783112887));
#24633=CARTESIAN_POINT('Ctrl Pts',(1.73682580585691,1.,1.34854391898045));
#24634=CARTESIAN_POINT('Ctrl Pts',(1.73811241238545,1.,1.34869019493419));
#24635=CARTESIAN_POINT('',(1.31362392696032,0.,1.15624053661742));
#24636=CARTESIAN_POINT('Origin',(0.,0.,0.));
#24637=CARTESIAN_POINT('',(1.15624053661742,1.,1.31362392696033));
#24638=CARTESIAN_POINT('Origin',(0.,1.,0.));
#24639=CARTESIAN_POINT('',(1.15624053661742,0.,1.31362392696032));
#24640=CARTESIAN_POINT('Ctrl Pts',(1.34869019493419,-1.,1.73811241238545));
#24641=CARTESIAN_POINT('Ctrl Pts',(1.34869019493419,1.,1.73811241238545));
#24642=CARTESIAN_POINT('Ctrl Pts',(1.34854391898145,-1.,1.73682580585819));
#24643=CARTESIAN_POINT('Ctrl Pts',(1.34854391898145,1.,1.73682580585819));
#24644=CARTESIAN_POINT('Ctrl Pts',(1.34824783113158,-1.,1.73425417886255));
#24645=CARTESIAN_POINT('Ctrl Pts',(1.34824783113158,1.,1.73425417886255));
#24646=CARTESIAN_POINT('Ctrl Pts',(1.3477930915247,-1.,1.73040149654497));
#24647=CARTESIAN_POINT('Ctrl Pts',(1.3477930915247,1.,1.73040149654497));
#24648=CARTESIAN_POINT('Ctrl Pts',(1.34716554820013,-1.,1.72527410681298));
#24649=CARTESIAN_POINT('Ctrl Pts',(1.34716554820013,1.,1.72527410681298));
#24650=CARTESIAN_POINT('Ctrl Pts',(1.34634568653586,-1.,1.7188807715095));
#24651=CARTESIAN_POINT('Ctrl Pts',(1.34634568653586,1.,1.7188807715095));
#24652=CARTESIAN_POINT('Ctrl Pts',(1.34549029589563,-1.,1.71250340687011));
#24653=CARTESIAN_POINT('Ctrl Pts',(1.34549029589563,1.,1.71250340687011));
#24654=CARTESIAN_POINT('Ctrl Pts',(1.34459924533783,-1.,1.70614212266676));
#24655=CARTESIAN_POINT('Ctrl Pts',(1.34459924533783,1.,1.70614212266676));
#24656=CARTESIAN_POINT('Ctrl Pts',(1.34367237124322,-1.,1.69979707754221));
#24657=CARTESIAN_POINT('Ctrl Pts',(1.34367237124322,1.,1.69979707754221));
#24658=CARTESIAN_POINT('Ctrl Pts',(1.34270948206139,-1.,1.6934684849664));
#24659=CARTESIAN_POINT('Ctrl Pts',(1.34270948206139,1.,1.6934684849664));
#24660=CARTESIAN_POINT('Ctrl Pts',(1.34171037484673,-1.,1.68715660868602));
#24661=CARTESIAN_POINT('Ctrl Pts',(1.34171037484673,1.,1.68715660868602));
#24662=CARTESIAN_POINT('Ctrl Pts',(1.3406748518516,-1.,1.68086176030308));
#24663=CARTESIAN_POINT('Ctrl Pts',(1.3406748518516,1.,1.68086176030308));
#24664=CARTESIAN_POINT('Ctrl Pts',(1.33960273470372,-1.,1.67458429426126));
#24665=CARTESIAN_POINT('Ctrl Pts',(1.33960273470372,1.,1.67458429426126));
#24666=CARTESIAN_POINT('Ctrl Pts',(1.33849388654458,-1.,1.66832460784078));
#24667=CARTESIAN_POINT('Ctrl Pts',(1.33849388654458,1.,1.66832460784078));
#24668=CARTESIAN_POINT('Ctrl Pts',(1.33734820885331,-1.,1.66208312542073));
#24669=CARTESIAN_POINT('Ctrl Pts',(1.33734820885331,1.,1.66208312542073));
#24670=CARTESIAN_POINT('Ctrl Pts',(1.33616559745217,-1.,1.65586025952651));
#24671=CARTESIAN_POINT('Ctrl Pts',(1.33616559745217,1.,1.65586025952651));
#24672=CARTESIAN_POINT('Ctrl Pts',(1.33494590468003,-1.,1.64965637286843));
#24673=CARTESIAN_POINT('Ctrl Pts',(1.33494590468003,1.,1.64965637286843));
#24674=CARTESIAN_POINT('Ctrl Pts',(1.33368890676554,-1.,1.64347174856007));
#24675=CARTESIAN_POINT('Ctrl Pts',(1.33368890676554,1.,1.64347174856007));
#24676=CARTESIAN_POINT('Ctrl Pts',(1.33239425103694,-1.,1.6373065347505));
#24677=CARTESIAN_POINT('Ctrl Pts',(1.33239425103694,1.,1.6373065347505));
#24678=CARTESIAN_POINT('Ctrl Pts',(1.33106149345618,-1.,1.63116079730887));
#24679=CARTESIAN_POINT('Ctrl Pts',(1.33106149345618,1.,1.63116079730887));
#24680=CARTESIAN_POINT('Ctrl Pts',(1.32969019505665,-1.,1.62503464209777));
#24681=CARTESIAN_POINT('Ctrl Pts',(1.32969019505665,1.,1.62503464209777));
#24682=CARTESIAN_POINT('Ctrl Pts',(1.32828000610448,-1.,1.61892832270723));
#24683=CARTESIAN_POINT('Ctrl Pts',(1.32828000610448,1.,1.61892832270723));
#24684=CARTESIAN_POINT('Ctrl Pts',(1.32683074483365,-1.,1.61284234015762));
#24685=CARTESIAN_POINT('Ctrl Pts',(1.32683074483365,1.,1.61284234015762));
#24686=CARTESIAN_POINT('Ctrl Pts',(1.32534250785794,-1.,1.6067775829097));
#24687=CARTESIAN_POINT('Ctrl Pts',(1.32534250785794,1.,1.6067775829097));
#24688=CARTESIAN_POINT('Ctrl Pts',(1.32381550858266,-1.,1.600735118587));
#24689=CARTESIAN_POINT('Ctrl Pts',(1.32381550858266,1.,1.600735118587));
#24690=CARTESIAN_POINT('Ctrl Pts',(1.32224985747686,-1.,1.59471591079408));
#24691=CARTESIAN_POINT('Ctrl Pts',(1.32224985747686,1.,1.59471591079408));
#24692=CARTESIAN_POINT('Ctrl Pts',(1.32064537110891,-1.,1.58872057258244));
#24693=CARTESIAN_POINT('Ctrl Pts',(1.32064537110891,1.,1.58872057258244));
#24694=CARTESIAN_POINT('Ctrl Pts',(1.31900135021428,-1.,1.58274907898829));
#24695=CARTESIAN_POINT('Ctrl Pts',(1.31900135021428,1.,1.58274907898829));
#24696=CARTESIAN_POINT('Ctrl Pts',(1.31731642317183,-1.,1.57680056505585));
#24697=CARTESIAN_POINT('Ctrl Pts',(1.31731642317183,1.,1.57680056505585));
#24698=CARTESIAN_POINT('Ctrl Pts',(1.31558903860015,-1.,1.57087397835721));
#24699=CARTESIAN_POINT('Ctrl Pts',(1.31558903860015,1.,1.57087397835721));
#24700=CARTESIAN_POINT('Ctrl Pts',(1.31381795281002,-1.,1.56496872402352));
#24701=CARTESIAN_POINT('Ctrl Pts',(1.31381795281002,1.,1.56496872402352));
#24702=CARTESIAN_POINT('Ctrl Pts',(1.31200264341696,-1.,1.55908521254822));
#24703=CARTESIAN_POINT('Ctrl Pts',(1.31200264341696,1.,1.55908521254822));
#24704=CARTESIAN_POINT('Ctrl Pts',(1.31014393684221,-1.,1.55322568759481));
#24705=CARTESIAN_POINT('Ctrl Pts',(1.31014393684221,1.,1.55322568759481));
#24706=CARTESIAN_POINT('Ctrl Pts',(1.30824393907471,-1.,1.54739413957183));
#24707=CARTESIAN_POINT('Ctrl Pts',(1.30824393907471,1.,1.54739413957183));
#24708=CARTESIAN_POINT('Ctrl Pts',(1.30630475189553,-1.,1.54159462645428));
#24709=CARTESIAN_POINT('Ctrl Pts',(1.30630475189553,1.,1.54159462645428));
#24710=CARTESIAN_POINT('Ctrl Pts',(1.30432735639487,-1.,1.53582981268976));
#24711=CARTESIAN_POINT('Ctrl Pts',(1.30432735639487,1.,1.53582981268976));
#24712=CARTESIAN_POINT('Ctrl Pts',(1.3023106439557,-1.,1.53009970283893));
#24713=CARTESIAN_POINT('Ctrl Pts',(1.3023106439557,1.,1.53009970283893));
#24714=CARTESIAN_POINT('Ctrl Pts',(1.30024984366334,-1.,1.5243995786107));
#24715=CARTESIAN_POINT('Ctrl Pts',(1.30024984366334,1.,1.5243995786107));
#24716=CARTESIAN_POINT('Ctrl Pts',(1.29813791800757,-1.,1.51872184912735));
#24717=CARTESIAN_POINT('Ctrl Pts',(1.29813791800757,1.,1.51872184912735));
#24718=CARTESIAN_POINT('Ctrl Pts',(1.29596850710518,-1.,1.51305994241412));
#24719=CARTESIAN_POINT('Ctrl Pts',(1.29596850710518,1.,1.51305994241412));
#24720=CARTESIAN_POINT('Ctrl Pts',(1.29373841372843,-1.,1.50741159078367));
#24721=CARTESIAN_POINT('Ctrl Pts',(1.29373841372843,1.,1.50741159078367));
#24722=CARTESIAN_POINT('Ctrl Pts',(1.29145022885171,-1.,1.50178230149764));
#24723=CARTESIAN_POINT('Ctrl Pts',(1.29145022885171,1.,1.50178230149764));
#24724=CARTESIAN_POINT('Ctrl Pts',(1.28911506584232,-1.,1.49618896881729));
#24725=CARTESIAN_POINT('Ctrl Pts',(1.28911506584232,1.,1.49618896881729));
#24726=CARTESIAN_POINT('Ctrl Pts',(1.28674676116415,-1.,1.4906522831275));
#24727=CARTESIAN_POINT('Ctrl Pts',(1.28674676116415,1.,1.4906522831275));
#24728=CARTESIAN_POINT('Ctrl Pts',(1.28435533880184,-1.,1.48518817118891));
#24729=CARTESIAN_POINT('Ctrl Pts',(1.28435533880184,1.,1.48518817118891));
#24730=CARTESIAN_POINT('Ctrl Pts',(1.28194158939522,-1.,1.47980070347102));
#24731=CARTESIAN_POINT('Ctrl Pts',(1.28194158939522,1.,1.47980070347102));
#24732=CARTESIAN_POINT('Ctrl Pts',(1.27948918248524,-1.,1.4744717526711));
#24733=CARTESIAN_POINT('Ctrl Pts',(1.27948918248524,1.,1.4744717526711));
#24734=CARTESIAN_POINT('Ctrl Pts',(1.27696414831144,-1.,1.46916035917197));
#24735=CARTESIAN_POINT('Ctrl Pts',(1.27696414831144,1.,1.46916035917197));
#24736=CARTESIAN_POINT('Ctrl Pts',(1.27433119897877,-1.,1.4638243133254));
#24737=CARTESIAN_POINT('Ctrl Pts',(1.27433119897877,1.,1.4638243133254));
#24738=CARTESIAN_POINT('Ctrl Pts',(1.27156805265312,-1.,1.45843906294725));
#24739=CARTESIAN_POINT('Ctrl Pts',(1.27156805265312,1.,1.45843906294725));
#24740=CARTESIAN_POINT('Ctrl Pts',(1.26867786804854,-1.,1.45301422764205));
#24741=CARTESIAN_POINT('Ctrl Pts',(1.26867786804854,1.,1.45301422764205));
#24742=CARTESIAN_POINT('Ctrl Pts',(1.26570925118767,-1.,1.44761985001544));
#24743=CARTESIAN_POINT('Ctrl Pts',(1.26570925118767,1.,1.44761985001544));
#24744=CARTESIAN_POINT('Ctrl Pts',(1.26273903323723,-1.,1.44236470511145));
#24745=CARTESIAN_POINT('Ctrl Pts',(1.26273903323723,1.,1.44236470511145));
#24746=CARTESIAN_POINT('Ctrl Pts',(1.25983531011894,-1.,1.43734919180719));
#24747=CARTESIAN_POINT('Ctrl Pts',(1.25983531011894,1.,1.43734919180719));
#24748=CARTESIAN_POINT('Ctrl Pts',(1.25702687965744,-1.,1.43262645609679));
#24749=CARTESIAN_POINT('Ctrl Pts',(1.25702687965744,1.,1.43262645609679));
#24750=CARTESIAN_POINT('Ctrl Pts',(1.25426945222783,-1.,1.42815938799555));
#24751=CARTESIAN_POINT('Ctrl Pts',(1.25426945222783,1.,1.42815938799555));
#24752=CARTESIAN_POINT('Ctrl Pts',(1.25141455570299,-1.,1.42378102115911));
#24753=CARTESIAN_POINT('Ctrl Pts',(1.25141455570299,1.,1.42378102115911));
#24754=CARTESIAN_POINT('Ctrl Pts',(1.24824430986911,-1.,1.41923722596421));
#24755=CARTESIAN_POINT('Ctrl Pts',(1.24824430986911,1.,1.41923722596421));
#24756=CARTESIAN_POINT('Ctrl Pts',(1.24450600513278,-1.,1.41422913175437));
#24757=CARTESIAN_POINT('Ctrl Pts',(1.24450600513278,1.,1.41422913175437));
#24758=CARTESIAN_POINT('Ctrl Pts',(1.23994455029421,-1.,1.40845295531151));
#24759=CARTESIAN_POINT('Ctrl Pts',(1.23994455029421,1.,1.40845295531151));
#24760=CARTESIAN_POINT('Ctrl Pts',(1.23434087289768,-1.,1.40164708205345));
#24761=CARTESIAN_POINT('Ctrl Pts',(1.23434087289768,1.,1.40164708205345));
#24762=CARTESIAN_POINT('Ctrl Pts',(1.22752961898063,-1.,1.39361389567257));
#24763=CARTESIAN_POINT('Ctrl Pts',(1.22752961898063,1.,1.39361389567257));
#24764=CARTESIAN_POINT('Ctrl Pts',(1.21938737278853,-1.,1.38420564525391));
#24765=CARTESIAN_POINT('Ctrl Pts',(1.21938737278853,1.,1.38420564525391));
#24766=CARTESIAN_POINT('Ctrl Pts',(1.20982812923113,-1.,1.37331915604962));
#24767=CARTESIAN_POINT('Ctrl Pts',(1.20982812923113,1.,1.37331915604962));
#24768=CARTESIAN_POINT('Ctrl Pts',(1.1987959077656,-1.,1.36088705040677));
#24769=CARTESIAN_POINT('Ctrl Pts',(1.1987959077656,1.,1.36088705040677));
#24770=CARTESIAN_POINT('Ctrl Pts',(1.18625865664915,-1.,1.34687053998157));
#24771=CARTESIAN_POINT('Ctrl Pts',(1.18625865664915,1.,1.34687053998157));
#24772=CARTESIAN_POINT('Ctrl Pts',(1.17501305787994,-1.,1.33437539344842));
#24773=CARTESIAN_POINT('Ctrl Pts',(1.17501305787994,1.,1.33437539344842));
#24774=CARTESIAN_POINT('Ctrl Pts',(1.16589330092532,-1.,1.32428080720544));
#24775=CARTESIAN_POINT('Ctrl Pts',(1.16589330092532,1.,1.32428080720544));
#24776=CARTESIAN_POINT('Ctrl Pts',(1.15950888730433,-1.,1.3172297721596));
#24777=CARTESIAN_POINT('Ctrl Pts',(1.15950888730433,1.,1.3172297721596));
#24778=CARTESIAN_POINT('Ctrl Pts',(1.15624053661742,-1.,1.31362392696033));
#24779=CARTESIAN_POINT('Ctrl Pts',(1.15624053661742,1.,1.31362392696033));
#24780=CARTESIAN_POINT('',(1.34869019493419,1.,1.73811241238545));
#24781=CARTESIAN_POINT('Ctrl Pts',(1.34869019493419,1.,1.73811241238545));
#24782=CARTESIAN_POINT('Ctrl Pts',(1.34854391898145,1.,1.73682580585819));
#24783=CARTESIAN_POINT('Ctrl Pts',(1.34824783113158,1.,1.73425417886255));
#24784=CARTESIAN_POINT('Ctrl Pts',(1.3477930915247,1.,1.73040149654497));
#24785=CARTESIAN_POINT('Ctrl Pts',(1.34716554820013,1.,1.72527410681298));
#24786=CARTESIAN_POINT('Ctrl Pts',(1.34634568653586,1.,1.7188807715095));
#24787=CARTESIAN_POINT('Ctrl Pts',(1.34549029589563,1.,1.71250340687011));
#24788=CARTESIAN_POINT('Ctrl Pts',(1.34459924533783,1.,1.70614212266676));
#24789=CARTESIAN_POINT('Ctrl Pts',(1.34367237124322,1.,1.69979707754221));
#24790=CARTESIAN_POINT('Ctrl Pts',(1.34270948206139,1.,1.6934684849664));
#24791=CARTESIAN_POINT('Ctrl Pts',(1.34171037484673,1.,1.68715660868602));
#24792=CARTESIAN_POINT('Ctrl Pts',(1.3406748518516,1.,1.68086176030308));
#24793=CARTESIAN_POINT('Ctrl Pts',(1.33960273470372,1.,1.67458429426126));
#24794=CARTESIAN_POINT('Ctrl Pts',(1.33849388654458,1.,1.66832460784078));
#24795=CARTESIAN_POINT('Ctrl Pts',(1.33734820885331,1.,1.66208312542073));
#24796=CARTESIAN_POINT('Ctrl Pts',(1.33616559745217,1.,1.65586025952651));
#24797=CARTESIAN_POINT('Ctrl Pts',(1.33494590468003,1.,1.64965637286843));
#24798=CARTESIAN_POINT('Ctrl Pts',(1.33368890676554,1.,1.64347174856007));
#24799=CARTESIAN_POINT('Ctrl Pts',(1.33239425103694,1.,1.6373065347505));
#24800=CARTESIAN_POINT('Ctrl Pts',(1.33106149345618,1.,1.63116079730887));
#24801=CARTESIAN_POINT('Ctrl Pts',(1.32969019505665,1.,1.62503464209777));
#24802=CARTESIAN_POINT('Ctrl Pts',(1.32828000610448,1.,1.61892832270723));
#24803=CARTESIAN_POINT('Ctrl Pts',(1.32683074483365,1.,1.61284234015762));
#24804=CARTESIAN_POINT('Ctrl Pts',(1.32534250785794,1.,1.6067775829097));
#24805=CARTESIAN_POINT('Ctrl Pts',(1.32381550858266,1.,1.600735118587));
#24806=CARTESIAN_POINT('Ctrl Pts',(1.32224985747686,1.,1.59471591079408));
#24807=CARTESIAN_POINT('Ctrl Pts',(1.32064537110891,1.,1.58872057258244));
#24808=CARTESIAN_POINT('Ctrl Pts',(1.31900135021428,1.,1.58274907898829));
#24809=CARTESIAN_POINT('Ctrl Pts',(1.31731642317183,1.,1.57680056505585));
#24810=CARTESIAN_POINT('Ctrl Pts',(1.31558903860015,1.,1.57087397835721));
#24811=CARTESIAN_POINT('Ctrl Pts',(1.31381795281002,1.,1.56496872402352));
#24812=CARTESIAN_POINT('Ctrl Pts',(1.31200264341696,1.,1.55908521254822));
#24813=CARTESIAN_POINT('Ctrl Pts',(1.31014393684221,1.,1.55322568759481));
#24814=CARTESIAN_POINT('Ctrl Pts',(1.30824393907471,1.,1.54739413957183));
#24815=CARTESIAN_POINT('Ctrl Pts',(1.30630475189553,1.,1.54159462645428));
#24816=CARTESIAN_POINT('Ctrl Pts',(1.30432735639487,1.,1.53582981268976));
#24817=CARTESIAN_POINT('Ctrl Pts',(1.3023106439557,1.,1.53009970283893));
#24818=CARTESIAN_POINT('Ctrl Pts',(1.30024984366334,1.,1.5243995786107));
#24819=CARTESIAN_POINT('Ctrl Pts',(1.29813791800757,1.,1.51872184912735));
#24820=CARTESIAN_POINT('Ctrl Pts',(1.29596850710518,1.,1.51305994241412));
#24821=CARTESIAN_POINT('Ctrl Pts',(1.29373841372843,1.,1.50741159078367));
#24822=CARTESIAN_POINT('Ctrl Pts',(1.29145022885171,1.,1.50178230149764));
#24823=CARTESIAN_POINT('Ctrl Pts',(1.28911506584232,1.,1.49618896881729));
#24824=CARTESIAN_POINT('Ctrl Pts',(1.28674676116415,1.,1.4906522831275));
#24825=CARTESIAN_POINT('Ctrl Pts',(1.28435533880184,1.,1.48518817118891));
#24826=CARTESIAN_POINT('Ctrl Pts',(1.28194158939522,1.,1.47980070347102));
#24827=CARTESIAN_POINT('Ctrl Pts',(1.27948918248524,1.,1.4744717526711));
#24828=CARTESIAN_POINT('Ctrl Pts',(1.27696414831144,1.,1.46916035917197));
#24829=CARTESIAN_POINT('Ctrl Pts',(1.27433119897877,1.,1.4638243133254));
#24830=CARTESIAN_POINT('Ctrl Pts',(1.27156805265312,1.,1.45843906294725));
#24831=CARTESIAN_POINT('Ctrl Pts',(1.26867786804854,1.,1.45301422764205));
#24832=CARTESIAN_POINT('Ctrl Pts',(1.26570925118767,1.,1.44761985001544));
#24833=CARTESIAN_POINT('Ctrl Pts',(1.26273903323723,1.,1.44236470511145));
#24834=CARTESIAN_POINT('Ctrl Pts',(1.25983531011894,1.,1.43734919180719));
#24835=CARTESIAN_POINT('Ctrl Pts',(1.25702687965744,1.,1.43262645609679));
#24836=CARTESIAN_POINT('Ctrl Pts',(1.25426945222783,1.,1.42815938799555));
#24837=CARTESIAN_POINT('Ctrl Pts',(1.25141455570299,1.,1.42378102115911));
#24838=CARTESIAN_POINT('Ctrl Pts',(1.24824430986911,1.,1.41923722596421));
#24839=CARTESIAN_POINT('Ctrl Pts',(1.24450600513278,1.,1.41422913175437));
#24840=CARTESIAN_POINT('Ctrl Pts',(1.23994455029421,1.,1.40845295531151));
#24841=CARTESIAN_POINT('Ctrl Pts',(1.23434087289768,1.,1.40164708205345));
#24842=CARTESIAN_POINT('Ctrl Pts',(1.22752961898063,1.,1.39361389567257));
#24843=CARTESIAN_POINT('Ctrl Pts',(1.21938737278853,1.,1.38420564525391));
#24844=CARTESIAN_POINT('Ctrl Pts',(1.20982812923113,1.,1.37331915604962));
#24845=CARTESIAN_POINT('Ctrl Pts',(1.1987959077656,1.,1.36088705040677));
#24846=CARTESIAN_POINT('Ctrl Pts',(1.18625865664915,1.,1.34687053998157));
#24847=CARTESIAN_POINT('Ctrl Pts',(1.17501305787994,1.,1.33437539344842));
#24848=CARTESIAN_POINT('Ctrl Pts',(1.16589330092532,1.,1.32428080720544));
#24849=CARTESIAN_POINT('Ctrl Pts',(1.15950888730433,1.,1.3172297721596));
#24850=CARTESIAN_POINT('Ctrl Pts',(1.15624053661742,1.,1.31362392696033));
#24851=CARTESIAN_POINT('',(1.34869019493419,0.,1.73811241238545));
#24852=CARTESIAN_POINT('Origin',(1.23627494547115,0.,1.81978687191668));
#24853=CARTESIAN_POINT('',(1.23627494547115,1.,1.81978687191668));
#24854=CARTESIAN_POINT('',(1.34869019493419,1.,1.73811241238545));
#24855=CARTESIAN_POINT('',(1.23627494547115,0.,1.81978687191668));
#24856=CARTESIAN_POINT('Ctrl Pts',(0.892032620296855,-1.,1.5055822144029));
#24857=CARTESIAN_POINT('Ctrl Pts',(0.892032620296855,1.,1.5055822144029));
#24858=CARTESIAN_POINT('Ctrl Pts',(0.894452006967538,-1.,1.50980486807181));
#24859=CARTESIAN_POINT('Ctrl Pts',(0.894452006967538,1.,1.50980486807181));
#24860=CARTESIAN_POINT('Ctrl Pts',(0.89918504749193,-1.,1.51805569591479));
#24861=CARTESIAN_POINT('Ctrl Pts',(0.89918504749193,1.,1.51805569591479));
#24862=CARTESIAN_POINT('Ctrl Pts',(0.905967409640498,-1.,1.52984849890434));
#24863=CARTESIAN_POINT('Ctrl Pts',(0.905967409640498,1.,1.52984849890434));
#24864=CARTESIAN_POINT('Ctrl Pts',(0.914375919046579,-1.,1.54440491152808));
#24865=CARTESIAN_POINT('Ctrl Pts',(0.914375919046579,1.,1.54440491152808));
#24866=CARTESIAN_POINT('Ctrl Pts',(0.923832188966322,-1.,1.56065988582509));
#24867=CARTESIAN_POINT('Ctrl Pts',(0.923832188966322,1.,1.56065988582509));
#24868=CARTESIAN_POINT('Ctrl Pts',(0.932246680128848,-1.,1.57499388385561));
#24869=CARTESIAN_POINT('Ctrl Pts',(0.932246680128848,1.,1.57499388385561));
#24870=CARTESIAN_POINT('Ctrl Pts',(0.939646377909319,-1.,1.58744937489796));
#24871=CARTESIAN_POINT('Ctrl Pts',(0.939646377909319,1.,1.58744937489796));
#24872=CARTESIAN_POINT('Ctrl Pts',(0.946078063325795,-1.,1.59810042045408));
#24873=CARTESIAN_POINT('Ctrl Pts',(0.946078063325795,1.,1.59810042045408));
#24874=CARTESIAN_POINT('Ctrl Pts',(0.951613284361247,-1.,1.60706069897794));
#24875=CARTESIAN_POINT('Ctrl Pts',(0.951613284361247,1.,1.60706069897794));
#24876=CARTESIAN_POINT('Ctrl Pts',(0.956354422921572,-1.,1.61449324337233));
#24877=CARTESIAN_POINT('Ctrl Pts',(0.956354422921572,1.,1.61449324337233));
#24878=CARTESIAN_POINT('Ctrl Pts',(0.960438326099958,-1.,1.62061638139929));
#24879=CARTESIAN_POINT('Ctrl Pts',(0.960438326099958,1.,1.62061638139929));
#24880=CARTESIAN_POINT('Ctrl Pts',(0.964046107037821,-1.,1.6257193066974));
#24881=CARTESIAN_POINT('Ctrl Pts',(0.964046107037821,1.,1.6257193066974));
#24882=CARTESIAN_POINT('Ctrl Pts',(0.967387853228041,-1.,1.63013849959083));
#24883=CARTESIAN_POINT('Ctrl Pts',(0.967387853228041,1.,1.63013849959083));
#24884=CARTESIAN_POINT('Ctrl Pts',(0.970669715996356,-1.,1.63420665729609));
#24885=CARTESIAN_POINT('Ctrl Pts',(0.970669715996356,1.,1.63420665729609));
#24886=CARTESIAN_POINT('Ctrl Pts',(0.974066058287501,-1.,1.63820952658157));
#24887=CARTESIAN_POINT('Ctrl Pts',(0.974066058287501,1.,1.63820952658157));
#24888=CARTESIAN_POINT('Ctrl Pts',(0.977689794120296,-1.,1.64233990826831));
#24889=CARTESIAN_POINT('Ctrl Pts',(0.977689794120296,1.,1.64233990826831));
#24890=CARTESIAN_POINT('Ctrl Pts',(0.981562530940574,-1.,1.64665139190834));
#24891=CARTESIAN_POINT('Ctrl Pts',(0.981562530940574,1.,1.64665139190834));
#24892=CARTESIAN_POINT('Ctrl Pts',(0.985642622921626,-1.,1.6511001661277));
#24893=CARTESIAN_POINT('Ctrl Pts',(0.985642622921626,1.,1.6511001661277));
#24894=CARTESIAN_POINT('Ctrl Pts',(0.98985562785445,-1.,1.65559044289746));
#24895=CARTESIAN_POINT('Ctrl Pts',(0.98985562785445,1.,1.65559044289746));
#24896=CARTESIAN_POINT('Ctrl Pts',(0.994121836661115,-1.,1.66001553809916));
#24897=CARTESIAN_POINT('Ctrl Pts',(0.994121836661115,1.,1.66001553809916));
#24898=CARTESIAN_POINT('Ctrl Pts',(0.998389654952317,-1.,1.66430758030304));
#24899=CARTESIAN_POINT('Ctrl Pts',(0.998389654952317,1.,1.66430758030304));
#24900=CARTESIAN_POINT('Ctrl Pts',(1.00265091003682,-1.,1.66846059277231));
#24901=CARTESIAN_POINT('Ctrl Pts',(1.00265091003682,1.,1.66846059277231));
#24902=CARTESIAN_POINT('Ctrl Pts',(1.00692206696387,-1.,1.67250335383248));
#24903=CARTESIAN_POINT('Ctrl Pts',(1.00692206696387,1.,1.67250335383248));
#24904=CARTESIAN_POINT('Ctrl Pts',(1.01123236493507,-1.,1.67648246776457));
#24905=CARTESIAN_POINT('Ctrl Pts',(1.01123236493507,1.,1.67648246776457));
#24906=CARTESIAN_POINT('Ctrl Pts',(1.01561026162786,-1.,1.6804428989482));
#24907=CARTESIAN_POINT('Ctrl Pts',(1.01561026162786,1.,1.6804428989482));
#24908=CARTESIAN_POINT('Ctrl Pts',(1.02006795074222,-1.,1.68440578021739));
#24909=CARTESIAN_POINT('Ctrl Pts',(1.02006795074222,1.,1.68440578021739));
#24910=CARTESIAN_POINT('Ctrl Pts',(1.02460180535272,-1.,1.68836910178475));
#24911=CARTESIAN_POINT('Ctrl Pts',(1.02460180535272,1.,1.68836910178475));
#24912=CARTESIAN_POINT('Ctrl Pts',(1.02919977579155,-1.,1.69231840863471));
#24913=CARTESIAN_POINT('Ctrl Pts',(1.02919977579155,1.,1.69231840863471));
#24914=CARTESIAN_POINT('Ctrl Pts',(1.03384646003587,-1.,1.69623414782769));
#24915=CARTESIAN_POINT('Ctrl Pts',(1.03384646003587,1.,1.69623414782769));
#24916=CARTESIAN_POINT('Ctrl Pts',(1.03852922490782,-1.,1.70010052930951));
#24917=CARTESIAN_POINT('Ctrl Pts',(1.03852922490782,1.,1.70010052930951));
#24918=CARTESIAN_POINT('Ctrl Pts',(1.04324363334546,-1.,1.70391338707969));
#24919=CARTESIAN_POINT('Ctrl Pts',(1.04324363334546,1.,1.70391338707969));
#24920=CARTESIAN_POINT('Ctrl Pts',(1.0479908540499,-1.,1.70767646263641));
#24921=CARTESIAN_POINT('Ctrl Pts',(1.0479908540499,1.,1.70767646263641));
#24922=CARTESIAN_POINT('Ctrl Pts',(1.05277517202853,-1.,1.71139783543986));
#24923=CARTESIAN_POINT('Ctrl Pts',(1.05277517202853,1.,1.71139783543986));
#24924=CARTESIAN_POINT('Ctrl Pts',(1.05760163192481,-1.,1.71508654427022));
#24925=CARTESIAN_POINT('Ctrl Pts',(1.05760163192481,1.,1.71508654427022));
#24926=CARTESIAN_POINT('Ctrl Pts',(1.06247324680649,-1.,1.71874858456908));
#24927=CARTESIAN_POINT('Ctrl Pts',(1.06247324680649,1.,1.71874858456908));
#24928=CARTESIAN_POINT('Ctrl Pts',(1.06738966975463,-1.,1.72238500928456));
#24929=CARTESIAN_POINT('Ctrl Pts',(1.06738966975463,1.,1.72238500928456));
#24930=CARTESIAN_POINT('Ctrl Pts',(1.07234866990252,-1.,1.72599406198489));
#24931=CARTESIAN_POINT('Ctrl Pts',(1.07234866990252,1.,1.72599406198489));
#24932=CARTESIAN_POINT('Ctrl Pts',(1.0773470373727,-1.,1.72957248977424));
#24933=CARTESIAN_POINT('Ctrl Pts',(1.0773470373727,1.,1.72957248977424));
#24934=CARTESIAN_POINT('Ctrl Pts',(1.08238162784749,-1.,1.73311705663407));
#24935=CARTESIAN_POINT('Ctrl Pts',(1.08238162784749,1.,1.73311705663407));
#24936=CARTESIAN_POINT('Ctrl Pts',(1.08745056285429,-1.,1.73662628326093));
#24937=CARTESIAN_POINT('Ctrl Pts',(1.08745056285429,1.,1.73662628326093));
#24938=CARTESIAN_POINT('Ctrl Pts',(1.09255329056496,-1.,1.74010053962252));
#24939=CARTESIAN_POINT('Ctrl Pts',(1.09255329056496,1.,1.74010053962252));
#24940=CARTESIAN_POINT('Ctrl Pts',(1.09768999241229,-1.,1.74354119236212));
#24941=CARTESIAN_POINT('Ctrl Pts',(1.09768999241229,1.,1.74354119236212));
#24942=CARTESIAN_POINT('Ctrl Pts',(1.10286118991144,-1.,1.74695004214924));
#24943=CARTESIAN_POINT('Ctrl Pts',(1.10286118991144,1.,1.74695004214924));
#24944=CARTESIAN_POINT('Ctrl Pts',(1.10806728183003,-1.,1.75032866075914));
#24945=CARTESIAN_POINT('Ctrl Pts',(1.10806728183003,1.,1.75032866075914));
#24946=CARTESIAN_POINT('Ctrl Pts',(1.11330807582542,-1.,1.75367772094617));
#24947=CARTESIAN_POINT('Ctrl Pts',(1.11330807582542,1.,1.75367772094617));
#24948=CARTESIAN_POINT('Ctrl Pts',(1.11858293216752,-1.,1.75699720772089));
#24949=CARTESIAN_POINT('Ctrl Pts',(1.11858293216752,1.,1.75699720772089));
#24950=CARTESIAN_POINT('Ctrl Pts',(1.12389096855078,-1.,1.76028671825084));
#24951=CARTESIAN_POINT('Ctrl Pts',(1.12389096855078,1.,1.76028671825084));
#24952=CARTESIAN_POINT('Ctrl Pts',(1.12923123555076,-1.,1.76354571966171));
#24953=CARTESIAN_POINT('Ctrl Pts',(1.12923123555076,1.,1.76354571966171));
#24954=CARTESIAN_POINT('Ctrl Pts',(1.13460291804634,-1.,1.76677384551883));
#24955=CARTESIAN_POINT('Ctrl Pts',(1.13460291804634,1.,1.76677384551883));
#24956=CARTESIAN_POINT('Ctrl Pts',(1.14000548337,-1.,1.76997111386806));
#24957=CARTESIAN_POINT('Ctrl Pts',(1.14000548337,1.,1.76997111386806));
#24958=CARTESIAN_POINT('Ctrl Pts',(1.14543858226948,-1.,1.77313777896234));
#24959=CARTESIAN_POINT('Ctrl Pts',(1.14543858226948,1.,1.77313777896234));
#24960=CARTESIAN_POINT('Ctrl Pts',(1.15090197841531,-1.,1.77627422557034));
#24961=CARTESIAN_POINT('Ctrl Pts',(1.15090197841531,1.,1.77627422557034));
#24962=CARTESIAN_POINT('Ctrl Pts',(1.15639547194689,-1.,1.77938085564261));
#24963=CARTESIAN_POINT('Ctrl Pts',(1.15639547194689,1.,1.77938085564261));
#24964=CARTESIAN_POINT('Ctrl Pts',(1.16191881298458,-1.,1.78245795880949));
#24965=CARTESIAN_POINT('Ctrl Pts',(1.16191881298458,1.,1.78245795880949));
#24966=CARTESIAN_POINT('Ctrl Pts',(1.16747166312239,-1.,1.78550566040349));
#24967=CARTESIAN_POINT('Ctrl Pts',(1.16747166312239,1.,1.78550566040349));
#24968=CARTESIAN_POINT('Ctrl Pts',(1.17305363177265,-1.,1.78852398877523));
#24969=CARTESIAN_POINT('Ctrl Pts',(1.17305363177265,1.,1.78852398877523));
#24970=CARTESIAN_POINT('Ctrl Pts',(1.17866429440781,-1.,1.79151291552646));
#24971=CARTESIAN_POINT('Ctrl Pts',(1.17866429440781,1.,1.79151291552646));
#24972=CARTESIAN_POINT('Ctrl Pts',(1.18430321697471,-1.,1.79447240321572));
#24973=CARTESIAN_POINT('Ctrl Pts',(1.18430321697471,1.,1.79447240321572));
#24974=CARTESIAN_POINT('Ctrl Pts',(1.1899699793456,-1.,1.79740245923649));
#24975=CARTESIAN_POINT('Ctrl Pts',(1.1899699793456,1.,1.79740245923649));
#24976=CARTESIAN_POINT('Ctrl Pts',(1.19566418930405,-1.,1.80030314370121));
#24977=CARTESIAN_POINT('Ctrl Pts',(1.19566418930405,1.,1.80030314370121));
#24978=CARTESIAN_POINT('Ctrl Pts',(1.2013854893912,-1.,1.8031745483882));
#24979=CARTESIAN_POINT('Ctrl Pts',(1.2013854893912,1.,1.8031745483882));
#24980=CARTESIAN_POINT('Ctrl Pts',(1.20713356605519,-1.,1.80601678480772));
#24981=CARTESIAN_POINT('Ctrl Pts',(1.20713356605519,1.,1.80601678480772));
#24982=CARTESIAN_POINT('Ctrl Pts',(1.2129081570818,-1.,1.80882996916931));
#24983=CARTESIAN_POINT('Ctrl Pts',(1.2129081570818,1.,1.80882996916931));
#24984=CARTESIAN_POINT('Ctrl Pts',(1.2187090610323,-1.,1.81161420806172));
#24985=CARTESIAN_POINT('Ctrl Pts',(1.2187090610323,1.,1.81161420806172));
#24986=CARTESIAN_POINT('Ctrl Pts',(1.22453613304507,-1.,1.81436959209778));
#24987=CARTESIAN_POINT('Ctrl Pts',(1.22453613304507,1.,1.81436959209778));
#24988=CARTESIAN_POINT('Ctrl Pts',(1.22921864890975,-1.,1.81655087183054));
#24989=CARTESIAN_POINT('Ctrl Pts',(1.22921864890975,1.,1.81655087183054));
#24990=CARTESIAN_POINT('Ctrl Pts',(1.23274224526804,-1.,1.81817389920914));
#24991=CARTESIAN_POINT('Ctrl Pts',(1.23274224526804,1.,1.81817389920914));
#24992=CARTESIAN_POINT('Ctrl Pts',(1.23509651170384,-1.,1.81925017193531));
#24993=CARTESIAN_POINT('Ctrl Pts',(1.23509651170384,1.,1.81925017193531));
#24994=CARTESIAN_POINT('Ctrl Pts',(1.23627494547115,-1.,1.81978687191668));
#24995=CARTESIAN_POINT('Ctrl Pts',(1.23627494547115,1.,1.81978687191668));
#24996=CARTESIAN_POINT('',(0.892032620296855,1.,1.5055822144029));
#24997=CARTESIAN_POINT('Ctrl Pts',(0.892032620296855,1.,1.5055822144029));
#24998=CARTESIAN_POINT('Ctrl Pts',(0.894452006967538,1.,1.50980486807181));
#24999=CARTESIAN_POINT('Ctrl Pts',(0.89918504749193,1.,1.51805569591479));
#25000=CARTESIAN_POINT('Ctrl Pts',(0.905967409640498,1.,1.52984849890434));
#25001=CARTESIAN_POINT('Ctrl Pts',(0.914375919046579,1.,1.54440491152808));
#25002=CARTESIAN_POINT('Ctrl Pts',(0.923832188966322,1.,1.56065988582509));
#25003=CARTESIAN_POINT('Ctrl Pts',(0.932246680128848,1.,1.57499388385561));
#25004=CARTESIAN_POINT('Ctrl Pts',(0.939646377909319,1.,1.58744937489796));
#25005=CARTESIAN_POINT('Ctrl Pts',(0.946078063325795,1.,1.59810042045408));
#25006=CARTESIAN_POINT('Ctrl Pts',(0.951613284361247,1.,1.60706069897794));
#25007=CARTESIAN_POINT('Ctrl Pts',(0.956354422921572,1.,1.61449324337233));
#25008=CARTESIAN_POINT('Ctrl Pts',(0.960438326099958,1.,1.62061638139929));
#25009=CARTESIAN_POINT('Ctrl Pts',(0.964046107037821,1.,1.6257193066974));
#25010=CARTESIAN_POINT('Ctrl Pts',(0.967387853228041,1.,1.63013849959083));
#25011=CARTESIAN_POINT('Ctrl Pts',(0.970669715996356,1.,1.63420665729609));
#25012=CARTESIAN_POINT('Ctrl Pts',(0.974066058287501,1.,1.63820952658157));
#25013=CARTESIAN_POINT('Ctrl Pts',(0.977689794120296,1.,1.64233990826831));
#25014=CARTESIAN_POINT('Ctrl Pts',(0.981562530940574,1.,1.64665139190834));
#25015=CARTESIAN_POINT('Ctrl Pts',(0.985642622921626,1.,1.6511001661277));
#25016=CARTESIAN_POINT('Ctrl Pts',(0.98985562785445,1.,1.65559044289746));
#25017=CARTESIAN_POINT('Ctrl Pts',(0.994121836661115,1.,1.66001553809916));
#25018=CARTESIAN_POINT('Ctrl Pts',(0.998389654952317,1.,1.66430758030304));
#25019=CARTESIAN_POINT('Ctrl Pts',(1.00265091003682,1.,1.66846059277231));
#25020=CARTESIAN_POINT('Ctrl Pts',(1.00692206696387,1.,1.67250335383248));
#25021=CARTESIAN_POINT('Ctrl Pts',(1.01123236493507,1.,1.67648246776457));
#25022=CARTESIAN_POINT('Ctrl Pts',(1.01561026162786,1.,1.6804428989482));
#25023=CARTESIAN_POINT('Ctrl Pts',(1.02006795074222,1.,1.68440578021739));
#25024=CARTESIAN_POINT('Ctrl Pts',(1.02460180535272,1.,1.68836910178475));
#25025=CARTESIAN_POINT('Ctrl Pts',(1.02919977579155,1.,1.69231840863471));
#25026=CARTESIAN_POINT('Ctrl Pts',(1.03384646003587,1.,1.69623414782769));
#25027=CARTESIAN_POINT('Ctrl Pts',(1.03852922490782,1.,1.70010052930951));
#25028=CARTESIAN_POINT('Ctrl Pts',(1.04324363334546,1.,1.70391338707969));
#25029=CARTESIAN_POINT('Ctrl Pts',(1.0479908540499,1.,1.70767646263641));
#25030=CARTESIAN_POINT('Ctrl Pts',(1.05277517202853,1.,1.71139783543986));
#25031=CARTESIAN_POINT('Ctrl Pts',(1.05760163192481,1.,1.71508654427022));
#25032=CARTESIAN_POINT('Ctrl Pts',(1.06247324680649,1.,1.71874858456908));
#25033=CARTESIAN_POINT('Ctrl Pts',(1.06738966975463,1.,1.72238500928456));
#25034=CARTESIAN_POINT('Ctrl Pts',(1.07234866990252,1.,1.72599406198489));
#25035=CARTESIAN_POINT('Ctrl Pts',(1.0773470373727,1.,1.72957248977424));
#25036=CARTESIAN_POINT('Ctrl Pts',(1.08238162784749,1.,1.73311705663407));
#25037=CARTESIAN_POINT('Ctrl Pts',(1.08745056285429,1.,1.73662628326093));
#25038=CARTESIAN_POINT('Ctrl Pts',(1.09255329056496,1.,1.74010053962252));
#25039=CARTESIAN_POINT('Ctrl Pts',(1.09768999241229,1.,1.74354119236212));
#25040=CARTESIAN_POINT('Ctrl Pts',(1.10286118991144,1.,1.74695004214924));
#25041=CARTESIAN_POINT('Ctrl Pts',(1.10806728183003,1.,1.75032866075914));
#25042=CARTESIAN_POINT('Ctrl Pts',(1.11330807582542,1.,1.75367772094617));
#25043=CARTESIAN_POINT('Ctrl Pts',(1.11858293216752,1.,1.75699720772089));
#25044=CARTESIAN_POINT('Ctrl Pts',(1.12389096855078,1.,1.76028671825084));
#25045=CARTESIAN_POINT('Ctrl Pts',(1.12923123555076,1.,1.76354571966171));
#25046=CARTESIAN_POINT('Ctrl Pts',(1.13460291804634,1.,1.76677384551883));
#25047=CARTESIAN_POINT('Ctrl Pts',(1.14000548337,1.,1.76997111386806));
#25048=CARTESIAN_POINT('Ctrl Pts',(1.14543858226948,1.,1.77313777896234));
#25049=CARTESIAN_POINT('Ctrl Pts',(1.15090197841531,1.,1.77627422557034));
#25050=CARTESIAN_POINT('Ctrl Pts',(1.15639547194689,1.,1.77938085564261));
#25051=CARTESIAN_POINT('Ctrl Pts',(1.16191881298458,1.,1.78245795880949));
#25052=CARTESIAN_POINT('Ctrl Pts',(1.16747166312239,1.,1.78550566040349));
#25053=CARTESIAN_POINT('Ctrl Pts',(1.17305363177265,1.,1.78852398877523));
#25054=CARTESIAN_POINT('Ctrl Pts',(1.17866429440781,1.,1.79151291552646));
#25055=CARTESIAN_POINT('Ctrl Pts',(1.18430321697471,1.,1.79447240321572));
#25056=CARTESIAN_POINT('Ctrl Pts',(1.1899699793456,1.,1.79740245923649));
#25057=CARTESIAN_POINT('Ctrl Pts',(1.19566418930405,1.,1.80030314370121));
#25058=CARTESIAN_POINT('Ctrl Pts',(1.2013854893912,1.,1.8031745483882));
#25059=CARTESIAN_POINT('Ctrl Pts',(1.20713356605519,1.,1.80601678480772));
#25060=CARTESIAN_POINT('Ctrl Pts',(1.2129081570818,1.,1.80882996916931));
#25061=CARTESIAN_POINT('Ctrl Pts',(1.2187090610323,1.,1.81161420806172));
#25062=CARTESIAN_POINT('Ctrl Pts',(1.22453613304507,1.,1.81436959209778));
#25063=CARTESIAN_POINT('Ctrl Pts',(1.22921864890975,1.,1.81655087183054));
#25064=CARTESIAN_POINT('Ctrl Pts',(1.23274224526804,1.,1.81817389920914));
#25065=CARTESIAN_POINT('Ctrl Pts',(1.23509651170384,1.,1.81925017193531));
#25066=CARTESIAN_POINT('Ctrl Pts',(1.23627494547115,1.,1.81978687191668));
#25067=CARTESIAN_POINT('',(0.892032620296854,0.,1.5055822144029));
#25068=CARTESIAN_POINT('Origin',(0.,0.,0.));
#25069=CARTESIAN_POINT('',(0.693717979106305,1.,1.60662857109684));
#25070=CARTESIAN_POINT('Origin',(0.,1.,0.));
#25071=CARTESIAN_POINT('',(0.693717979106305,0.,1.60662857109684));
#25072=CARTESIAN_POINT('Ctrl Pts',(0.7455743247944,-1.,2.0698113262342));
#25073=CARTESIAN_POINT('Ctrl Pts',(0.7455743247944,1.,2.0698113262342));
#25074=CARTESIAN_POINT('Ctrl Pts',(0.745832791378367,-1.,2.06854248895728));
#25075=CARTESIAN_POINT('Ctrl Pts',(0.745832791378367,1.,2.06854248895728));
#25076=CARTESIAN_POINT('Ctrl Pts',(0.7463458715442,-1.,2.06600523016815));
#25077=CARTESIAN_POINT('Ctrl Pts',(0.7463458715442,1.,2.06600523016815));
#25078=CARTESIAN_POINT('Ctrl Pts',(0.747103932787919,-1.,2.06220058927826));
#25079=CARTESIAN_POINT('Ctrl Pts',(0.747103932787919,1.,2.06220058927826));
#25080=CARTESIAN_POINT('Ctrl Pts',(0.748091554183802,-1.,2.05713023031007));
#25081=CARTESIAN_POINT('Ctrl Pts',(0.748091554183802,1.,2.05713023031007));
#25082=CARTESIAN_POINT('Ctrl Pts',(0.749287468665046,-1.,2.05079645592154));
#25083=CARTESIAN_POINT('Ctrl Pts',(0.749287468665046,1.,2.05079645592154));
#25084=CARTESIAN_POINT('Ctrl Pts',(0.750444657875575,-1.,2.04446689147979));
#25085=CARTESIAN_POINT('Ctrl Pts',(0.750444657875575,1.,2.04446689147979));
#25086=CARTESIAN_POINT('Ctrl Pts',(0.751562963361115,-1.,2.03814160092099));
#25087=CARTESIAN_POINT('Ctrl Pts',(0.751562963361115,1.,2.03814160092099));
#25088=CARTESIAN_POINT('Ctrl Pts',(0.75264218048721,-1.,2.03182068456221));
#25089=CARTESIAN_POINT('Ctrl Pts',(0.75264218048721,1.,2.03182068456221));
#25090=CARTESIAN_POINT('Ctrl Pts',(0.753682061112768,-1.,2.02550428623313));
#25091=CARTESIAN_POINT('Ctrl Pts',(0.753682061112768,1.,2.02550428623313));
#25092=CARTESIAN_POINT('Ctrl Pts',(0.754682330722816,-1.,2.01919259405809));
#25093=CARTESIAN_POINT('Ctrl Pts',(0.754682330722816,1.,2.01919259405809));
#25094=CARTESIAN_POINT('Ctrl Pts',(0.755642704957865,-1.,2.01288584328084));
#25095=CARTESIAN_POINT('Ctrl Pts',(0.755642704957865,1.,2.01288584328084));
#25096=CARTESIAN_POINT('Ctrl Pts',(0.75656290464667,-1.,2.0065843158773));
#25097=CARTESIAN_POINT('Ctrl Pts',(0.75656290464667,1.,2.0065843158773));
#25098=CARTESIAN_POINT('Ctrl Pts',(0.757442676862724,-1.,2.00028834739178));
#25099=CARTESIAN_POINT('Ctrl Pts',(0.757442676862724,1.,2.00028834739178));
#25100=CARTESIAN_POINT('Ctrl Pts',(0.758281796766761,-1.,1.99399831098817));
#25101=CARTESIAN_POINT('Ctrl Pts',(0.758281796766761,1.,1.99399831098817));
#25102=CARTESIAN_POINT('Ctrl Pts',(0.759080037802488,-1.,1.98771456680874));
#25103=CARTESIAN_POINT('Ctrl Pts',(0.759080037802488,1.,1.98771456680874));
#25104=CARTESIAN_POINT('Ctrl Pts',(0.75983714745219,-1.,1.98143741418172));
#25105=CARTESIAN_POINT('Ctrl Pts',(0.75983714745219,1.,1.98143741418172));
#25106=CARTESIAN_POINT('Ctrl Pts',(0.760552825409757,-1.,1.97516705321494));
#25107=CARTESIAN_POINT('Ctrl Pts',(0.760552825409757,1.,1.97516705321494));
#25108=CARTESIAN_POINT('Ctrl Pts',(0.76122669048382,-1.,1.96890351582499));
#25109=CARTESIAN_POINT('Ctrl Pts',(0.76122669048382,1.,1.96890351582499));
#25110=CARTESIAN_POINT('Ctrl Pts',(0.761858300014423,-1.,1.96264672744186));
#25111=CARTESIAN_POINT('Ctrl Pts',(0.761858300014423,1.,1.96264672744186));
#25112=CARTESIAN_POINT('Ctrl Pts',(0.762447203806178,-1.,1.95639665309869));
#25113=CARTESIAN_POINT('Ctrl Pts',(0.762447203806178,1.,1.95639665309869));
#25114=CARTESIAN_POINT('Ctrl Pts',(0.762992990878769,-1.,1.95015342590024));
#25115=CARTESIAN_POINT('Ctrl Pts',(0.762992990878769,1.,1.95015342590024));
#25116=CARTESIAN_POINT('Ctrl Pts',(0.763495333538629,-1.,1.9439174661764));
#25117=CARTESIAN_POINT('Ctrl Pts',(0.763495333538629,1.,1.9439174661764));
#25118=CARTESIAN_POINT('Ctrl Pts',(0.763954049121458,-1.,1.93768964875886));
#25119=CARTESIAN_POINT('Ctrl Pts',(0.763954049121458,1.,1.93768964875886));
#25120=CARTESIAN_POINT('Ctrl Pts',(0.76436901067394,-1.,1.93147105496382));
#25121=CARTESIAN_POINT('Ctrl Pts',(0.76436901067394,1.,1.93147105496382));
#25122=CARTESIAN_POINT('Ctrl Pts',(0.764740025488211,-1.,1.92526263537048));
#25123=CARTESIAN_POINT('Ctrl Pts',(0.764740025488211,1.,1.92526263537048));
#25124=CARTESIAN_POINT('Ctrl Pts',(0.765066729667088,-1.,1.91906491634196));
#25125=CARTESIAN_POINT('Ctrl Pts',(0.765066729667088,1.,1.91906491634196));
#25126=CARTESIAN_POINT('Ctrl Pts',(0.765348465884722,-1.,1.91287765805169));
#25127=CARTESIAN_POINT('Ctrl Pts',(0.765348465884722,1.,1.91287765805169));
#25128=CARTESIAN_POINT('Ctrl Pts',(0.765584196937919,-1.,1.90669961402356));
#25129=CARTESIAN_POINT('Ctrl Pts',(0.765584196937919,1.,1.90669961402356));
#25130=CARTESIAN_POINT('Ctrl Pts',(0.765772772593386,-1.,1.90052930393596));
#25131=CARTESIAN_POINT('Ctrl Pts',(0.765772772593386,1.,1.90052930393596));
#25132=CARTESIAN_POINT('Ctrl Pts',(0.765913193856978,-1.,1.89436577771388));
#25133=CARTESIAN_POINT('Ctrl Pts',(0.765913193856978,1.,1.89436577771388));
#25134=CARTESIAN_POINT('Ctrl Pts',(0.766004837062091,-1.,1.88820926433409));
#25135=CARTESIAN_POINT('Ctrl Pts',(0.766004837062091,1.,1.88820926433409));
#25136=CARTESIAN_POINT('Ctrl Pts',(0.766047794851864,-1.,1.88206215302561));
#25137=CARTESIAN_POINT('Ctrl Pts',(0.766047794851864,1.,1.88206215302561));
#25138=CARTESIAN_POINT('Ctrl Pts',(0.766042837036744,-1.,1.87592888967883));
#25139=CARTESIAN_POINT('Ctrl Pts',(0.766042837036744,1.,1.87592888967883));
#25140=CARTESIAN_POINT('Ctrl Pts',(0.765990708546091,-1.,1.86981398314341));
#25141=CARTESIAN_POINT('Ctrl Pts',(0.765990708546091,1.,1.86981398314341));
#25142=CARTESIAN_POINT('Ctrl Pts',(0.765891519092547,-1.,1.86372027063312));
#25143=CARTESIAN_POINT('Ctrl Pts',(0.765891519092547,1.,1.86372027063312));
#25144=CARTESIAN_POINT('Ctrl Pts',(0.765744212909318,-1.,1.85764741390394));
#25145=CARTESIAN_POINT('Ctrl Pts',(0.765744212909318,1.,1.85764741390394));
#25146=CARTESIAN_POINT('Ctrl Pts',(0.765545710619062,-1.,1.85158945130063));
#25147=CARTESIAN_POINT('Ctrl Pts',(0.765545710619062,1.,1.85158945130063));
#25148=CARTESIAN_POINT('Ctrl Pts',(0.765291664862029,-1.,1.84553698875924));
#25149=CARTESIAN_POINT('Ctrl Pts',(0.765291664862029,1.,1.84553698875924));
#25150=CARTESIAN_POINT('Ctrl Pts',(0.764978057881737,-1.,1.83948181064835));
#25151=CARTESIAN_POINT('Ctrl Pts',(0.764978057881737,1.,1.83948181064835));
#25152=CARTESIAN_POINT('Ctrl Pts',(0.764602549687853,-1.,1.83342077227142));
#25153=CARTESIAN_POINT('Ctrl Pts',(0.764602549687853,1.,1.83342077227142));
#25154=CARTESIAN_POINT('Ctrl Pts',(0.764165902605995,-1.,1.82735991200065));
#25155=CARTESIAN_POINT('Ctrl Pts',(0.764165902605995,1.,1.82735991200065));
#25156=CARTESIAN_POINT('Ctrl Pts',(0.763673465462726,-1.,1.82131873145266));
#25157=CARTESIAN_POINT('Ctrl Pts',(0.763673465462726,1.,1.82131873145266));
#25158=CARTESIAN_POINT('Ctrl Pts',(0.763132003836634,-1.,1.8153211840553));
#25159=CARTESIAN_POINT('Ctrl Pts',(0.763132003836634,1.,1.8153211840553));
#25160=CARTESIAN_POINT('Ctrl Pts',(0.762546129463938,-1.,1.80938551463965));
#25161=CARTESIAN_POINT('Ctrl Pts',(0.762546129463938,1.,1.80938551463965));
#25162=CARTESIAN_POINT('Ctrl Pts',(0.761915336443547,-1.,1.80351583877342));
#25163=CARTESIAN_POINT('Ctrl Pts',(0.761915336443547,1.,1.80351583877342));
#25164=CARTESIAN_POINT('Ctrl Pts',(0.761229695230558,-1.,1.79768986997783));
#25165=CARTESIAN_POINT('Ctrl Pts',(0.761229695230558,1.,1.79768986997783));
#25166=CARTESIAN_POINT('Ctrl Pts',(0.760469555880749,-1.,1.7918581561088));
#25167=CARTESIAN_POINT('Ctrl Pts',(0.760469555880749,1.,1.7918581561088));
#25168=CARTESIAN_POINT('Ctrl Pts',(0.759614401110189,-1.,1.78596964884604));
#25169=CARTESIAN_POINT('Ctrl Pts',(0.759614401110189,1.,1.78596964884604));
#25170=CARTESIAN_POINT('Ctrl Pts',(0.758650626677518,-1.,1.77999411220945));
#25171=CARTESIAN_POINT('Ctrl Pts',(0.758650626677518,1.,1.77999411220945));
#25172=CARTESIAN_POINT('Ctrl Pts',(0.757578264077028,-1.,1.77394167108292));
#25173=CARTESIAN_POINT('Ctrl Pts',(0.757578264077028,1.,1.77394167108292));
#25174=CARTESIAN_POINT('Ctrl Pts',(0.75642189602781,-1.,1.76789396002998));
#25175=CARTESIAN_POINT('Ctrl Pts',(0.75642189602781,1.,1.76789396002998));
#25176=CARTESIAN_POINT('Ctrl Pts',(0.755220979974461,-1.,1.76197817240128));
#25177=CARTESIAN_POINT('Ctrl Pts',(0.755220979974461,1.,1.76197817240128));
#25178=CARTESIAN_POINT('Ctrl Pts',(0.754009254027828,-1.,1.75631083600019));
#25179=CARTESIAN_POINT('Ctrl Pts',(0.754009254027828,1.,1.75631083600019));
#25180=CARTESIAN_POINT('Ctrl Pts',(0.752797683531314,-1.,1.75095139468794));
#25181=CARTESIAN_POINT('Ctrl Pts',(0.752797683531314,1.,1.75095139468794));
#25182=CARTESIAN_POINT('Ctrl Pts',(0.751555614164482,-1.,1.74585086852502));
#25183=CARTESIAN_POINT('Ctrl Pts',(0.751555614164482,1.,1.74585086852502));
#25184=CARTESIAN_POINT('Ctrl Pts',(0.750193435981249,-1.,1.74080458267114));
#25185=CARTESIAN_POINT('Ctrl Pts',(0.750193435981249,1.,1.74080458267114));
#25186=CARTESIAN_POINT('Ctrl Pts',(0.74858246295687,-1.,1.7355035168033));
#25187=CARTESIAN_POINT('Ctrl Pts',(0.74858246295687,1.,1.7355035168033));
#25188=CARTESIAN_POINT('Ctrl Pts',(0.746574710097752,-1.,1.72958533647714));
#25189=CARTESIAN_POINT('Ctrl Pts',(0.746574710097752,1.,1.72958533647714));
#25190=CARTESIAN_POINT('Ctrl Pts',(0.744021445433093,-1.,1.72268229916769));
#25191=CARTESIAN_POINT('Ctrl Pts',(0.744021445433093,1.,1.72268229916769));
#25192=CARTESIAN_POINT('Ctrl Pts',(0.74079516202821,-1.,1.71447789751001));
#25193=CARTESIAN_POINT('Ctrl Pts',(0.74079516202821,1.,1.71447789751001));
#25194=CARTESIAN_POINT('Ctrl Pts',(0.736799665716932,-1.,1.70473309004249));
#25195=CARTESIAN_POINT('Ctrl Pts',(0.736799665716932,1.,1.70473309004249));
#25196=CARTESIAN_POINT('Ctrl Pts',(0.731963238685357,-1.,1.69326921972915));
#25197=CARTESIAN_POINT('Ctrl Pts',(0.731963238685357,1.,1.69326921972915));
#25198=CARTESIAN_POINT('Ctrl Pts',(0.726235967982445,-1.,1.67996158451922));
#25199=CARTESIAN_POINT('Ctrl Pts',(0.726235967982445,1.,1.67996158451922));
#25200=CARTESIAN_POINT('Ctrl Pts',(0.719585433787949,-1.,1.66472880551777));
#25201=CARTESIAN_POINT('Ctrl Pts',(0.719585433787949,1.,1.66472880551777));
#25202=CARTESIAN_POINT('Ctrl Pts',(0.711993139340447,-1.,1.64752408828442));
#25203=CARTESIAN_POINT('Ctrl Pts',(0.711993139340447,1.,1.64752408828442));
#25204=CARTESIAN_POINT('Ctrl Pts',(0.705159151977294,-1.,1.6321654166204));
#25205=CARTESIAN_POINT('Ctrl Pts',(0.705159151977294,1.,1.6321654166204));
#25206=CARTESIAN_POINT('Ctrl Pts',(0.699605146398836,-1.,1.61974673471117));
#25207=CARTESIAN_POINT('Ctrl Pts',(0.699605146398836,1.,1.61974673471117));
#25208=CARTESIAN_POINT('Ctrl Pts',(0.69571209787897,-1.,1.61106790957619));
#25209=CARTESIAN_POINT('Ctrl Pts',(0.69571209787897,1.,1.61106790957619));
#25210=CARTESIAN_POINT('Ctrl Pts',(0.693717979106305,-1.,1.60662857109684));
#25211=CARTESIAN_POINT('Ctrl Pts',(0.693717979106305,1.,1.60662857109684));
#25212=CARTESIAN_POINT('',(0.7455743247944,1.,2.0698113262342));
#25213=CARTESIAN_POINT('Ctrl Pts',(0.7455743247944,1.,2.0698113262342));
#25214=CARTESIAN_POINT('Ctrl Pts',(0.745832791378367,1.,2.06854248895728));
#25215=CARTESIAN_POINT('Ctrl Pts',(0.7463458715442,1.,2.06600523016815));
#25216=CARTESIAN_POINT('Ctrl Pts',(0.747103932787919,1.,2.06220058927826));
#25217=CARTESIAN_POINT('Ctrl Pts',(0.748091554183802,1.,2.05713023031007));
#25218=CARTESIAN_POINT('Ctrl Pts',(0.749287468665046,1.,2.05079645592154));
#25219=CARTESIAN_POINT('Ctrl Pts',(0.750444657875575,1.,2.04446689147979));
#25220=CARTESIAN_POINT('Ctrl Pts',(0.751562963361115,1.,2.03814160092099));
#25221=CARTESIAN_POINT('Ctrl Pts',(0.75264218048721,1.,2.03182068456221));
#25222=CARTESIAN_POINT('Ctrl Pts',(0.753682061112768,1.,2.02550428623313));
#25223=CARTESIAN_POINT('Ctrl Pts',(0.754682330722816,1.,2.01919259405809));
#25224=CARTESIAN_POINT('Ctrl Pts',(0.755642704957865,1.,2.01288584328084));
#25225=CARTESIAN_POINT('Ctrl Pts',(0.75656290464667,1.,2.0065843158773));
#25226=CARTESIAN_POINT('Ctrl Pts',(0.757442676862724,1.,2.00028834739178));
#25227=CARTESIAN_POINT('Ctrl Pts',(0.758281796766761,1.,1.99399831098817));
#25228=CARTESIAN_POINT('Ctrl Pts',(0.759080037802488,1.,1.98771456680874));
#25229=CARTESIAN_POINT('Ctrl Pts',(0.75983714745219,1.,1.98143741418172));
#25230=CARTESIAN_POINT('Ctrl Pts',(0.760552825409757,1.,1.97516705321494));
#25231=CARTESIAN_POINT('Ctrl Pts',(0.76122669048382,1.,1.96890351582499));
#25232=CARTESIAN_POINT('Ctrl Pts',(0.761858300014423,1.,1.96264672744186));
#25233=CARTESIAN_POINT('Ctrl Pts',(0.762447203806178,1.,1.95639665309869));
#25234=CARTESIAN_POINT('Ctrl Pts',(0.762992990878769,1.,1.95015342590024));
#25235=CARTESIAN_POINT('Ctrl Pts',(0.763495333538629,1.,1.9439174661764));
#25236=CARTESIAN_POINT('Ctrl Pts',(0.763954049121458,1.,1.93768964875886));
#25237=CARTESIAN_POINT('Ctrl Pts',(0.76436901067394,1.,1.93147105496382));
#25238=CARTESIAN_POINT('Ctrl Pts',(0.764740025488211,1.,1.92526263537048));
#25239=CARTESIAN_POINT('Ctrl Pts',(0.765066729667088,1.,1.91906491634196));
#25240=CARTESIAN_POINT('Ctrl Pts',(0.765348465884722,1.,1.91287765805169));
#25241=CARTESIAN_POINT('Ctrl Pts',(0.765584196937919,1.,1.90669961402356));
#25242=CARTESIAN_POINT('Ctrl Pts',(0.765772772593386,1.,1.90052930393596));
#25243=CARTESIAN_POINT('Ctrl Pts',(0.765913193856978,1.,1.89436577771388));
#25244=CARTESIAN_POINT('Ctrl Pts',(0.766004837062091,1.,1.88820926433409));
#25245=CARTESIAN_POINT('Ctrl Pts',(0.766047794851864,1.,1.88206215302561));
#25246=CARTESIAN_POINT('Ctrl Pts',(0.766042837036744,1.,1.87592888967883));
#25247=CARTESIAN_POINT('Ctrl Pts',(0.765990708546091,1.,1.86981398314341));
#25248=CARTESIAN_POINT('Ctrl Pts',(0.765891519092547,1.,1.86372027063312));
#25249=CARTESIAN_POINT('Ctrl Pts',(0.765744212909318,1.,1.85764741390394));
#25250=CARTESIAN_POINT('Ctrl Pts',(0.765545710619062,1.,1.85158945130063));
#25251=CARTESIAN_POINT('Ctrl Pts',(0.765291664862029,1.,1.84553698875924));
#25252=CARTESIAN_POINT('Ctrl Pts',(0.764978057881737,1.,1.83948181064835));
#25253=CARTESIAN_POINT('Ctrl Pts',(0.764602549687853,1.,1.83342077227142));
#25254=CARTESIAN_POINT('Ctrl Pts',(0.764165902605995,1.,1.82735991200065));
#25255=CARTESIAN_POINT('Ctrl Pts',(0.763673465462726,1.,1.82131873145266));
#25256=CARTESIAN_POINT('Ctrl Pts',(0.763132003836634,1.,1.8153211840553));
#25257=CARTESIAN_POINT('Ctrl Pts',(0.762546129463938,1.,1.80938551463965));
#25258=CARTESIAN_POINT('Ctrl Pts',(0.761915336443547,1.,1.80351583877342));
#25259=CARTESIAN_POINT('Ctrl Pts',(0.761229695230558,1.,1.79768986997783));
#25260=CARTESIAN_POINT('Ctrl Pts',(0.760469555880749,1.,1.7918581561088));
#25261=CARTESIAN_POINT('Ctrl Pts',(0.759614401110189,1.,1.78596964884604));
#25262=CARTESIAN_POINT('Ctrl Pts',(0.758650626677518,1.,1.77999411220945));
#25263=CARTESIAN_POINT('Ctrl Pts',(0.757578264077028,1.,1.77394167108292));
#25264=CARTESIAN_POINT('Ctrl Pts',(0.75642189602781,1.,1.76789396002998));
#25265=CARTESIAN_POINT('Ctrl Pts',(0.755220979974461,1.,1.76197817240128));
#25266=CARTESIAN_POINT('Ctrl Pts',(0.754009254027828,1.,1.75631083600019));
#25267=CARTESIAN_POINT('Ctrl Pts',(0.752797683531314,1.,1.75095139468794));
#25268=CARTESIAN_POINT('Ctrl Pts',(0.751555614164482,1.,1.74585086852502));
#25269=CARTESIAN_POINT('Ctrl Pts',(0.750193435981249,1.,1.74080458267114));
#25270=CARTESIAN_POINT('Ctrl Pts',(0.74858246295687,1.,1.7355035168033));
#25271=CARTESIAN_POINT('Ctrl Pts',(0.746574710097752,1.,1.72958533647714));
#25272=CARTESIAN_POINT('Ctrl Pts',(0.744021445433093,1.,1.72268229916769));
#25273=CARTESIAN_POINT('Ctrl Pts',(0.74079516202821,1.,1.71447789751001));
#25274=CARTESIAN_POINT('Ctrl Pts',(0.736799665716932,1.,1.70473309004249));
#25275=CARTESIAN_POINT('Ctrl Pts',(0.731963238685357,1.,1.69326921972915));
#25276=CARTESIAN_POINT('Ctrl Pts',(0.726235967982445,1.,1.67996158451922));
#25277=CARTESIAN_POINT('Ctrl Pts',(0.719585433787949,1.,1.66472880551777));
#25278=CARTESIAN_POINT('Ctrl Pts',(0.711993139340447,1.,1.64752408828442));
#25279=CARTESIAN_POINT('Ctrl Pts',(0.705159151977294,1.,1.6321654166204));
#25280=CARTESIAN_POINT('Ctrl Pts',(0.699605146398836,1.,1.61974673471117));
#25281=CARTESIAN_POINT('Ctrl Pts',(0.69571209787897,1.,1.61106790957619));
#25282=CARTESIAN_POINT('Ctrl Pts',(0.693717979106305,1.,1.60662857109684));
#25283=CARTESIAN_POINT('',(0.7455743247944,0.,2.0698113262342));
#25284=CARTESIAN_POINT('Origin',(0.61342227326009,0.,2.11275013067528));
#25285=CARTESIAN_POINT('',(0.61342227326009,1.,2.11275013067528));
#25286=CARTESIAN_POINT('',(0.7455743247944,1.,2.0698113262342));
#25287=CARTESIAN_POINT('',(0.61342227326009,0.,2.11275013067528));
#25288=CARTESIAN_POINT('Ctrl Pts',(0.383122945602004,-1.,1.7075470150345));
#25289=CARTESIAN_POINT('Ctrl Pts',(0.383122945602004,1.,1.7075470150345));
#25290=CARTESIAN_POINT('Ctrl Pts',(0.384119047315541,-1.,1.71231062891958));
#25291=CARTESIAN_POINT('Ctrl Pts',(0.384119047315541,1.,1.71231062891958));
#25292=CARTESIAN_POINT('Ctrl Pts',(0.38607079032701,-1.,1.72162022246158));
#25293=CARTESIAN_POINT('Ctrl Pts',(0.38607079032701,1.,1.72162022246158));
#25294=CARTESIAN_POINT('Ctrl Pts',(0.388877023509191,-1.,1.7349317097561));
#25295=CARTESIAN_POINT('Ctrl Pts',(0.388877023509191,1.,1.7349317097561));
#25296=CARTESIAN_POINT('Ctrl Pts',(0.392375812294307,-1.,1.75137405313962));
#25297=CARTESIAN_POINT('Ctrl Pts',(0.392375812294307,1.,1.75137405313962));
#25298=CARTESIAN_POINT('Ctrl Pts',(0.39634619612042,-1.,1.7697556004756));
#25299=CARTESIAN_POINT('Ctrl Pts',(0.39634619612042,1.,1.7697556004756));
#25300=CARTESIAN_POINT('Ctrl Pts',(0.39991940378308,-1.,1.78598826347533));
#25301=CARTESIAN_POINT('Ctrl Pts',(0.39991940378308,1.,1.78598826347533));
#25302=CARTESIAN_POINT('Ctrl Pts',(0.403107976170441,-1.,1.80012077176221));
#25303=CARTESIAN_POINT('Ctrl Pts',(0.403107976170441,1.,1.80012077176221));
#25304=CARTESIAN_POINT('Ctrl Pts',(0.405933518411838,-1.,1.81223801813988));
#25305=CARTESIAN_POINT('Ctrl Pts',(0.405933518411838,1.,1.81223801813988));
#25306=CARTESIAN_POINT('Ctrl Pts',(0.408428948108533,-1.,1.8224702267854));
#25307=CARTESIAN_POINT('Ctrl Pts',(0.408428948108533,1.,1.8224702267854));
#25308=CARTESIAN_POINT('Ctrl Pts',(0.410641256301674,-1.,1.83100408895216));
#25309=CARTESIAN_POINT('Ctrl Pts',(0.410641256301674,1.,1.83100408895216));
#25310=CARTESIAN_POINT('Ctrl Pts',(0.412633125322161,-1.,1.83808953475839));
#25311=CARTESIAN_POINT('Ctrl Pts',(0.412633125322161,1.,1.83808953475839));
#25312=CARTESIAN_POINT('Ctrl Pts',(0.41448743825434,-1.,1.8440575707371));
#25313=CARTESIAN_POINT('Ctrl Pts',(0.41448743825434,1.,1.8440575707371));
#25314=CARTESIAN_POINT('Ctrl Pts',(0.416300022038864,-1.,1.84929312929882));
#25315=CARTESIAN_POINT('Ctrl Pts',(0.416300022038864,1.,1.84929312929882));
#25316=CARTESIAN_POINT('Ctrl Pts',(0.418164129143534,-1.,1.85417632856234));
#25317=CARTESIAN_POINT('Ctrl Pts',(0.418164129143534,1.,1.85417632856234));
#25318=CARTESIAN_POINT('Ctrl Pts',(0.420157287975619,-1.,1.85903281096686));
#25319=CARTESIAN_POINT('Ctrl Pts',(0.420157287975619,1.,1.85903281096686));
#25320=CARTESIAN_POINT('Ctrl Pts',(0.422327307418275,-1.,1.86408083334028));
#25321=CARTESIAN_POINT('Ctrl Pts',(0.422327307418275,1.,1.86408083334028));
#25322=CARTESIAN_POINT('Ctrl Pts',(0.424678177291358,-1.,1.86937803944323));
#25323=CARTESIAN_POINT('Ctrl Pts',(0.424678177291358,1.,1.86937803944323));
#25324=CARTESIAN_POINT('Ctrl Pts',(0.427183828519102,-1.,1.87486989291484));
#25325=CARTESIAN_POINT('Ctrl Pts',(0.427183828519102,1.,1.87486989291484));
#25326=CARTESIAN_POINT('Ctrl Pts',(0.429803062482344,-1.,1.88044229001832));
#25327=CARTESIAN_POINT('Ctrl Pts',(0.429803062482344,1.,1.88044229001832));
#25328=CARTESIAN_POINT('Ctrl Pts',(0.432493038548748,-1.,1.88596913666793));
#25329=CARTESIAN_POINT('Ctrl Pts',(0.432493038548748,1.,1.88596913666793));
#25330=CARTESIAN_POINT('Ctrl Pts',(0.435225660963383,-1.,1.89136993975504));
#25331=CARTESIAN_POINT('Ctrl Pts',(0.435225660963383,1.,1.89136993975504));
#25332=CARTESIAN_POINT('Ctrl Pts',(0.437995003948244,-1.,1.89663648956466));
#25333=CARTESIAN_POINT('Ctrl Pts',(0.437995003948244,1.,1.89663648956466));
#25334=CARTESIAN_POINT('Ctrl Pts',(0.440807833704038,-1.,1.90180124389086));
#25335=CARTESIAN_POINT('Ctrl Pts',(0.440807833704038,1.,1.90180124389086));
#25336=CARTESIAN_POINT('Ctrl Pts',(0.44367755684915,-1.,1.90691756144898));
#25337=CARTESIAN_POINT('Ctrl Pts',(0.44367755684915,1.,1.90691756144898));
#25338=CARTESIAN_POINT('Ctrl Pts',(0.446617343485711,-1.,1.9120369998112));
#25339=CARTESIAN_POINT('Ctrl Pts',(0.446617343485711,1.,1.9120369998112));
#25340=CARTESIAN_POINT('Ctrl Pts',(0.449632260106662,-1.,1.91718342555755));
#25341=CARTESIAN_POINT('Ctrl Pts',(0.449632260106662,1.,1.91718342555755));
#25342=CARTESIAN_POINT('Ctrl Pts',(0.452719478359432,-1.,1.92235380648502));
#25343=CARTESIAN_POINT('Ctrl Pts',(0.452719478359432,1.,1.92235380648502));
#25344=CARTESIAN_POINT('Ctrl Pts',(0.45587200517437,-1.,1.92753067150476));
#25345=CARTESIAN_POINT('Ctrl Pts',(0.45587200517437,1.,1.92753067150476));
#25346=CARTESIAN_POINT('Ctrl Pts',(0.459081234547926,-1.,1.93269066517934));
#25347=CARTESIAN_POINT('Ctrl Pts',(0.459081234547926,1.,1.93269066517934));
#25348=CARTESIAN_POINT('Ctrl Pts',(0.462340031009056,-1.,1.93781486640821));
#25349=CARTESIAN_POINT('Ctrl Pts',(0.462340031009056,1.,1.93781486640821));
#25350=CARTESIAN_POINT('Ctrl Pts',(0.46564546202603,-1.,1.9428979419619));
#25351=CARTESIAN_POINT('Ctrl Pts',(0.46564546202603,1.,1.9428979419619));
#25352=CARTESIAN_POINT('Ctrl Pts',(0.468997482913135,-1.,1.94794381136514));
#25353=CARTESIAN_POINT('Ctrl Pts',(0.468997482913135,1.,1.94794381136514));
#25354=CARTESIAN_POINT('Ctrl Pts',(0.472397672264072,-1.,1.95296148278133));
#25355=CARTESIAN_POINT('Ctrl Pts',(0.472397672264072,1.,1.95296148278133));
#25356=CARTESIAN_POINT('Ctrl Pts',(0.475848034683176,-1.,1.95796111148177));
#25357=CARTESIAN_POINT('Ctrl Pts',(0.475848034683176,1.,1.95796111148177));
#25358=CARTESIAN_POINT('Ctrl Pts',(0.479349583074855,-1.,1.96294933055943));
#25359=CARTESIAN_POINT('Ctrl Pts',(0.479349583074855,1.,1.96294933055943));
#25360=CARTESIAN_POINT('Ctrl Pts',(0.48290166212069,-1.,1.96792703422362));
#25361=CARTESIAN_POINT('Ctrl Pts',(0.48290166212069,1.,1.96792703422362));
#25362=CARTESIAN_POINT('Ctrl Pts',(0.486502692907658,-1.,1.97289186263272));
#25363=CARTESIAN_POINT('Ctrl Pts',(0.486502692907658,1.,1.97289186263272));
#25364=CARTESIAN_POINT('Ctrl Pts',(0.490150627860952,-1.,1.97783973019229));
#25365=CARTESIAN_POINT('Ctrl Pts',(0.490150627860952,1.,1.97783973019229));
#25366=CARTESIAN_POINT('Ctrl Pts',(0.493843476541494,-1.,1.98276658761821));
#25367=CARTESIAN_POINT('Ctrl Pts',(0.493843476541494,1.,1.98276658761821));
#25368=CARTESIAN_POINT('Ctrl Pts',(0.497579909545574,-1.,1.98767044752932));
#25369=CARTESIAN_POINT('Ctrl Pts',(0.497579909545574,1.,1.98767044752932));
#25370=CARTESIAN_POINT('Ctrl Pts',(0.501359287727146,-1.,1.99255149126155));
#25371=CARTESIAN_POINT('Ctrl Pts',(0.501359287727146,1.,1.99255149126155));
#25372=CARTESIAN_POINT('Ctrl Pts',(0.505181361323026,-1.,1.99741107463572));
#25373=CARTESIAN_POINT('Ctrl Pts',(0.505181361323026,1.,1.99741107463572));
#25374=CARTESIAN_POINT('Ctrl Pts',(0.509046069886157,-1.,2.00225107134734));
#25375=CARTESIAN_POINT('Ctrl Pts',(0.509046069886157,1.,2.00225107134734));
#25376=CARTESIAN_POINT('Ctrl Pts',(0.512953306961792,-1.,2.00707309946949));
#25377=CARTESIAN_POINT('Ctrl Pts',(0.512953306961792,1.,2.00707309946949));
#25378=CARTESIAN_POINT('Ctrl Pts',(0.516902681728687,-1.,2.01187773939242));
#25379=CARTESIAN_POINT('Ctrl Pts',(0.516902681728687,1.,2.01187773939242));
#25380=CARTESIAN_POINT('Ctrl Pts',(0.52089359039937,-1.,2.01666477917286));
#25381=CARTESIAN_POINT('Ctrl Pts',(0.52089359039937,1.,2.01666477917286));
#25382=CARTESIAN_POINT('Ctrl Pts',(0.524925318333476,-1.,2.02143356304698));
#25383=CARTESIAN_POINT('Ctrl Pts',(0.524925318333476,1.,2.02143356304698));
#25384=CARTESIAN_POINT('Ctrl Pts',(0.528997127241914,-1.,2.0261832908329));
#25385=CARTESIAN_POINT('Ctrl Pts',(0.528997127241914,1.,2.0261832908329));
#25386=CARTESIAN_POINT('Ctrl Pts',(0.533108355132976,-1.,2.03091336214426));
#25387=CARTESIAN_POINT('Ctrl Pts',(0.533108355132976,1.,2.03091336214426));
#25388=CARTESIAN_POINT('Ctrl Pts',(0.537258489833262,-1.,2.03562362954037));
#25389=CARTESIAN_POINT('Ctrl Pts',(0.537258489833262,1.,2.03562362954037));
#25390=CARTESIAN_POINT('Ctrl Pts',(0.541447120615659,-1.,2.04031422690527));
#25391=CARTESIAN_POINT('Ctrl Pts',(0.541447120615659,1.,2.04031422690527));
#25392=CARTESIAN_POINT('Ctrl Pts',(0.54567390381743,-1.,2.04498544714588));
#25393=CARTESIAN_POINT('Ctrl Pts',(0.54567390381743,1.,2.04498544714588));
#25394=CARTESIAN_POINT('Ctrl Pts',(0.549938525150295,-1.,2.04963761077958));
#25395=CARTESIAN_POINT('Ctrl Pts',(0.549938525150295,1.,2.04963761077958));
#25396=CARTESIAN_POINT('Ctrl Pts',(0.554240657463906,-1.,2.05427091604413));
#25397=CARTESIAN_POINT('Ctrl Pts',(0.554240657463906,1.,2.05427091604413));
#25398=CARTESIAN_POINT('Ctrl Pts',(0.558579940185151,-1.,2.05888537756462));
#25399=CARTESIAN_POINT('Ctrl Pts',(0.558579940185151,1.,2.05888537756462));
#25400=CARTESIAN_POINT('Ctrl Pts',(0.562955993082261,-1.,2.06348090160589));
#25401=CARTESIAN_POINT('Ctrl Pts',(0.562955993082261,1.,2.06348090160589));
#25402=CARTESIAN_POINT('Ctrl Pts',(0.567368421181087,-1.,2.06805732997334));
#25403=CARTESIAN_POINT('Ctrl Pts',(0.567368421181087,1.,2.06805732997334));
#25404=CARTESIAN_POINT('Ctrl Pts',(0.571816823242602,-1.,2.07261449292824));
#25405=CARTESIAN_POINT('Ctrl Pts',(0.571816823242602,1.,2.07261449292824));
#25406=CARTESIAN_POINT('Ctrl Pts',(0.576300797416844,-1.,2.07715226767559));
#25407=CARTESIAN_POINT('Ctrl Pts',(0.576300797416844,1.,2.07715226767559));
#25408=CARTESIAN_POINT('Ctrl Pts',(0.580819952108063,-1.,2.08167059018418));
#25409=CARTESIAN_POINT('Ctrl Pts',(0.580819952108063,1.,2.08167059018418));
#25410=CARTESIAN_POINT('Ctrl Pts',(0.585373918991617,-1.,2.08616943727951));
#25411=CARTESIAN_POINT('Ctrl Pts',(0.585373918991617,1.,2.08616943727951));
#25412=CARTESIAN_POINT('Ctrl Pts',(0.589962365403406,-1.,2.09064881812129));
#25413=CARTESIAN_POINT('Ctrl Pts',(0.589962365403406,1.,2.09064881812129));
#25414=CARTESIAN_POINT('Ctrl Pts',(0.594585006052162,-1.,2.0951087622027));
#25415=CARTESIAN_POINT('Ctrl Pts',(0.594585006052162,1.,2.0951087622027));
#25416=CARTESIAN_POINT('Ctrl Pts',(0.599241616420533,-1.,2.0995493086477));
#25417=CARTESIAN_POINT('Ctrl Pts',(0.599241616420533,1.,2.0995493086477));
#25418=CARTESIAN_POINT('Ctrl Pts',(0.60393203073603,-1.,2.10397049886949));
#25419=CARTESIAN_POINT('Ctrl Pts',(0.60393203073603,1.,2.10397049886949));
#25420=CARTESIAN_POINT('Ctrl Pts',(0.607711315454876,-1.,2.1074919961518));
#25421=CARTESIAN_POINT('Ctrl Pts',(0.607711315454876,1.,2.1074919961518));
#25422=CARTESIAN_POINT('Ctrl Pts',(0.610560911689898,-1.,2.11012443807238));
#25423=CARTESIAN_POINT('Ctrl Pts',(0.610560911689898,1.,2.11012443807238));
#25424=CARTESIAN_POINT('Ctrl Pts',(0.6124673655618,-1.,2.11187554259986));
#25425=CARTESIAN_POINT('Ctrl Pts',(0.6124673655618,1.,2.11187554259986));
#25426=CARTESIAN_POINT('Ctrl Pts',(0.61342227326009,-1.,2.11275013067528));
#25427=CARTESIAN_POINT('Ctrl Pts',(0.61342227326009,1.,2.11275013067528));
#25428=CARTESIAN_POINT('',(0.383122945602004,1.,1.7075470150345));
#25429=CARTESIAN_POINT('Ctrl Pts',(0.383122945602004,1.,1.7075470150345));
#25430=CARTESIAN_POINT('Ctrl Pts',(0.384119047315541,1.,1.71231062891958));
#25431=CARTESIAN_POINT('Ctrl Pts',(0.38607079032701,1.,1.72162022246158));
#25432=CARTESIAN_POINT('Ctrl Pts',(0.388877023509191,1.,1.7349317097561));
#25433=CARTESIAN_POINT('Ctrl Pts',(0.392375812294307,1.,1.75137405313962));
#25434=CARTESIAN_POINT('Ctrl Pts',(0.39634619612042,1.,1.7697556004756));
#25435=CARTESIAN_POINT('Ctrl Pts',(0.39991940378308,1.,1.78598826347533));
#25436=CARTESIAN_POINT('Ctrl Pts',(0.403107976170441,1.,1.80012077176221));
#25437=CARTESIAN_POINT('Ctrl Pts',(0.405933518411838,1.,1.81223801813988));
#25438=CARTESIAN_POINT('Ctrl Pts',(0.408428948108533,1.,1.8224702267854));
#25439=CARTESIAN_POINT('Ctrl Pts',(0.410641256301674,1.,1.83100408895216));
#25440=CARTESIAN_POINT('Ctrl Pts',(0.412633125322161,1.,1.83808953475839));
#25441=CARTESIAN_POINT('Ctrl Pts',(0.41448743825434,1.,1.8440575707371));
#25442=CARTESIAN_POINT('Ctrl Pts',(0.416300022038864,1.,1.84929312929882));
#25443=CARTESIAN_POINT('Ctrl Pts',(0.418164129143534,1.,1.85417632856234));
#25444=CARTESIAN_POINT('Ctrl Pts',(0.420157287975619,1.,1.85903281096686));
#25445=CARTESIAN_POINT('Ctrl Pts',(0.422327307418275,1.,1.86408083334028));
#25446=CARTESIAN_POINT('Ctrl Pts',(0.424678177291358,1.,1.86937803944323));
#25447=CARTESIAN_POINT('Ctrl Pts',(0.427183828519102,1.,1.87486989291484));
#25448=CARTESIAN_POINT('Ctrl Pts',(0.429803062482344,1.,1.88044229001832));
#25449=CARTESIAN_POINT('Ctrl Pts',(0.432493038548748,1.,1.88596913666793));
#25450=CARTESIAN_POINT('Ctrl Pts',(0.435225660963383,1.,1.89136993975504));
#25451=CARTESIAN_POINT('Ctrl Pts',(0.437995003948244,1.,1.89663648956466));
#25452=CARTESIAN_POINT('Ctrl Pts',(0.440807833704038,1.,1.90180124389086));
#25453=CARTESIAN_POINT('Ctrl Pts',(0.44367755684915,1.,1.90691756144898));
#25454=CARTESIAN_POINT('Ctrl Pts',(0.446617343485711,1.,1.9120369998112));
#25455=CARTESIAN_POINT('Ctrl Pts',(0.449632260106662,1.,1.91718342555755));
#25456=CARTESIAN_POINT('Ctrl Pts',(0.452719478359432,1.,1.92235380648502));
#25457=CARTESIAN_POINT('Ctrl Pts',(0.45587200517437,1.,1.92753067150476));
#25458=CARTESIAN_POINT('Ctrl Pts',(0.459081234547926,1.,1.93269066517934));
#25459=CARTESIAN_POINT('Ctrl Pts',(0.462340031009056,1.,1.93781486640821));
#25460=CARTESIAN_POINT('Ctrl Pts',(0.46564546202603,1.,1.9428979419619));
#25461=CARTESIAN_POINT('Ctrl Pts',(0.468997482913135,1.,1.94794381136514));
#25462=CARTESIAN_POINT('Ctrl Pts',(0.472397672264072,1.,1.95296148278133));
#25463=CARTESIAN_POINT('Ctrl Pts',(0.475848034683176,1.,1.95796111148177));
#25464=CARTESIAN_POINT('Ctrl Pts',(0.479349583074855,1.,1.96294933055943));
#25465=CARTESIAN_POINT('Ctrl Pts',(0.48290166212069,1.,1.96792703422362));
#25466=CARTESIAN_POINT('Ctrl Pts',(0.486502692907658,1.,1.97289186263272));
#25467=CARTESIAN_POINT('Ctrl Pts',(0.490150627860952,1.,1.97783973019229));
#25468=CARTESIAN_POINT('Ctrl Pts',(0.493843476541494,1.,1.98276658761821));
#25469=CARTESIAN_POINT('Ctrl Pts',(0.497579909545574,1.,1.98767044752932));
#25470=CARTESIAN_POINT('Ctrl Pts',(0.501359287727146,1.,1.99255149126155));
#25471=CARTESIAN_POINT('Ctrl Pts',(0.505181361323026,1.,1.99741107463572));
#25472=CARTESIAN_POINT('Ctrl Pts',(0.509046069886157,1.,2.00225107134734));
#25473=CARTESIAN_POINT('Ctrl Pts',(0.512953306961792,1.,2.00707309946949));
#25474=CARTESIAN_POINT('Ctrl Pts',(0.516902681728687,1.,2.01187773939242));
#25475=CARTESIAN_POINT('Ctrl Pts',(0.52089359039937,1.,2.01666477917286));
#25476=CARTESIAN_POINT('Ctrl Pts',(0.524925318333476,1.,2.02143356304698));
#25477=CARTESIAN_POINT('Ctrl Pts',(0.528997127241914,1.,2.0261832908329));
#25478=CARTESIAN_POINT('Ctrl Pts',(0.533108355132976,1.,2.03091336214426));
#25479=CARTESIAN_POINT('Ctrl Pts',(0.537258489833262,1.,2.03562362954037));
#25480=CARTESIAN_POINT('Ctrl Pts',(0.541447120615659,1.,2.04031422690527));
#25481=CARTESIAN_POINT('Ctrl Pts',(0.54567390381743,1.,2.04498544714588));
#25482=CARTESIAN_POINT('Ctrl Pts',(0.549938525150295,1.,2.04963761077958));
#25483=CARTESIAN_POINT('Ctrl Pts',(0.554240657463906,1.,2.05427091604413));
#25484=CARTESIAN_POINT('Ctrl Pts',(0.558579940185151,1.,2.05888537756462));
#25485=CARTESIAN_POINT('Ctrl Pts',(0.562955993082261,1.,2.06348090160589));
#25486=CARTESIAN_POINT('Ctrl Pts',(0.567368421181087,1.,2.06805732997334));
#25487=CARTESIAN_POINT('Ctrl Pts',(0.571816823242602,1.,2.07261449292824));
#25488=CARTESIAN_POINT('Ctrl Pts',(0.576300797416844,1.,2.07715226767559));
#25489=CARTESIAN_POINT('Ctrl Pts',(0.580819952108063,1.,2.08167059018418));
#25490=CARTESIAN_POINT('Ctrl Pts',(0.585373918991617,1.,2.08616943727951));
#25491=CARTESIAN_POINT('Ctrl Pts',(0.589962365403406,1.,2.09064881812129));
#25492=CARTESIAN_POINT('Ctrl Pts',(0.594585006052162,1.,2.0951087622027));
#25493=CARTESIAN_POINT('Ctrl Pts',(0.599241616420533,1.,2.0995493086477));
#25494=CARTESIAN_POINT('Ctrl Pts',(0.60393203073603,1.,2.10397049886949));
#25495=CARTESIAN_POINT('Ctrl Pts',(0.607711315454876,1.,2.1074919961518));
#25496=CARTESIAN_POINT('Ctrl Pts',(0.610560911689898,1.,2.11012443807238));
#25497=CARTESIAN_POINT('Ctrl Pts',(0.6124673655618,1.,2.11187554259986));
#25498=CARTESIAN_POINT('Ctrl Pts',(0.61342227326009,1.,2.11275013067528));
#25499=CARTESIAN_POINT('',(0.383122945602003,0.,1.7075470150345));
#25500=CARTESIAN_POINT('Origin',(0.,0.,0.));
#25501=CARTESIAN_POINT('',(0.163289472382896,1.,1.74236521665491));
#25502=CARTESIAN_POINT('Origin',(0.,1.,0.));
#25503=CARTESIAN_POINT('',(0.163289472382896,0.,1.74236521665491));
#25504=CARTESIAN_POINT('Ctrl Pts',(0.0694764450219578,-1.,2.19890268624765));
#25505=CARTESIAN_POINT('Ctrl Pts',(0.0694764450219578,1.,2.19890268624765));
#25506=CARTESIAN_POINT('Ctrl Pts',(0.0701143536325487,-1.,2.19777582085423));
#25507=CARTESIAN_POINT('Ctrl Pts',(0.0701143536325487,1.,2.19777582085423));
#25508=CARTESIAN_POINT('Ctrl Pts',(0.0713863779526151,-1.,2.19552129484002));
#25509=CARTESIAN_POINT('Ctrl Pts',(0.0713863779526151,1.,2.19552129484002));
#25510=CARTESIAN_POINT('Ctrl Pts',(0.0732830357306722,-1.,2.19213712013662));
#25511=CARTESIAN_POINT('Ctrl Pts',(0.0732830357306722,1.,2.19213712013662));
#25512=CARTESIAN_POINT('Ctrl Pts',(0.0757891465836145,-1.,2.1876201139953));
#25513=CARTESIAN_POINT('Ctrl Pts',(0.0757891465836145,1.,2.1876201139953));
#25514=CARTESIAN_POINT('Ctrl Pts',(0.078883772768524,-1.,2.18196589448887));
#25515=CARTESIAN_POINT('Ctrl Pts',(0.078883772768524,1.,2.18196589448887));
#25516=CARTESIAN_POINT('Ctrl Pts',(0.0819402680872763,-1.,2.176303712113));
#25517=CARTESIAN_POINT('Ctrl Pts',(0.0819402680872763,1.,2.176303712113));
#25518=CARTESIAN_POINT('Ctrl Pts',(0.084958462083537,-1.,2.17063357870952));
#25519=CARTESIAN_POINT('Ctrl Pts',(0.084958462083537,1.,2.17063357870952));
#25520=CARTESIAN_POINT('Ctrl Pts',(0.087938129138692,-1.,2.16495552645014));
#25521=CARTESIAN_POINT('Ctrl Pts',(0.087938129138692,1.,2.16495552645014));
#25522=CARTESIAN_POINT('Ctrl Pts',(0.0908789888107263,-1.,2.15926961544516));
#25523=CARTESIAN_POINT('Ctrl Pts',(0.0908789888107263,1.,2.15926961544516));
#25524=CARTESIAN_POINT('Ctrl Pts',(0.0937807218867641,-1.,2.1535759397817));
#25525=CARTESIAN_POINT('Ctrl Pts',(0.0937807218867641,1.,2.1535759397817));
#25526=CARTESIAN_POINT('Ctrl Pts',(0.0966429852305456,-1.,2.14787463531795));
#25527=CARTESIAN_POINT('Ctrl Pts',(0.0966429852305456,1.,2.14787463531795));
#25528=CARTESIAN_POINT('Ctrl Pts',(0.0994654261990913,-1.,2.14216588396025));
#25529=CARTESIAN_POINT('Ctrl Pts',(0.0994654261990913,1.,2.14216588396025));
#25530=CARTESIAN_POINT('Ctrl Pts',(0.1022477005561,-1.,2.13644992667165));
#25531=CARTESIAN_POINT('Ctrl Pts',(0.1022477005561,1.,2.13644992667165));
#25532=CARTESIAN_POINT('Ctrl Pts',(0.104989479152739,-1.,2.13072704887293));
#25533=CARTESIAN_POINT('Ctrl Pts',(0.104989479152739,1.,2.13072704887293));
#25534=CARTESIAN_POINT('Ctrl Pts',(0.10769043523109,-1.,2.12499752307));
#25535=CARTESIAN_POINT('Ctrl Pts',(0.10769043523109,1.,2.12499752307));
#25536=CARTESIAN_POINT('Ctrl Pts',(0.110350236135025,-1.,2.11926155590865));
#25537=CARTESIAN_POINT('Ctrl Pts',(0.110350236135025,1.,2.11926155590865));
#25538=CARTESIAN_POINT('Ctrl Pts',(0.112968534419737,-1.,2.11351924490306));
#25539=CARTESIAN_POINT('Ctrl Pts',(0.112968534419737,1.,2.11351924490306));
#25540=CARTESIAN_POINT('Ctrl Pts',(0.115544957687926,-1.,2.10777050261309));
#25541=CARTESIAN_POINT('Ctrl Pts',(0.115544957687926,1.,2.10777050261309));
#25542=CARTESIAN_POINT('Ctrl Pts',(0.118079107988355,-1.,2.102015121329));
#25543=CARTESIAN_POINT('Ctrl Pts',(0.118079107988355,1.,2.102015121329));
#25544=CARTESIAN_POINT('Ctrl Pts',(0.120570567965122,-1.,2.0962529286773));
#25545=CARTESIAN_POINT('Ctrl Pts',(0.120570567965122,1.,2.0962529286773));
#25546=CARTESIAN_POINT('Ctrl Pts',(0.123018905621083,-1.,2.09048392424825));
#25547=CARTESIAN_POINT('Ctrl Pts',(0.123018905621083,1.,2.09048392424825));
#25548=CARTESIAN_POINT('Ctrl Pts',(0.125423679412061,-1.,2.08470840653643));
#25549=CARTESIAN_POINT('Ctrl Pts',(0.125423679412061,1.,2.08470840653643));
#25550=CARTESIAN_POINT('Ctrl Pts',(0.12778444527612,-1.,2.07892715110987));
#25551=CARTESIAN_POINT('Ctrl Pts',(0.12778444527612,1.,2.07892715110987));
#25552=CARTESIAN_POINT('Ctrl Pts',(0.130100748328403,-1.,2.07314114713063));
#25553=CARTESIAN_POINT('Ctrl Pts',(0.130100748328403,1.,2.07314114713063));
#25554=CARTESIAN_POINT('Ctrl Pts',(0.13237211154771,-1.,2.06735123910326));
#25555=CARTESIAN_POINT('Ctrl Pts',(0.13237211154771,1.,2.06735123910326));
#25556=CARTESIAN_POINT('Ctrl Pts',(0.134598026192106,-1.,2.06155781517842));
#25557=CARTESIAN_POINT('Ctrl Pts',(0.134598026192106,1.,2.06155781517842));
#25558=CARTESIAN_POINT('Ctrl Pts',(0.136777941218043,-1.,2.05576044414264));
#25559=CARTESIAN_POINT('Ctrl Pts',(0.136777941218043,1.,2.05576044414264));
#25560=CARTESIAN_POINT('Ctrl Pts',(0.138911255368966,-1.,2.04995762001328));
#25561=CARTESIAN_POINT('Ctrl Pts',(0.138911255368966,1.,2.04995762001328));
#25562=CARTESIAN_POINT('Ctrl Pts',(0.140997332152546,-1.,2.04414757947916));
#25563=CARTESIAN_POINT('Ctrl Pts',(0.140997332152546,1.,2.04414757947916));
#25564=CARTESIAN_POINT('Ctrl Pts',(0.143035515058208,-1.,2.03832911025912));
#25565=CARTESIAN_POINT('Ctrl Pts',(0.143035515058208,1.,2.03832911025912));
#25566=CARTESIAN_POINT('Ctrl Pts',(0.145025140186057,-1.,2.03250223739942));
#25567=CARTESIAN_POINT('Ctrl Pts',(0.145025140186057,1.,2.03250223739942));
#25568=CARTESIAN_POINT('Ctrl Pts',(0.146965557332583,-1.,2.02666926182017));
#25569=CARTESIAN_POINT('Ctrl Pts',(0.146965557332583,1.,2.02666926182017));
#25570=CARTESIAN_POINT('Ctrl Pts',(0.148856124775337,-1.,2.02083464969894));
#25571=CARTESIAN_POINT('Ctrl Pts',(0.148856124775337,1.,2.02083464969894));
#25572=CARTESIAN_POINT('Ctrl Pts',(0.150696157673078,-1.,2.01500291940238));
#25573=CARTESIAN_POINT('Ctrl Pts',(0.150696157673078,1.,2.01500291940238));
#25574=CARTESIAN_POINT('Ctrl Pts',(0.152484883621449,-1.,2.00917680318424));
#25575=CARTESIAN_POINT('Ctrl Pts',(0.152484883621449,1.,2.00917680318424));
#25576=CARTESIAN_POINT('Ctrl Pts',(0.154221403049722,-1.,2.00335565310543));
#25577=CARTESIAN_POINT('Ctrl Pts',(0.154221403049722,1.,2.00335565310543));
#25578=CARTESIAN_POINT('Ctrl Pts',(0.155904629548783,-1.,1.99753284771497));
#25579=CARTESIAN_POINT('Ctrl Pts',(0.155904629548783,1.,1.99753284771497));
#25580=CARTESIAN_POINT('Ctrl Pts',(0.157533331459227,-1.,1.99169810931908));
#25581=CARTESIAN_POINT('Ctrl Pts',(0.157533331459227,1.,1.99169810931908));
#25582=CARTESIAN_POINT('Ctrl Pts',(0.159106226437299,-1.,1.98584238283292));
#25583=CARTESIAN_POINT('Ctrl Pts',(0.159106226437299,1.,1.98584238283292));
#25584=CARTESIAN_POINT('Ctrl Pts',(0.160622060784611,-1.,1.97996195437559));
#25585=CARTESIAN_POINT('Ctrl Pts',(0.160622060784611,1.,1.97996195437559));
#25586=CARTESIAN_POINT('Ctrl Pts',(0.162079693556288,-1.,1.97406280235188));
#25587=CARTESIAN_POINT('Ctrl Pts',(0.162079693556288,1.,1.97406280235188));
#25588=CARTESIAN_POINT('Ctrl Pts',(0.163478185457734,-1.,1.96816512677967));
#25589=CARTESIAN_POINT('Ctrl Pts',(0.163478185457734,1.,1.96816512677967));
#25590=CARTESIAN_POINT('Ctrl Pts',(0.164816568920269,-1.,1.96229379940136));
#25591=CARTESIAN_POINT('Ctrl Pts',(0.164816568920269,1.,1.96229379940136));
#25592=CARTESIAN_POINT('Ctrl Pts',(0.166093592002812,-1.,1.9564675971873));
#25593=CARTESIAN_POINT('Ctrl Pts',(0.166093592002812,1.,1.9564675971873));
#25594=CARTESIAN_POINT('Ctrl Pts',(0.167307501784475,-1.,1.95069027794294));
#25595=CARTESIAN_POINT('Ctrl Pts',(0.167307501784475,1.,1.95069027794294));
#25596=CARTESIAN_POINT('Ctrl Pts',(0.168455741607556,-1.,1.94493757756931));
#25597=CARTESIAN_POINT('Ctrl Pts',(0.168455741607556,1.,1.94493757756931));
#25598=CARTESIAN_POINT('Ctrl Pts',(0.16953490481749,-1.,1.93915639211581));
#25599=CARTESIAN_POINT('Ctrl Pts',(0.16953490481749,1.,1.93915639211581));
#25600=CARTESIAN_POINT('Ctrl Pts',(0.170541253116201,-1.,1.93329183155539));
#25601=CARTESIAN_POINT('Ctrl Pts',(0.170541253116201,1.,1.93329183155539));
#25602=CARTESIAN_POINT('Ctrl Pts',(0.171471191532988,-1.,1.92731093582036));
#25603=CARTESIAN_POINT('Ctrl Pts',(0.171471191532988,1.,1.92731093582036));
#25604=CARTESIAN_POINT('Ctrl Pts',(0.172321621259513,-1.,1.9212233439798));
#25605=CARTESIAN_POINT('Ctrl Pts',(0.172321621259513,1.,1.9212233439798));
#25606=CARTESIAN_POINT('Ctrl Pts',(0.173090695383496,-1.,1.91511429159527));
#25607=CARTESIAN_POINT('Ctrl Pts',(0.173090695383496,1.,1.91511429159527));
#25608=CARTESIAN_POINT('Ctrl Pts',(0.173776635257816,-1.,1.90911693975267));
#25609=CARTESIAN_POINT('Ctrl Pts',(0.173776635257816,1.,1.90911693975267));
#25610=CARTESIAN_POINT('Ctrl Pts',(0.174375518661085,-1.,1.90335253862834));
#25611=CARTESIAN_POINT('Ctrl Pts',(0.174375518661085,1.,1.90335253862834));
#25612=CARTESIAN_POINT('Ctrl Pts',(0.174879405091263,-1.,1.89788101117132));
#25613=CARTESIAN_POINT('Ctrl Pts',(0.174879405091263,1.,1.89788101117132));
#25614=CARTESIAN_POINT('Ctrl Pts',(0.175274276190844,-1.,1.892646301985));
#25615=CARTESIAN_POINT('Ctrl Pts',(0.175274276190844,1.,1.892646301985));
#25616=CARTESIAN_POINT('Ctrl Pts',(0.175538155840648,-1.,1.88742606273259));
#25617=CARTESIAN_POINT('Ctrl Pts',(0.175538155840648,1.,1.88742606273259));
#25618=CARTESIAN_POINT('Ctrl Pts',(0.175644148889698,-1.,1.88188663145367));
#25619=CARTESIAN_POINT('Ctrl Pts',(0.175644148889698,1.,1.88188663145367));
#25620=CARTESIAN_POINT('Ctrl Pts',(0.175563480746485,-1.,1.87563767773588));
#25621=CARTESIAN_POINT('Ctrl Pts',(0.175563480746485,1.,1.87563767773588));
#25622=CARTESIAN_POINT('Ctrl Pts',(0.175268337590757,-1.,1.86828349694799));
#25623=CARTESIAN_POINT('Ctrl Pts',(0.175268337590757,1.,1.86828349694799));
#25624=CARTESIAN_POINT('Ctrl Pts',(0.17473525927603,-1.,1.85948367088837));
#25625=CARTESIAN_POINT('Ctrl Pts',(0.17473525927603,1.,1.85948367088837));
#25626=CARTESIAN_POINT('Ctrl Pts',(0.173946627587731,-1.,1.8489811319852));
#25627=CARTESIAN_POINT('Ctrl Pts',(0.173946627587731,1.,1.8489811319852));
#25628=CARTESIAN_POINT('Ctrl Pts',(0.1728894428919,-1.,1.83658380527692));
#25629=CARTESIAN_POINT('Ctrl Pts',(0.1728894428919,1.,1.83658380527692));
#25630=CARTESIAN_POINT('Ctrl Pts',(0.171554770204119,-1.,1.82215766811545));
#25631=CARTESIAN_POINT('Ctrl Pts',(0.171554770204119,1.,1.82215766811545));
#25632=CARTESIAN_POINT('Ctrl Pts',(0.169936923904608,-1.,1.80561530629706));
#25633=CARTESIAN_POINT('Ctrl Pts',(0.169936923904608,1.,1.80561530629706));
#25634=CARTESIAN_POINT('Ctrl Pts',(0.168032772805197,-1.,1.7869064998507));
#25635=CARTESIAN_POINT('Ctrl Pts',(0.168032772805197,1.,1.7869064998507));
#25636=CARTESIAN_POINT('Ctrl Pts',(0.1662793551464,-1.,1.77018771684844));
#25637=CARTESIAN_POINT('Ctrl Pts',(0.1662793551464,1.,1.77018771684844));
#25638=CARTESIAN_POINT('Ctrl Pts',(0.164834765707158,-1.,1.75666056638427));
#25639=CARTESIAN_POINT('Ctrl Pts',(0.164834765707158,1.,1.75666056638427));
#25640=CARTESIAN_POINT('Ctrl Pts',(0.163814161002002,-1.,1.7472034950333));
#25641=CARTESIAN_POINT('Ctrl Pts',(0.163814161002002,1.,1.7472034950333));
#25642=CARTESIAN_POINT('Ctrl Pts',(0.163289472382896,-1.,1.74236521665491));
#25643=CARTESIAN_POINT('Ctrl Pts',(0.163289472382896,1.,1.74236521665491));
#25644=CARTESIAN_POINT('',(0.0694764450219578,1.,2.19890268624765));
#25645=CARTESIAN_POINT('Ctrl Pts',(0.0694764450219578,1.,2.19890268624765));
#25646=CARTESIAN_POINT('Ctrl Pts',(0.0701143536325487,1.,2.19777582085423));
#25647=CARTESIAN_POINT('Ctrl Pts',(0.0713863779526151,1.,2.19552129484002));
#25648=CARTESIAN_POINT('Ctrl Pts',(0.0732830357306722,1.,2.19213712013662));
#25649=CARTESIAN_POINT('Ctrl Pts',(0.0757891465836145,1.,2.1876201139953));
#25650=CARTESIAN_POINT('Ctrl Pts',(0.078883772768524,1.,2.18196589448887));
#25651=CARTESIAN_POINT('Ctrl Pts',(0.0819402680872763,1.,2.176303712113));
#25652=CARTESIAN_POINT('Ctrl Pts',(0.084958462083537,1.,2.17063357870952));
#25653=CARTESIAN_POINT('Ctrl Pts',(0.087938129138692,1.,2.16495552645014));
#25654=CARTESIAN_POINT('Ctrl Pts',(0.0908789888107263,1.,2.15926961544516));
#25655=CARTESIAN_POINT('Ctrl Pts',(0.0937807218867641,1.,2.1535759397817));
#25656=CARTESIAN_POINT('Ctrl Pts',(0.0966429852305456,1.,2.14787463531795));
#25657=CARTESIAN_POINT('Ctrl Pts',(0.0994654261990913,1.,2.14216588396025));
#25658=CARTESIAN_POINT('Ctrl Pts',(0.1022477005561,1.,2.13644992667165));
#25659=CARTESIAN_POINT('Ctrl Pts',(0.104989479152739,1.,2.13072704887293));
#25660=CARTESIAN_POINT('Ctrl Pts',(0.10769043523109,1.,2.12499752307));
#25661=CARTESIAN_POINT('Ctrl Pts',(0.110350236135025,1.,2.11926155590865));
#25662=CARTESIAN_POINT('Ctrl Pts',(0.112968534419737,1.,2.11351924490306));
#25663=CARTESIAN_POINT('Ctrl Pts',(0.115544957687926,1.,2.10777050261309));
#25664=CARTESIAN_POINT('Ctrl Pts',(0.118079107988355,1.,2.102015121329));
#25665=CARTESIAN_POINT('Ctrl Pts',(0.120570567965122,1.,2.0962529286773));
#25666=CARTESIAN_POINT('Ctrl Pts',(0.123018905621083,1.,2.09048392424825));
#25667=CARTESIAN_POINT('Ctrl Pts',(0.125423679412061,1.,2.08470840653643));
#25668=CARTESIAN_POINT('Ctrl Pts',(0.12778444527612,1.,2.07892715110987));
#25669=CARTESIAN_POINT('Ctrl Pts',(0.130100748328403,1.,2.07314114713063));
#25670=CARTESIAN_POINT('Ctrl Pts',(0.13237211154771,1.,2.06735123910326));
#25671=CARTESIAN_POINT('Ctrl Pts',(0.134598026192106,1.,2.06155781517842));
#25672=CARTESIAN_POINT('Ctrl Pts',(0.136777941218043,1.,2.05576044414264));
#25673=CARTESIAN_POINT('Ctrl Pts',(0.138911255368966,1.,2.04995762001328));
#25674=CARTESIAN_POINT('Ctrl Pts',(0.140997332152546,1.,2.04414757947916));
#25675=CARTESIAN_POINT('Ctrl Pts',(0.143035515058208,1.,2.03832911025912));
#25676=CARTESIAN_POINT('Ctrl Pts',(0.145025140186057,1.,2.03250223739942));
#25677=CARTESIAN_POINT('Ctrl Pts',(0.146965557332583,1.,2.02666926182017));
#25678=CARTESIAN_POINT('Ctrl Pts',(0.148856124775337,1.,2.02083464969894));
#25679=CARTESIAN_POINT('Ctrl Pts',(0.150696157673078,1.,2.01500291940238));
#25680=CARTESIAN_POINT('Ctrl Pts',(0.152484883621449,1.,2.00917680318424));
#25681=CARTESIAN_POINT('Ctrl Pts',(0.154221403049722,1.,2.00335565310543));
#25682=CARTESIAN_POINT('Ctrl Pts',(0.155904629548783,1.,1.99753284771497));
#25683=CARTESIAN_POINT('Ctrl Pts',(0.157533331459227,1.,1.99169810931908));
#25684=CARTESIAN_POINT('Ctrl Pts',(0.159106226437299,1.,1.98584238283292));
#25685=CARTESIAN_POINT('Ctrl Pts',(0.160622060784611,1.,1.97996195437559));
#25686=CARTESIAN_POINT('Ctrl Pts',(0.162079693556288,1.,1.97406280235188));
#25687=CARTESIAN_POINT('Ctrl Pts',(0.163478185457734,1.,1.96816512677967));
#25688=CARTESIAN_POINT('Ctrl Pts',(0.164816568920269,1.,1.96229379940136));
#25689=CARTESIAN_POINT('Ctrl Pts',(0.166093592002812,1.,1.9564675971873));
#25690=CARTESIAN_POINT('Ctrl Pts',(0.167307501784475,1.,1.95069027794294));
#25691=CARTESIAN_POINT('Ctrl Pts',(0.168455741607556,1.,1.94493757756931));
#25692=CARTESIAN_POINT('Ctrl Pts',(0.16953490481749,1.,1.93915639211581));
#25693=CARTESIAN_POINT('Ctrl Pts',(0.170541253116201,1.,1.93329183155539));
#25694=CARTESIAN_POINT('Ctrl Pts',(0.171471191532988,1.,1.92731093582036));
#25695=CARTESIAN_POINT('Ctrl Pts',(0.172321621259513,1.,1.9212233439798));
#25696=CARTESIAN_POINT('Ctrl Pts',(0.173090695383496,1.,1.91511429159527));
#25697=CARTESIAN_POINT('Ctrl Pts',(0.173776635257816,1.,1.90911693975267));
#25698=CARTESIAN_POINT('Ctrl Pts',(0.174375518661085,1.,1.90335253862834));
#25699=CARTESIAN_POINT('Ctrl Pts',(0.174879405091263,1.,1.89788101117132));
#25700=CARTESIAN_POINT('Ctrl Pts',(0.175274276190844,1.,1.892646301985));
#25701=CARTESIAN_POINT('Ctrl Pts',(0.175538155840648,1.,1.88742606273259));
#25702=CARTESIAN_POINT('Ctrl Pts',(0.175644148889698,1.,1.88188663145367));
#25703=CARTESIAN_POINT('Ctrl Pts',(0.175563480746485,1.,1.87563767773588));
#25704=CARTESIAN_POINT('Ctrl Pts',(0.175268337590757,1.,1.86828349694799));
#25705=CARTESIAN_POINT('Ctrl Pts',(0.17473525927603,1.,1.85948367088837));
#25706=CARTESIAN_POINT('Ctrl Pts',(0.173946627587731,1.,1.8489811319852));
#25707=CARTESIAN_POINT('Ctrl Pts',(0.1728894428919,1.,1.83658380527692));
#25708=CARTESIAN_POINT('Ctrl Pts',(0.171554770204119,1.,1.82215766811545));
#25709=CARTESIAN_POINT('Ctrl Pts',(0.169936923904608,1.,1.80561530629706));
#25710=CARTESIAN_POINT('Ctrl Pts',(0.168032772805197,1.,1.7869064998507));
#25711=CARTESIAN_POINT('Ctrl Pts',(0.1662793551464,1.,1.77018771684844));
#25712=CARTESIAN_POINT('Ctrl Pts',(0.164834765707158,1.,1.75666056638427));
#25713=CARTESIAN_POINT('Ctrl Pts',(0.163814161002002,1.,1.7472034950333));
#25714=CARTESIAN_POINT('Ctrl Pts',(0.163289472382896,1.,1.74236521665491));
#25715=CARTESIAN_POINT('',(0.0694764450219578,0.,2.19890268624765));
#25716=CARTESIAN_POINT('Origin',(-0.0694764450219586,0.,2.19890268624765));
#25717=CARTESIAN_POINT('',(-0.0694764450219586,1.,2.19890268624765));
#25718=CARTESIAN_POINT('',(0.0694764450219578,1.,2.19890268624765));
#25719=CARTESIAN_POINT('',(-0.0694764450219586,0.,2.19890268624765));
#25720=CARTESIAN_POINT('Ctrl Pts',(-0.163289472382896,-1.,1.74236521665491));
#25721=CARTESIAN_POINT('Ctrl Pts',(-0.163289472382896,1.,1.74236521665491));
#25722=CARTESIAN_POINT('Ctrl Pts',(-0.163814161002474,-1.,1.74720349503904));
#25723=CARTESIAN_POINT('Ctrl Pts',(-0.163814161002474,1.,1.74720349503904));
#25724=CARTESIAN_POINT('Ctrl Pts',(-0.164834765708484,-1.,1.75666056640041));
#25725=CARTESIAN_POINT('Ctrl Pts',(-0.164834765708484,1.,1.75666056640041));
#25726=CARTESIAN_POINT('Ctrl Pts',(-0.166279355148738,-1.,1.77018771687692));
#25727=CARTESIAN_POINT('Ctrl Pts',(-0.166279355148738,1.,1.77018771687692));
#25728=CARTESIAN_POINT('Ctrl Pts',(-0.16803277280837,-1.,1.78690649988931));
#25729=CARTESIAN_POINT('Ctrl Pts',(-0.16803277280837,1.,1.78690649988931));
#25730=CARTESIAN_POINT('Ctrl Pts',(-0.169936923908078,-1.,1.80561530633924));
#25731=CARTESIAN_POINT('Ctrl Pts',(-0.169936923908078,1.,1.80561530633924));
#25732=CARTESIAN_POINT('Ctrl Pts',(-0.171554770207306,-1.,1.82215766815414));
#25733=CARTESIAN_POINT('Ctrl Pts',(-0.171554770207306,1.,1.82215766815414));
#25734=CARTESIAN_POINT('Ctrl Pts',(-0.17288944289442,-1.,1.83658380530747));
#25735=CARTESIAN_POINT('Ctrl Pts',(-0.17288944289442,1.,1.83658380530747));
#25736=CARTESIAN_POINT('Ctrl Pts',(-0.173946627589401,-1.,1.84898113200543));
#25737=CARTESIAN_POINT('Ctrl Pts',(-0.173946627589401,1.,1.84898113200543));
#25738=CARTESIAN_POINT('Ctrl Pts',(-0.174735259276856,-1.,1.85948367089838));
#25739=CARTESIAN_POINT('Ctrl Pts',(-0.174735259276856,1.,1.85948367089838));
#25740=CARTESIAN_POINT('Ctrl Pts',(-0.175268337590901,-1.,1.86828349694972));
#25741=CARTESIAN_POINT('Ctrl Pts',(-0.175268337590901,1.,1.86828349694972));
#25742=CARTESIAN_POINT('Ctrl Pts',(-0.175563480746206,-1.,1.87563767773249));
#25743=CARTESIAN_POINT('Ctrl Pts',(-0.175563480746206,1.,1.87563767773249));
#25744=CARTESIAN_POINT('Ctrl Pts',(-0.175644148889271,-1.,1.88188663144846));
#25745=CARTESIAN_POINT('Ctrl Pts',(-0.175644148889271,1.,1.88188663144846));
#25746=CARTESIAN_POINT('Ctrl Pts',(-0.175538155840286,-1.,1.88742606272818));
#25747=CARTESIAN_POINT('Ctrl Pts',(-0.175538155840286,1.,1.88742606272818));
#25748=CARTESIAN_POINT('Ctrl Pts',(-0.175274276190664,-1.,1.89264630198279));
#25749=CARTESIAN_POINT('Ctrl Pts',(-0.175274276190664,1.,1.89264630198279));
#25750=CARTESIAN_POINT('Ctrl Pts',(-0.174879405091277,-1.,1.89788101117148));
#25751=CARTESIAN_POINT('Ctrl Pts',(-0.174879405091277,1.,1.89788101117148));
#25752=CARTESIAN_POINT('Ctrl Pts',(-0.174375518661222,-1.,1.90335253863003));
#25753=CARTESIAN_POINT('Ctrl Pts',(-0.174375518661222,1.,1.90335253863003));
#25754=CARTESIAN_POINT('Ctrl Pts',(-0.173776635257984,-1.,1.90911693975475));
#25755=CARTESIAN_POINT('Ctrl Pts',(-0.173776635257984,1.,1.90911693975475));
#25756=CARTESIAN_POINT('Ctrl Pts',(-0.173090695383619,-1.,1.91511429159681));
#25757=CARTESIAN_POINT('Ctrl Pts',(-0.173090695383619,1.,1.91511429159681));
#25758=CARTESIAN_POINT('Ctrl Pts',(-0.172321621259557,-1.,1.92122334398034));
#25759=CARTESIAN_POINT('Ctrl Pts',(-0.172321621259557,1.,1.92122334398034));
#25760=CARTESIAN_POINT('Ctrl Pts',(-0.17147119153296,-1.,1.92731093582));
#25761=CARTESIAN_POINT('Ctrl Pts',(-0.17147119153296,1.,1.92731093582));
#25762=CARTESIAN_POINT('Ctrl Pts',(-0.170541253116136,-1.,1.93329183155455));
#25763=CARTESIAN_POINT('Ctrl Pts',(-0.170541253116136,1.,1.93329183155455));
#25764=CARTESIAN_POINT('Ctrl Pts',(-0.169534904817425,-1.,1.93915639211497));
#25765=CARTESIAN_POINT('Ctrl Pts',(-0.169534904817425,1.,1.93915639211497));
#25766=CARTESIAN_POINT('Ctrl Pts',(-0.168455741607516,-1.,1.94493757756879));
#25767=CARTESIAN_POINT('Ctrl Pts',(-0.168455741607516,1.,1.94493757756879));
#25768=CARTESIAN_POINT('Ctrl Pts',(-0.167307501784469,-1.,1.95069027794286));
#25769=CARTESIAN_POINT('Ctrl Pts',(-0.167307501784469,1.,1.95069027794286));
#25770=CARTESIAN_POINT('Ctrl Pts',(-0.166093592002833,-1.,1.95646759718755));
#25771=CARTESIAN_POINT('Ctrl Pts',(-0.166093592002833,1.,1.95646759718755));
#25772=CARTESIAN_POINT('Ctrl Pts',(-0.1648165689203,-1.,1.96229379940174));
#25773=CARTESIAN_POINT('Ctrl Pts',(-0.1648165689203,1.,1.96229379940174));
#25774=CARTESIAN_POINT('Ctrl Pts',(-0.16347818545776,-1.,1.96816512678));
#25775=CARTESIAN_POINT('Ctrl Pts',(-0.16347818545776,1.,1.96816512678));
#25776=CARTESIAN_POINT('Ctrl Pts',(-0.162079693556302,-1.,1.97406280235204));
#25777=CARTESIAN_POINT('Ctrl Pts',(-0.162079693556302,1.,1.97406280235204));
#25778=CARTESIAN_POINT('Ctrl Pts',(-0.16062206078461,-1.,1.97996195437557));
#25779=CARTESIAN_POINT('Ctrl Pts',(-0.16062206078461,1.,1.97996195437557));
#25780=CARTESIAN_POINT('Ctrl Pts',(-0.159106226437289,-1.,1.98584238283279));
#25781=CARTESIAN_POINT('Ctrl Pts',(-0.159106226437289,1.,1.98584238283279));
#25782=CARTESIAN_POINT('Ctrl Pts',(-0.157533331459215,-1.,1.99169810931893));
#25783=CARTESIAN_POINT('Ctrl Pts',(-0.157533331459215,1.,1.99169810931893));
#25784=CARTESIAN_POINT('Ctrl Pts',(-0.155904629548775,-1.,1.99753284771487));
#25785=CARTESIAN_POINT('Ctrl Pts',(-0.155904629548775,1.,1.99753284771487));
#25786=CARTESIAN_POINT('Ctrl Pts',(-0.154221403049719,-1.,2.00335565310539));
#25787=CARTESIAN_POINT('Ctrl Pts',(-0.154221403049719,1.,2.00335565310539));
#25788=CARTESIAN_POINT('Ctrl Pts',(-0.152484883621452,-1.,2.00917680318426));
#25789=CARTESIAN_POINT('Ctrl Pts',(-0.152484883621452,1.,2.00917680318426));
#25790=CARTESIAN_POINT('Ctrl Pts',(-0.150696157673084,-1.,2.01500291940243));
#25791=CARTESIAN_POINT('Ctrl Pts',(-0.150696157673084,1.,2.01500291940243));
#25792=CARTESIAN_POINT('Ctrl Pts',(-0.148856124775343,-1.,2.02083464969897));
#25793=CARTESIAN_POINT('Ctrl Pts',(-0.148856124775343,1.,2.02083464969897));
#25794=CARTESIAN_POINT('Ctrl Pts',(-0.146965557332586,-1.,2.02666926182017));
#25795=CARTESIAN_POINT('Ctrl Pts',(-0.146965557332586,1.,2.02666926182017));
#25796=CARTESIAN_POINT('Ctrl Pts',(-0.145025140186058,-1.,2.03250223739941));
#25797=CARTESIAN_POINT('Ctrl Pts',(-0.145025140186058,1.,2.03250223739941));
#25798=CARTESIAN_POINT('Ctrl Pts',(-0.143035515058208,-1.,2.03832911025913));
#25799=CARTESIAN_POINT('Ctrl Pts',(-0.143035515058208,1.,2.03832911025913));
#25800=CARTESIAN_POINT('Ctrl Pts',(-0.140997332152546,-1.,2.04414757947919));
#25801=CARTESIAN_POINT('Ctrl Pts',(-0.140997332152546,1.,2.04414757947919));
#25802=CARTESIAN_POINT('Ctrl Pts',(-0.138911255368966,-1.,2.04995762001333));
#25803=CARTESIAN_POINT('Ctrl Pts',(-0.138911255368966,1.,2.04995762001333));
#25804=CARTESIAN_POINT('Ctrl Pts',(-0.136777941218044,-1.,2.0557604441427));
#25805=CARTESIAN_POINT('Ctrl Pts',(-0.136777941218044,1.,2.0557604441427));
#25806=CARTESIAN_POINT('Ctrl Pts',(-0.134598026192107,-1.,2.06155781517844));
#25807=CARTESIAN_POINT('Ctrl Pts',(-0.134598026192107,1.,2.06155781517844));
#25808=CARTESIAN_POINT('Ctrl Pts',(-0.13237211154771,-1.,2.06735123910319));
#25809=CARTESIAN_POINT('Ctrl Pts',(-0.13237211154771,1.,2.06735123910319));
#25810=CARTESIAN_POINT('Ctrl Pts',(-0.130100748328401,-1.,2.07314114713047));
#25811=CARTESIAN_POINT('Ctrl Pts',(-0.130100748328401,1.,2.07314114713047));
#25812=CARTESIAN_POINT('Ctrl Pts',(-0.127784445276116,-1.,2.07892715110967));
#25813=CARTESIAN_POINT('Ctrl Pts',(-0.127784445276116,1.,2.07892715110967));
#25814=CARTESIAN_POINT('Ctrl Pts',(-0.125423679412058,-1.,2.08470840653628));
#25815=CARTESIAN_POINT('Ctrl Pts',(-0.125423679412058,1.,2.08470840653628));
#25816=CARTESIAN_POINT('Ctrl Pts',(-0.123018905621083,-1.,2.09048392424826));
#25817=CARTESIAN_POINT('Ctrl Pts',(-0.123018905621083,1.,2.09048392424826));
#25818=CARTESIAN_POINT('Ctrl Pts',(-0.120570567965129,-1.,2.09625292867756));
#25819=CARTESIAN_POINT('Ctrl Pts',(-0.120570567965129,1.,2.09625292867756));
#25820=CARTESIAN_POINT('Ctrl Pts',(-0.118079107988368,-1.,2.10201512132945));
#25821=CARTESIAN_POINT('Ctrl Pts',(-0.118079107988368,1.,2.10201512132945));
#25822=CARTESIAN_POINT('Ctrl Pts',(-0.115544957687941,-1.,2.10777050261359));
#25823=CARTESIAN_POINT('Ctrl Pts',(-0.115544957687941,1.,2.10777050261359));
#25824=CARTESIAN_POINT('Ctrl Pts',(-0.112968534419746,-1.,2.11351924490335));
#25825=CARTESIAN_POINT('Ctrl Pts',(-0.112968534419746,1.,2.11351924490335));
#25826=CARTESIAN_POINT('Ctrl Pts',(-0.11035023613502,-1.,2.11926155590849));
#25827=CARTESIAN_POINT('Ctrl Pts',(-0.11035023613502,1.,2.11926155590849));
#25828=CARTESIAN_POINT('Ctrl Pts',(-0.107690435231068,-1.,2.12499752306927));
#25829=CARTESIAN_POINT('Ctrl Pts',(-0.107690435231068,1.,2.12499752306927));
#25830=CARTESIAN_POINT('Ctrl Pts',(-0.104989479152703,-1.,2.1307270488718));
#25831=CARTESIAN_POINT('Ctrl Pts',(-0.104989479152703,1.,2.1307270488718));
#25832=CARTESIAN_POINT('Ctrl Pts',(-0.102247700556064,-1.,2.13644992667052));
#25833=CARTESIAN_POINT('Ctrl Pts',(-0.102247700556064,1.,2.13644992667052));
#25834=CARTESIAN_POINT('Ctrl Pts',(-0.0994654261990745,-1.,2.14216588395974));
#25835=CARTESIAN_POINT('Ctrl Pts',(-0.0994654261990745,1.,2.14216588395974));
#25836=CARTESIAN_POINT('Ctrl Pts',(-0.0966429852305691,-1.,2.14787463531864));
#25837=CARTESIAN_POINT('Ctrl Pts',(-0.0966429852305691,1.,2.14787463531864));
#25838=CARTESIAN_POINT('Ctrl Pts',(-0.0937807218868348,-1.,2.15357593978377));
#25839=CARTESIAN_POINT('Ctrl Pts',(-0.0937807218868348,1.,2.15357593978377));
#25840=CARTESIAN_POINT('Ctrl Pts',(-0.0908789888108269,-1.,2.15926961544808));
#25841=CARTESIAN_POINT('Ctrl Pts',(-0.0908789888108269,1.,2.15926961544808));
#25842=CARTESIAN_POINT('Ctrl Pts',(-0.0879381291387825,-1.,2.16495552645275));
#25843=CARTESIAN_POINT('Ctrl Pts',(-0.0879381291387825,1.,2.16495552645275));
#25844=CARTESIAN_POINT('Ctrl Pts',(-0.0849584620835646,-1.,2.17063357871031));
#25845=CARTESIAN_POINT('Ctrl Pts',(-0.0849584620835646,1.,2.17063357871031));
#25846=CARTESIAN_POINT('Ctrl Pts',(-0.0819402680871942,-1.,2.1763037121106));
#25847=CARTESIAN_POINT('Ctrl Pts',(-0.0819402680871942,1.,2.1763037121106));
#25848=CARTESIAN_POINT('Ctrl Pts',(-0.078883772768323,-1.,2.18196589448304));
#25849=CARTESIAN_POINT('Ctrl Pts',(-0.078883772768323,1.,2.18196589448304));
#25850=CARTESIAN_POINT('Ctrl Pts',(-0.0757891465833414,-1.,2.1876201139874));
#25851=CARTESIAN_POINT('Ctrl Pts',(-0.0757891465833414,1.,2.1876201139874));
#25852=CARTESIAN_POINT('Ctrl Pts',(-0.0732830357304279,-1.,2.19213712012956));
#25853=CARTESIAN_POINT('Ctrl Pts',(-0.0732830357304279,1.,2.19213712012956));
#25854=CARTESIAN_POINT('Ctrl Pts',(-0.071386377952463,-1.,2.19552129483562));
#25855=CARTESIAN_POINT('Ctrl Pts',(-0.071386377952463,1.,2.19552129483562));
#25856=CARTESIAN_POINT('Ctrl Pts',(-0.0701143536324929,-1.,2.19777582085261));
#25857=CARTESIAN_POINT('Ctrl Pts',(-0.0701143536324929,1.,2.19777582085261));
#25858=CARTESIAN_POINT('Ctrl Pts',(-0.0694764450219586,-1.,2.19890268624765));
#25859=CARTESIAN_POINT('Ctrl Pts',(-0.0694764450219586,1.,2.19890268624765));
#25860=CARTESIAN_POINT('',(-0.163289472382896,1.,1.74236521665491));
#25861=CARTESIAN_POINT('Ctrl Pts',(-0.163289472382896,1.,1.74236521665491));
#25862=CARTESIAN_POINT('Ctrl Pts',(-0.163814161002474,1.,1.74720349503904));
#25863=CARTESIAN_POINT('Ctrl Pts',(-0.164834765708484,1.,1.75666056640041));
#25864=CARTESIAN_POINT('Ctrl Pts',(-0.166279355148738,1.,1.77018771687692));
#25865=CARTESIAN_POINT('Ctrl Pts',(-0.16803277280837,1.,1.78690649988931));
#25866=CARTESIAN_POINT('Ctrl Pts',(-0.169936923908078,1.,1.80561530633924));
#25867=CARTESIAN_POINT('Ctrl Pts',(-0.171554770207306,1.,1.82215766815414));
#25868=CARTESIAN_POINT('Ctrl Pts',(-0.17288944289442,1.,1.83658380530747));
#25869=CARTESIAN_POINT('Ctrl Pts',(-0.173946627589401,1.,1.84898113200543));
#25870=CARTESIAN_POINT('Ctrl Pts',(-0.174735259276856,1.,1.85948367089838));
#25871=CARTESIAN_POINT('Ctrl Pts',(-0.175268337590901,1.,1.86828349694972));
#25872=CARTESIAN_POINT('Ctrl Pts',(-0.175563480746206,1.,1.87563767773249));
#25873=CARTESIAN_POINT('Ctrl Pts',(-0.175644148889271,1.,1.88188663144846));
#25874=CARTESIAN_POINT('Ctrl Pts',(-0.175538155840286,1.,1.88742606272818));
#25875=CARTESIAN_POINT('Ctrl Pts',(-0.175274276190664,1.,1.89264630198279));
#25876=CARTESIAN_POINT('Ctrl Pts',(-0.174879405091277,1.,1.89788101117148));
#25877=CARTESIAN_POINT('Ctrl Pts',(-0.174375518661222,1.,1.90335253863003));
#25878=CARTESIAN_POINT('Ctrl Pts',(-0.173776635257984,1.,1.90911693975475));
#25879=CARTESIAN_POINT('Ctrl Pts',(-0.173090695383619,1.,1.91511429159681));
#25880=CARTESIAN_POINT('Ctrl Pts',(-0.172321621259557,1.,1.92122334398034));
#25881=CARTESIAN_POINT('Ctrl Pts',(-0.17147119153296,1.,1.92731093582));
#25882=CARTESIAN_POINT('Ctrl Pts',(-0.170541253116136,1.,1.93329183155455));
#25883=CARTESIAN_POINT('Ctrl Pts',(-0.169534904817425,1.,1.93915639211497));
#25884=CARTESIAN_POINT('Ctrl Pts',(-0.168455741607516,1.,1.94493757756879));
#25885=CARTESIAN_POINT('Ctrl Pts',(-0.167307501784469,1.,1.95069027794286));
#25886=CARTESIAN_POINT('Ctrl Pts',(-0.166093592002833,1.,1.95646759718755));
#25887=CARTESIAN_POINT('Ctrl Pts',(-0.1648165689203,1.,1.96229379940174));
#25888=CARTESIAN_POINT('Ctrl Pts',(-0.16347818545776,1.,1.96816512678));
#25889=CARTESIAN_POINT('Ctrl Pts',(-0.162079693556302,1.,1.97406280235204));
#25890=CARTESIAN_POINT('Ctrl Pts',(-0.16062206078461,1.,1.97996195437557));
#25891=CARTESIAN_POINT('Ctrl Pts',(-0.159106226437289,1.,1.98584238283279));
#25892=CARTESIAN_POINT('Ctrl Pts',(-0.157533331459215,1.,1.99169810931893));
#25893=CARTESIAN_POINT('Ctrl Pts',(-0.155904629548775,1.,1.99753284771487));
#25894=CARTESIAN_POINT('Ctrl Pts',(-0.154221403049719,1.,2.00335565310539));
#25895=CARTESIAN_POINT('Ctrl Pts',(-0.152484883621452,1.,2.00917680318426));
#25896=CARTESIAN_POINT('Ctrl Pts',(-0.150696157673084,1.,2.01500291940243));
#25897=CARTESIAN_POINT('Ctrl Pts',(-0.148856124775343,1.,2.02083464969897));
#25898=CARTESIAN_POINT('Ctrl Pts',(-0.146965557332586,1.,2.02666926182017));
#25899=CARTESIAN_POINT('Ctrl Pts',(-0.145025140186058,1.,2.03250223739941));
#25900=CARTESIAN_POINT('Ctrl Pts',(-0.143035515058208,1.,2.03832911025913));
#25901=CARTESIAN_POINT('Ctrl Pts',(-0.140997332152546,1.,2.04414757947919));
#25902=CARTESIAN_POINT('Ctrl Pts',(-0.138911255368966,1.,2.04995762001333));
#25903=CARTESIAN_POINT('Ctrl Pts',(-0.136777941218044,1.,2.0557604441427));
#25904=CARTESIAN_POINT('Ctrl Pts',(-0.134598026192107,1.,2.06155781517844));
#25905=CARTESIAN_POINT('Ctrl Pts',(-0.13237211154771,1.,2.06735123910319));
#25906=CARTESIAN_POINT('Ctrl Pts',(-0.130100748328401,1.,2.07314114713047));
#25907=CARTESIAN_POINT('Ctrl Pts',(-0.127784445276116,1.,2.07892715110967));
#25908=CARTESIAN_POINT('Ctrl Pts',(-0.125423679412058,1.,2.08470840653628));
#25909=CARTESIAN_POINT('Ctrl Pts',(-0.123018905621083,1.,2.09048392424826));
#25910=CARTESIAN_POINT('Ctrl Pts',(-0.120570567965129,1.,2.09625292867756));
#25911=CARTESIAN_POINT('Ctrl Pts',(-0.118079107988368,1.,2.10201512132945));
#25912=CARTESIAN_POINT('Ctrl Pts',(-0.115544957687941,1.,2.10777050261359));
#25913=CARTESIAN_POINT('Ctrl Pts',(-0.112968534419746,1.,2.11351924490335));
#25914=CARTESIAN_POINT('Ctrl Pts',(-0.11035023613502,1.,2.11926155590849));
#25915=CARTESIAN_POINT('Ctrl Pts',(-0.107690435231068,1.,2.12499752306927));
#25916=CARTESIAN_POINT('Ctrl Pts',(-0.104989479152703,1.,2.1307270488718));
#25917=CARTESIAN_POINT('Ctrl Pts',(-0.102247700556064,1.,2.13644992667052));
#25918=CARTESIAN_POINT('Ctrl Pts',(-0.0994654261990745,1.,2.14216588395974));
#25919=CARTESIAN_POINT('Ctrl Pts',(-0.0966429852305691,1.,2.14787463531864));
#25920=CARTESIAN_POINT('Ctrl Pts',(-0.0937807218868348,1.,2.15357593978377));
#25921=CARTESIAN_POINT('Ctrl Pts',(-0.0908789888108269,1.,2.15926961544808));
#25922=CARTESIAN_POINT('Ctrl Pts',(-0.0879381291387825,1.,2.16495552645275));
#25923=CARTESIAN_POINT('Ctrl Pts',(-0.0849584620835646,1.,2.17063357871031));
#25924=CARTESIAN_POINT('Ctrl Pts',(-0.0819402680871942,1.,2.1763037121106));
#25925=CARTESIAN_POINT('Ctrl Pts',(-0.078883772768323,1.,2.18196589448304));
#25926=CARTESIAN_POINT('Ctrl Pts',(-0.0757891465833414,1.,2.1876201139874));
#25927=CARTESIAN_POINT('Ctrl Pts',(-0.0732830357304279,1.,2.19213712012956));
#25928=CARTESIAN_POINT('Ctrl Pts',(-0.071386377952463,1.,2.19552129483562));
#25929=CARTESIAN_POINT('Ctrl Pts',(-0.0701143536324929,1.,2.19777582085261));
#25930=CARTESIAN_POINT('Ctrl Pts',(-0.0694764450219586,1.,2.19890268624765));
#25931=CARTESIAN_POINT('',(-0.163289472382897,0.,1.74236521665491));
#25932=CARTESIAN_POINT('Origin',(0.,0.,0.));
#25933=CARTESIAN_POINT('',(-0.383122945602004,1.,1.7075470150345));
#25934=CARTESIAN_POINT('Origin',(0.,1.,0.));
#25935=CARTESIAN_POINT('',(-0.383122945602004,0.,1.7075470150345));
#25936=CARTESIAN_POINT('Ctrl Pts',(-0.61342227326009,-1.,2.11275013067528));
#25937=CARTESIAN_POINT('Ctrl Pts',(-0.61342227326009,1.,2.11275013067528));
#25938=CARTESIAN_POINT('Ctrl Pts',(-0.61246736556225,-1.,2.11187554260142));
#25939=CARTESIAN_POINT('Ctrl Pts',(-0.61246736556225,1.,2.11187554260142));
#25940=CARTESIAN_POINT('Ctrl Pts',(-0.610560911691113,-1.,2.11012443807661));
#25941=CARTESIAN_POINT('Ctrl Pts',(-0.610560911691113,1.,2.11012443807661));
#25942=CARTESIAN_POINT('Ctrl Pts',(-0.607711315456826,-1.,2.10749199615859));
#25943=CARTESIAN_POINT('Ctrl Pts',(-0.607711315456826,1.,2.10749199615859));
#25944=CARTESIAN_POINT('Ctrl Pts',(-0.603932030738212,-1.,2.10397049887709));
#25945=CARTESIAN_POINT('Ctrl Pts',(-0.603932030738212,1.,2.10397049887709));
#25946=CARTESIAN_POINT('Ctrl Pts',(-0.599241616422144,-1.,2.09954930865331));
#25947=CARTESIAN_POINT('Ctrl Pts',(-0.599241616422144,1.,2.09954930865331));
#25948=CARTESIAN_POINT('Ctrl Pts',(-0.594585006052824,-1.,2.09510876220501));
#25949=CARTESIAN_POINT('Ctrl Pts',(-0.594585006052824,1.,2.09510876220501));
#25950=CARTESIAN_POINT('Ctrl Pts',(-0.589962365403189,-1.,2.09064881812053));
#25951=CARTESIAN_POINT('Ctrl Pts',(-0.589962365403189,1.,2.09064881812053));
#25952=CARTESIAN_POINT('Ctrl Pts',(-0.585373918990895,-1.,2.086169437277));
#25953=CARTESIAN_POINT('Ctrl Pts',(-0.585373918990895,1.,2.086169437277));
#25954=CARTESIAN_POINT('Ctrl Pts',(-0.580819952107257,-1.,2.08167059018138));
#25955=CARTESIAN_POINT('Ctrl Pts',(-0.580819952107257,1.,2.08167059018138));
#25956=CARTESIAN_POINT('Ctrl Pts',(-0.576300797416275,-1.,2.07715226767361));
#25957=CARTESIAN_POINT('Ctrl Pts',(-0.576300797416275,1.,2.07715226767361));
#25958=CARTESIAN_POINT('Ctrl Pts',(-0.571816823242411,-1.,2.07261449292757));
#25959=CARTESIAN_POINT('Ctrl Pts',(-0.571816823242411,1.,2.07261449292757));
#25960=CARTESIAN_POINT('Ctrl Pts',(-0.567368421181229,-1.,2.06805732997383));
#25961=CARTESIAN_POINT('Ctrl Pts',(-0.567368421181229,1.,2.06805732997383));
#25962=CARTESIAN_POINT('Ctrl Pts',(-0.562955993082574,-1.,2.06348090160697));
#25963=CARTESIAN_POINT('Ctrl Pts',(-0.562955993082574,1.,2.06348090160697));
#25964=CARTESIAN_POINT('Ctrl Pts',(-0.558579940185467,-1.,2.05888537756571));
#25965=CARTESIAN_POINT('Ctrl Pts',(-0.558579940185467,1.,2.05888537756571));
#25966=CARTESIAN_POINT('Ctrl Pts',(-0.55424065746411,-1.,2.05427091604482));
#25967=CARTESIAN_POINT('Ctrl Pts',(-0.55424065746411,1.,2.05427091604482));
#25968=CARTESIAN_POINT('Ctrl Pts',(-0.549938525150342,-1.,2.04963761077974));
#25969=CARTESIAN_POINT('Ctrl Pts',(-0.549938525150342,1.,2.04963761077974));
#25970=CARTESIAN_POINT('Ctrl Pts',(-0.545673903817348,-1.,2.0449854471456));
#25971=CARTESIAN_POINT('Ctrl Pts',(-0.545673903817348,1.,2.0449854471456));
#25972=CARTESIAN_POINT('Ctrl Pts',(-0.54144712061552,-1.,2.0403142269048));
#25973=CARTESIAN_POINT('Ctrl Pts',(-0.54144712061552,1.,2.0403142269048));
#25974=CARTESIAN_POINT('Ctrl Pts',(-0.537258489833134,-1.,2.03562362953993));
#25975=CARTESIAN_POINT('Ctrl Pts',(-0.537258489833134,1.,2.03562362953993));
#25976=CARTESIAN_POINT('Ctrl Pts',(-0.533108355132905,-1.,2.03091336214401));
#25977=CARTESIAN_POINT('Ctrl Pts',(-0.533108355132905,1.,2.03091336214401));
#25978=CARTESIAN_POINT('Ctrl Pts',(-0.528997127241911,-1.,2.02618329083289));
#25979=CARTESIAN_POINT('Ctrl Pts',(-0.528997127241911,1.,2.02618329083289));
#25980=CARTESIAN_POINT('Ctrl Pts',(-0.524925318333518,-1.,2.02143356304712));
#25981=CARTESIAN_POINT('Ctrl Pts',(-0.524925318333518,1.,2.02143356304712));
#25982=CARTESIAN_POINT('Ctrl Pts',(-0.520893590399428,-1.,2.01666477917305));
#25983=CARTESIAN_POINT('Ctrl Pts',(-0.520893590399428,1.,2.01666477917305));
#25984=CARTESIAN_POINT('Ctrl Pts',(-0.516902681728733,-1.,2.01187773939257));
#25985=CARTESIAN_POINT('Ctrl Pts',(-0.516902681728733,1.,2.01187773939257));
#25986=CARTESIAN_POINT('Ctrl Pts',(-0.512953306961814,-1.,2.00707309946955));
#25987=CARTESIAN_POINT('Ctrl Pts',(-0.512953306961814,1.,2.00707309946955));
#25988=CARTESIAN_POINT('Ctrl Pts',(-0.509046069886152,-1.,2.00225107134733));
#25989=CARTESIAN_POINT('Ctrl Pts',(-0.509046069886152,1.,2.00225107134733));
#25990=CARTESIAN_POINT('Ctrl Pts',(-0.505181361323011,-1.,1.99741107463567));
#25991=CARTESIAN_POINT('Ctrl Pts',(-0.505181361323011,1.,1.99741107463567));
#25992=CARTESIAN_POINT('Ctrl Pts',(-0.501359287727129,-1.,1.9925514912615));
#25993=CARTESIAN_POINT('Ctrl Pts',(-0.501359287727129,1.,1.9925514912615));
#25994=CARTESIAN_POINT('Ctrl Pts',(-0.497579909545564,-1.,1.98767044752929));
#25995=CARTESIAN_POINT('Ctrl Pts',(-0.497579909545564,1.,1.98767044752929));
#25996=CARTESIAN_POINT('Ctrl Pts',(-0.493843476541492,-1.,1.9827665876182));
#25997=CARTESIAN_POINT('Ctrl Pts',(-0.493843476541492,1.,1.9827665876182));
#25998=CARTESIAN_POINT('Ctrl Pts',(-0.490150627860955,-1.,1.97783973019229));
#25999=CARTESIAN_POINT('Ctrl Pts',(-0.490150627860955,1.,1.97783973019229));
#26000=CARTESIAN_POINT('Ctrl Pts',(-0.486502692907661,-1.,1.97289186263272));
#26001=CARTESIAN_POINT('Ctrl Pts',(-0.486502692907661,1.,1.97289186263272));
#26002=CARTESIAN_POINT('Ctrl Pts',(-0.482901662120687,-1.,1.96792703422358));
#26003=CARTESIAN_POINT('Ctrl Pts',(-0.482901662120687,1.,1.96792703422358));
#26004=CARTESIAN_POINT('Ctrl Pts',(-0.479349583074846,-1.,1.96294933055938));
#26005=CARTESIAN_POINT('Ctrl Pts',(-0.479349583074846,1.,1.96294933055938));
#26006=CARTESIAN_POINT('Ctrl Pts',(-0.475848034683172,-1.,1.95796111148175));
#26007=CARTESIAN_POINT('Ctrl Pts',(-0.475848034683172,1.,1.95796111148175));
#26008=CARTESIAN_POINT('Ctrl Pts',(-0.47239767226408,-1.,1.95296148278136));
#26009=CARTESIAN_POINT('Ctrl Pts',(-0.47239767226408,1.,1.95296148278136));
#26010=CARTESIAN_POINT('Ctrl Pts',(-0.468997482913158,-1.,1.94794381136524));
#26011=CARTESIAN_POINT('Ctrl Pts',(-0.468997482913158,1.,1.94794381136524));
#26012=CARTESIAN_POINT('Ctrl Pts',(-0.465645462026065,-1.,1.94289794196205));
#26013=CARTESIAN_POINT('Ctrl Pts',(-0.465645462026065,1.,1.94289794196205));
#26014=CARTESIAN_POINT('Ctrl Pts',(-0.462340031009087,-1.,1.93781486640834));
#26015=CARTESIAN_POINT('Ctrl Pts',(-0.462340031009087,1.,1.93781486640834));
#26016=CARTESIAN_POINT('Ctrl Pts',(-0.459081234547931,-1.,1.93269066517936));
#26017=CARTESIAN_POINT('Ctrl Pts',(-0.459081234547931,1.,1.93269066517936));
#26018=CARTESIAN_POINT('Ctrl Pts',(-0.455872005174335,-1.,1.92753067150461));
#26019=CARTESIAN_POINT('Ctrl Pts',(-0.455872005174335,1.,1.92753067150461));
#26020=CARTESIAN_POINT('Ctrl Pts',(-0.452719478359356,-1.,1.9223538064847));
#26021=CARTESIAN_POINT('Ctrl Pts',(-0.452719478359356,1.,1.9223538064847));
#26022=CARTESIAN_POINT('Ctrl Pts',(-0.449632260106572,-1.,1.91718342555717));
#26023=CARTESIAN_POINT('Ctrl Pts',(-0.449632260106572,1.,1.91718342555717));
#26024=CARTESIAN_POINT('Ctrl Pts',(-0.446617343485651,-1.,1.91203699981095));
#26025=CARTESIAN_POINT('Ctrl Pts',(-0.446617343485651,1.,1.91203699981095));
#26026=CARTESIAN_POINT('Ctrl Pts',(-0.44367755684917,-1.,1.90691756144906));
#26027=CARTESIAN_POINT('Ctrl Pts',(-0.44367755684917,1.,1.90691756144906));
#26028=CARTESIAN_POINT('Ctrl Pts',(-0.440807833704161,-1.,1.90180124389137));
#26029=CARTESIAN_POINT('Ctrl Pts',(-0.440807833704161,1.,1.90180124389137));
#26030=CARTESIAN_POINT('Ctrl Pts',(-0.437995003948443,-1.,1.89663648956549));
#26031=CARTESIAN_POINT('Ctrl Pts',(-0.437995003948443,1.,1.89663648956549));
#26032=CARTESIAN_POINT('Ctrl Pts',(-0.43522566096358,-1.,1.89136993975585));
#26033=CARTESIAN_POINT('Ctrl Pts',(-0.43522566096358,1.,1.89136993975585));
#26034=CARTESIAN_POINT('Ctrl Pts',(-0.432493038548833,-1.,1.88596913666828));
#26035=CARTESIAN_POINT('Ctrl Pts',(-0.432493038548833,1.,1.88596913666828));
#26036=CARTESIAN_POINT('Ctrl Pts',(-0.429803062482217,-1.,1.88044229001778));
#26037=CARTESIAN_POINT('Ctrl Pts',(-0.429803062482217,1.,1.88044229001778));
#26038=CARTESIAN_POINT('Ctrl Pts',(-0.427183828518743,-1.,1.87486989291333));
#26039=CARTESIAN_POINT('Ctrl Pts',(-0.427183828518743,1.,1.87486989291333));
#26040=CARTESIAN_POINT('Ctrl Pts',(-0.424678177290876,-1.,1.8693780394412));
#26041=CARTESIAN_POINT('Ctrl Pts',(-0.424678177290876,1.,1.8693780394412));
#26042=CARTESIAN_POINT('Ctrl Pts',(-0.422327307417885,-1.,1.86408083333863));
#26043=CARTESIAN_POINT('Ctrl Pts',(-0.422327307417885,1.,1.86408083333863));
#26044=CARTESIAN_POINT('Ctrl Pts',(-0.420157287975583,-1.,1.8590328109667));
#26045=CARTESIAN_POINT('Ctrl Pts',(-0.420157287975583,1.,1.8590328109667));
#26046=CARTESIAN_POINT('Ctrl Pts',(-0.418164129144045,-1.,1.8541763285645));
#26047=CARTESIAN_POINT('Ctrl Pts',(-0.418164129144045,1.,1.8541763285645));
#26048=CARTESIAN_POINT('Ctrl Pts',(-0.416300022039885,-1.,1.84929312930314));
#26049=CARTESIAN_POINT('Ctrl Pts',(-0.416300022039885,1.,1.84929312930314));
#26050=CARTESIAN_POINT('Ctrl Pts',(-0.414487438255542,-1.,1.84405757074218));
#26051=CARTESIAN_POINT('Ctrl Pts',(-0.414487438255542,1.,1.84405757074218));
#26052=CARTESIAN_POINT('Ctrl Pts',(-0.412633125322945,-1.,1.8380895347617));
#26053=CARTESIAN_POINT('Ctrl Pts',(-0.412633125322945,1.,1.8380895347617));
#26054=CARTESIAN_POINT('Ctrl Pts',(-0.410641256301276,-1.,1.83100408895047));
#26055=CARTESIAN_POINT('Ctrl Pts',(-0.410641256301276,1.,1.83100408895047));
#26056=CARTESIAN_POINT('Ctrl Pts',(-0.408428948106227,-1.,1.82247022677562));
#26057=CARTESIAN_POINT('Ctrl Pts',(-0.408428948106227,1.,1.82247022677562));
#26058=CARTESIAN_POINT('Ctrl Pts',(-0.405933518407175,-1.,1.81223801812013));
#26059=CARTESIAN_POINT('Ctrl Pts',(-0.405933518407175,1.,1.81223801812013));
#26060=CARTESIAN_POINT('Ctrl Pts',(-0.403107976163396,-1.,1.80012077173238));
#26061=CARTESIAN_POINT('Ctrl Pts',(-0.403107976163396,1.,1.80012077173238));
#26062=CARTESIAN_POINT('Ctrl Pts',(-0.399919403774155,-1.,1.78598826343754));
#26063=CARTESIAN_POINT('Ctrl Pts',(-0.399919403774155,1.,1.78598826343754));
#26064=CARTESIAN_POINT('Ctrl Pts',(-0.396346196110688,-1.,1.76975560043442));
#26065=CARTESIAN_POINT('Ctrl Pts',(-0.396346196110688,1.,1.76975560043442));
#26066=CARTESIAN_POINT('Ctrl Pts',(-0.392375812285395,-1.,1.75137405310193));
#26067=CARTESIAN_POINT('Ctrl Pts',(-0.392375812285395,1.,1.75137405310193));
#26068=CARTESIAN_POINT('Ctrl Pts',(-0.388877023502615,-1.,1.73493170972829));
#26069=CARTESIAN_POINT('Ctrl Pts',(-0.388877023502615,1.,1.73493170972829));
#26070=CARTESIAN_POINT('Ctrl Pts',(-0.386070790323281,-1.,1.72162022244582));
#26071=CARTESIAN_POINT('Ctrl Pts',(-0.386070790323281,1.,1.72162022244582));
#26072=CARTESIAN_POINT('Ctrl Pts',(-0.384119047314215,-1.,1.71231062891398));
#26073=CARTESIAN_POINT('Ctrl Pts',(-0.384119047314215,1.,1.71231062891398));
#26074=CARTESIAN_POINT('Ctrl Pts',(-0.383122945602004,-1.,1.7075470150345));
#26075=CARTESIAN_POINT('Ctrl Pts',(-0.383122945602004,1.,1.7075470150345));
#26076=CARTESIAN_POINT('',(-0.61342227326009,1.,2.11275013067528));
#26077=CARTESIAN_POINT('Ctrl Pts',(-0.61342227326009,1.,2.11275013067528));
#26078=CARTESIAN_POINT('Ctrl Pts',(-0.61246736556225,1.,2.11187554260142));
#26079=CARTESIAN_POINT('Ctrl Pts',(-0.610560911691113,1.,2.11012443807661));
#26080=CARTESIAN_POINT('Ctrl Pts',(-0.607711315456826,1.,2.10749199615859));
#26081=CARTESIAN_POINT('Ctrl Pts',(-0.603932030738212,1.,2.10397049887709));
#26082=CARTESIAN_POINT('Ctrl Pts',(-0.599241616422144,1.,2.09954930865331));
#26083=CARTESIAN_POINT('Ctrl Pts',(-0.594585006052824,1.,2.09510876220501));
#26084=CARTESIAN_POINT('Ctrl Pts',(-0.589962365403189,1.,2.09064881812053));
#26085=CARTESIAN_POINT('Ctrl Pts',(-0.585373918990895,1.,2.086169437277));
#26086=CARTESIAN_POINT('Ctrl Pts',(-0.580819952107257,1.,2.08167059018138));
#26087=CARTESIAN_POINT('Ctrl Pts',(-0.576300797416275,1.,2.07715226767361));
#26088=CARTESIAN_POINT('Ctrl Pts',(-0.571816823242411,1.,2.07261449292757));
#26089=CARTESIAN_POINT('Ctrl Pts',(-0.567368421181229,1.,2.06805732997383));
#26090=CARTESIAN_POINT('Ctrl Pts',(-0.562955993082574,1.,2.06348090160697));
#26091=CARTESIAN_POINT('Ctrl Pts',(-0.558579940185467,1.,2.05888537756571));
#26092=CARTESIAN_POINT('Ctrl Pts',(-0.55424065746411,1.,2.05427091604482));
#26093=CARTESIAN_POINT('Ctrl Pts',(-0.549938525150342,1.,2.04963761077974));
#26094=CARTESIAN_POINT('Ctrl Pts',(-0.545673903817348,1.,2.0449854471456));
#26095=CARTESIAN_POINT('Ctrl Pts',(-0.54144712061552,1.,2.0403142269048));
#26096=CARTESIAN_POINT('Ctrl Pts',(-0.537258489833134,1.,2.03562362953993));
#26097=CARTESIAN_POINT('Ctrl Pts',(-0.533108355132905,1.,2.03091336214401));
#26098=CARTESIAN_POINT('Ctrl Pts',(-0.528997127241911,1.,2.02618329083289));
#26099=CARTESIAN_POINT('Ctrl Pts',(-0.524925318333518,1.,2.02143356304712));
#26100=CARTESIAN_POINT('Ctrl Pts',(-0.520893590399428,1.,2.01666477917305));
#26101=CARTESIAN_POINT('Ctrl Pts',(-0.516902681728733,1.,2.01187773939257));
#26102=CARTESIAN_POINT('Ctrl Pts',(-0.512953306961814,1.,2.00707309946955));
#26103=CARTESIAN_POINT('Ctrl Pts',(-0.509046069886152,1.,2.00225107134733));
#26104=CARTESIAN_POINT('Ctrl Pts',(-0.505181361323011,1.,1.99741107463567));
#26105=CARTESIAN_POINT('Ctrl Pts',(-0.501359287727129,1.,1.9925514912615));
#26106=CARTESIAN_POINT('Ctrl Pts',(-0.497579909545564,1.,1.98767044752929));
#26107=CARTESIAN_POINT('Ctrl Pts',(-0.493843476541492,1.,1.9827665876182));
#26108=CARTESIAN_POINT('Ctrl Pts',(-0.490150627860955,1.,1.97783973019229));
#26109=CARTESIAN_POINT('Ctrl Pts',(-0.486502692907661,1.,1.97289186263272));
#26110=CARTESIAN_POINT('Ctrl Pts',(-0.482901662120687,1.,1.96792703422358));
#26111=CARTESIAN_POINT('Ctrl Pts',(-0.479349583074846,1.,1.96294933055938));
#26112=CARTESIAN_POINT('Ctrl Pts',(-0.475848034683172,1.,1.95796111148175));
#26113=CARTESIAN_POINT('Ctrl Pts',(-0.47239767226408,1.,1.95296148278136));
#26114=CARTESIAN_POINT('Ctrl Pts',(-0.468997482913158,1.,1.94794381136524));
#26115=CARTESIAN_POINT('Ctrl Pts',(-0.465645462026065,1.,1.94289794196205));
#26116=CARTESIAN_POINT('Ctrl Pts',(-0.462340031009087,1.,1.93781486640834));
#26117=CARTESIAN_POINT('Ctrl Pts',(-0.459081234547931,1.,1.93269066517936));
#26118=CARTESIAN_POINT('Ctrl Pts',(-0.455872005174335,1.,1.92753067150461));
#26119=CARTESIAN_POINT('Ctrl Pts',(-0.452719478359356,1.,1.9223538064847));
#26120=CARTESIAN_POINT('Ctrl Pts',(-0.449632260106572,1.,1.91718342555717));
#26121=CARTESIAN_POINT('Ctrl Pts',(-0.446617343485651,1.,1.91203699981095));
#26122=CARTESIAN_POINT('Ctrl Pts',(-0.44367755684917,1.,1.90691756144906));
#26123=CARTESIAN_POINT('Ctrl Pts',(-0.440807833704161,1.,1.90180124389137));
#26124=CARTESIAN_POINT('Ctrl Pts',(-0.437995003948443,1.,1.89663648956549));
#26125=CARTESIAN_POINT('Ctrl Pts',(-0.43522566096358,1.,1.89136993975585));
#26126=CARTESIAN_POINT('Ctrl Pts',(-0.432493038548833,1.,1.88596913666828));
#26127=CARTESIAN_POINT('Ctrl Pts',(-0.429803062482217,1.,1.88044229001778));
#26128=CARTESIAN_POINT('Ctrl Pts',(-0.427183828518743,1.,1.87486989291333));
#26129=CARTESIAN_POINT('Ctrl Pts',(-0.424678177290876,1.,1.8693780394412));
#26130=CARTESIAN_POINT('Ctrl Pts',(-0.422327307417885,1.,1.86408083333863));
#26131=CARTESIAN_POINT('Ctrl Pts',(-0.420157287975583,1.,1.8590328109667));
#26132=CARTESIAN_POINT('Ctrl Pts',(-0.418164129144045,1.,1.8541763285645));
#26133=CARTESIAN_POINT('Ctrl Pts',(-0.416300022039885,1.,1.84929312930314));
#26134=CARTESIAN_POINT('Ctrl Pts',(-0.414487438255542,1.,1.84405757074218));
#26135=CARTESIAN_POINT('Ctrl Pts',(-0.412633125322945,1.,1.8380895347617));
#26136=CARTESIAN_POINT('Ctrl Pts',(-0.410641256301276,1.,1.83100408895047));
#26137=CARTESIAN_POINT('Ctrl Pts',(-0.408428948106227,1.,1.82247022677562));
#26138=CARTESIAN_POINT('Ctrl Pts',(-0.405933518407175,1.,1.81223801812013));
#26139=CARTESIAN_POINT('Ctrl Pts',(-0.403107976163396,1.,1.80012077173238));
#26140=CARTESIAN_POINT('Ctrl Pts',(-0.399919403774155,1.,1.78598826343754));
#26141=CARTESIAN_POINT('Ctrl Pts',(-0.396346196110688,1.,1.76975560043442));
#26142=CARTESIAN_POINT('Ctrl Pts',(-0.392375812285395,1.,1.75137405310193));
#26143=CARTESIAN_POINT('Ctrl Pts',(-0.388877023502615,1.,1.73493170972829));
#26144=CARTESIAN_POINT('Ctrl Pts',(-0.386070790323281,1.,1.72162022244582));
#26145=CARTESIAN_POINT('Ctrl Pts',(-0.384119047314215,1.,1.71231062891398));
#26146=CARTESIAN_POINT('Ctrl Pts',(-0.383122945602004,1.,1.7075470150345));
#26147=CARTESIAN_POINT('',(-0.61342227326009,0.,2.11275013067528));
#26148=CARTESIAN_POINT('Origin',(-0.745574324794401,0.,2.0698113262342));
#26149=CARTESIAN_POINT('',(-0.745574324794401,1.,2.0698113262342));
#26150=CARTESIAN_POINT('',(-0.61342227326009,1.,2.11275013067528));
#26151=CARTESIAN_POINT('',(-0.745574324794401,0.,2.0698113262342));
#26152=CARTESIAN_POINT('Ctrl Pts',(-0.693717979106306,-1.,1.60662857109684));
#26153=CARTESIAN_POINT('Ctrl Pts',(-0.693717979106306,1.,1.60662857109684));
#26154=CARTESIAN_POINT('Ctrl Pts',(-0.695712097881194,-1.,1.61106790958151));
#26155=CARTESIAN_POINT('Ctrl Pts',(-0.695712097881194,1.,1.61106790958151));
#26156=CARTESIAN_POINT('Ctrl Pts',(-0.699605146405088,-1.,1.61974673472612));
#26157=CARTESIAN_POINT('Ctrl Pts',(-0.699605146405088,1.,1.61974673472612));
#26158=CARTESIAN_POINT('Ctrl Pts',(-0.705159151988319,-1.,1.63216541664676));
#26159=CARTESIAN_POINT('Ctrl Pts',(-0.705159151988319,1.,1.63216541664676));
#26160=CARTESIAN_POINT('Ctrl Pts',(-0.711993139355394,-1.,1.64752408832016));
#26161=CARTESIAN_POINT('Ctrl Pts',(-0.711993139355394,1.,1.64752408832016));
#26162=CARTESIAN_POINT('Ctrl Pts',(-0.719585433804282,-1.,1.6647288055568));
#26163=CARTESIAN_POINT('Ctrl Pts',(-0.719585433804282,1.,1.6647288055568));
#26164=CARTESIAN_POINT('Ctrl Pts',(-0.726235967997433,-1.,1.67996158455503));
#26165=CARTESIAN_POINT('Ctrl Pts',(-0.726235967997433,1.,1.67996158455503));
#26166=CARTESIAN_POINT('Ctrl Pts',(-0.731963238697195,-1.,1.69326921975743));
#26167=CARTESIAN_POINT('Ctrl Pts',(-0.731963238697195,1.,1.69326921975743));
#26168=CARTESIAN_POINT('Ctrl Pts',(-0.736799665724771,-1.,1.70473309006121));
#26169=CARTESIAN_POINT('Ctrl Pts',(-0.736799665724771,1.,1.70473309006121));
#26170=CARTESIAN_POINT('Ctrl Pts',(-0.740795162032088,-1.,1.71447789751927));
#26171=CARTESIAN_POINT('Ctrl Pts',(-0.740795162032088,1.,1.71447789751927));
#26172=CARTESIAN_POINT('Ctrl Pts',(-0.744021445433764,-1.,1.7226822991693));
#26173=CARTESIAN_POINT('Ctrl Pts',(-0.744021445433764,1.,1.7226822991693));
#26174=CARTESIAN_POINT('Ctrl Pts',(-0.746574710096436,-1.,1.72958533647399));
#26175=CARTESIAN_POINT('Ctrl Pts',(-0.746574710096436,1.,1.72958533647399));
#26176=CARTESIAN_POINT('Ctrl Pts',(-0.748582462954855,-1.,1.73550351679848));
#26177=CARTESIAN_POINT('Ctrl Pts',(-0.748582462954855,1.,1.73550351679848));
#26178=CARTESIAN_POINT('Ctrl Pts',(-0.75019343597954,-1.,1.74080458266705));
#26179=CARTESIAN_POINT('Ctrl Pts',(-0.75019343597954,1.,1.74080458266705));
#26180=CARTESIAN_POINT('Ctrl Pts',(-0.751555614163629,-1.,1.74585086852298));
#26181=CARTESIAN_POINT('Ctrl Pts',(-0.751555614163629,1.,1.74585086852298));
#26182=CARTESIAN_POINT('Ctrl Pts',(-0.752797683531377,-1.,1.75095139468809));
#26183=CARTESIAN_POINT('Ctrl Pts',(-0.752797683531377,1.,1.75095139468809));
#26184=CARTESIAN_POINT('Ctrl Pts',(-0.75400925402848,-1.,1.75631083600175));
#26185=CARTESIAN_POINT('Ctrl Pts',(-0.75400925402848,1.,1.75631083600175));
#26186=CARTESIAN_POINT('Ctrl Pts',(-0.755220979975262,-1.,1.7619781724032));
#26187=CARTESIAN_POINT('Ctrl Pts',(-0.755220979975262,1.,1.7619781724032));
#26188=CARTESIAN_POINT('Ctrl Pts',(-0.756421896028403,-1.,1.76789396003141));
#26189=CARTESIAN_POINT('Ctrl Pts',(-0.756421896028403,1.,1.76789396003141));
#26190=CARTESIAN_POINT('Ctrl Pts',(-0.757578264077238,-1.,1.77394167108342));
#26191=CARTESIAN_POINT('Ctrl Pts',(-0.757578264077238,1.,1.77394167108342));
#26192=CARTESIAN_POINT('Ctrl Pts',(-0.75865062667738,-1.,1.77999411220912));
#26193=CARTESIAN_POINT('Ctrl Pts',(-0.75865062667738,1.,1.77999411220912));
#26194=CARTESIAN_POINT('Ctrl Pts',(-0.759614401109868,-1.,1.78596964884526));
#26195=CARTESIAN_POINT('Ctrl Pts',(-0.759614401109868,1.,1.78596964884526));
#26196=CARTESIAN_POINT('Ctrl Pts',(-0.760469555880425,-1.,1.79185815610802));
#26197=CARTESIAN_POINT('Ctrl Pts',(-0.760469555880425,1.,1.79185815610802));
#26198=CARTESIAN_POINT('Ctrl Pts',(-0.761229695230359,-1.,1.79768986997735));
#26199=CARTESIAN_POINT('Ctrl Pts',(-0.761229695230359,1.,1.79768986997735));
#26200=CARTESIAN_POINT('Ctrl Pts',(-0.761915336443516,-1.,1.80351583877334));
#26201=CARTESIAN_POINT('Ctrl Pts',(-0.761915336443516,1.,1.80351583877334));
#26202=CARTESIAN_POINT('Ctrl Pts',(-0.762546129464036,-1.,1.80938551463989));
#26203=CARTESIAN_POINT('Ctrl Pts',(-0.762546129464036,1.,1.80938551463989));
#26204=CARTESIAN_POINT('Ctrl Pts',(-0.763132003836783,-1.,1.81532118405566));
#26205=CARTESIAN_POINT('Ctrl Pts',(-0.763132003836783,1.,1.81532118405566));
#26206=CARTESIAN_POINT('Ctrl Pts',(-0.763673465462854,-1.,1.82131873145297));
#26207=CARTESIAN_POINT('Ctrl Pts',(-0.763673465462854,1.,1.82131873145297));
#26208=CARTESIAN_POINT('Ctrl Pts',(-0.764165902606055,-1.,1.8273599120008));
#26209=CARTESIAN_POINT('Ctrl Pts',(-0.764165902606055,1.,1.8273599120008));
#26210=CARTESIAN_POINT('Ctrl Pts',(-0.764602549687845,-1.,1.8334207722714));
#26211=CARTESIAN_POINT('Ctrl Pts',(-0.764602549687845,1.,1.8334207722714));
#26212=CARTESIAN_POINT('Ctrl Pts',(-0.764978057881687,-1.,1.83948181064823));
#26213=CARTESIAN_POINT('Ctrl Pts',(-0.764978057881687,1.,1.83948181064823));
#26214=CARTESIAN_POINT('Ctrl Pts',(-0.765291664861971,-1.,1.8455369887591));
#26215=CARTESIAN_POINT('Ctrl Pts',(-0.765291664861971,1.,1.8455369887591));
#26216=CARTESIAN_POINT('Ctrl Pts',(-0.765545710619023,-1.,1.85158945130054));
#26217=CARTESIAN_POINT('Ctrl Pts',(-0.765545710619023,1.,1.85158945130054));
#26218=CARTESIAN_POINT('Ctrl Pts',(-0.765744212909305,-1.,1.85764741390391));
#26219=CARTESIAN_POINT('Ctrl Pts',(-0.765744212909305,1.,1.85764741390391));
#26220=CARTESIAN_POINT('Ctrl Pts',(-0.765891519092557,-1.,1.86372027063314));
#26221=CARTESIAN_POINT('Ctrl Pts',(-0.765891519092557,1.,1.86372027063314));
#26222=CARTESIAN_POINT('Ctrl Pts',(-0.765990708546111,-1.,1.86981398314345));
#26223=CARTESIAN_POINT('Ctrl Pts',(-0.765990708546111,1.,1.86981398314345));
#26224=CARTESIAN_POINT('Ctrl Pts',(-0.766042837036759,-1.,1.87592888967886));
#26225=CARTESIAN_POINT('Ctrl Pts',(-0.766042837036759,1.,1.87592888967886));
#26226=CARTESIAN_POINT('Ctrl Pts',(-0.766047794851869,-1.,1.88206215302561));
#26227=CARTESIAN_POINT('Ctrl Pts',(-0.766047794851869,1.,1.88206215302561));
#26228=CARTESIAN_POINT('Ctrl Pts',(-0.76600483706209,-1.,1.88820926433409));
#26229=CARTESIAN_POINT('Ctrl Pts',(-0.76600483706209,1.,1.88820926433409));
#26230=CARTESIAN_POINT('Ctrl Pts',(-0.765913193856979,-1.,1.89436577771389));
#26231=CARTESIAN_POINT('Ctrl Pts',(-0.765913193856979,1.,1.89436577771389));
#26232=CARTESIAN_POINT('Ctrl Pts',(-0.765772772593395,-1.,1.90052930393599));
#26233=CARTESIAN_POINT('Ctrl Pts',(-0.765772772593395,1.,1.90052930393599));
#26234=CARTESIAN_POINT('Ctrl Pts',(-0.765584196937936,-1.,1.90669961402362));
#26235=CARTESIAN_POINT('Ctrl Pts',(-0.765584196937936,1.,1.90669961402362));
#26236=CARTESIAN_POINT('Ctrl Pts',(-0.765348465884739,-1.,1.91287765805174));
#26237=CARTESIAN_POINT('Ctrl Pts',(-0.765348465884739,1.,1.91287765805174));
#26238=CARTESIAN_POINT('Ctrl Pts',(-0.765066729667095,-1.,1.91906491634197));
#26239=CARTESIAN_POINT('Ctrl Pts',(-0.765066729667095,1.,1.91906491634197));
#26240=CARTESIAN_POINT('Ctrl Pts',(-0.764740025488189,-1.,1.92526263537041));
#26241=CARTESIAN_POINT('Ctrl Pts',(-0.764740025488189,1.,1.92526263537041));
#26242=CARTESIAN_POINT('Ctrl Pts',(-0.764369010673889,-1.,1.93147105496367));
#26243=CARTESIAN_POINT('Ctrl Pts',(-0.764369010673889,1.,1.93147105496367));
#26244=CARTESIAN_POINT('Ctrl Pts',(-0.763954049121393,-1.,1.93768964875867));
#26245=CARTESIAN_POINT('Ctrl Pts',(-0.763954049121393,1.,1.93768964875867));
#26246=CARTESIAN_POINT('Ctrl Pts',(-0.76349533353858,-1.,1.94391746617626));
#26247=CARTESIAN_POINT('Ctrl Pts',(-0.76349533353858,1.,1.94391746617626));
#26248=CARTESIAN_POINT('Ctrl Pts',(-0.762992990878774,-1.,1.95015342590025));
#26249=CARTESIAN_POINT('Ctrl Pts',(-0.762992990878774,1.,1.95015342590025));
#26250=CARTESIAN_POINT('Ctrl Pts',(-0.762447203806263,-1.,1.95639665309893));
#26251=CARTESIAN_POINT('Ctrl Pts',(-0.762447203806263,1.,1.95639665309893));
#26252=CARTESIAN_POINT('Ctrl Pts',(-0.761858300014575,-1.,1.96264672744229));
#26253=CARTESIAN_POINT('Ctrl Pts',(-0.761858300014575,1.,1.96264672744229));
#26254=CARTESIAN_POINT('Ctrl Pts',(-0.761226690483986,-1.,1.96890351582545));
#26255=CARTESIAN_POINT('Ctrl Pts',(-0.761226690483986,1.,1.96890351582545));
#26256=CARTESIAN_POINT('Ctrl Pts',(-0.760552825409855,-1.,1.97516705321521));
#26257=CARTESIAN_POINT('Ctrl Pts',(-0.760552825409855,1.,1.97516705321521));
#26258=CARTESIAN_POINT('Ctrl Pts',(-0.759837147452135,-1.,1.98143741418156));
#26259=CARTESIAN_POINT('Ctrl Pts',(-0.759837147452135,1.,1.98143741418156));
#26260=CARTESIAN_POINT('Ctrl Pts',(-0.759080037802243,-1.,1.98771456680806));
#26261=CARTESIAN_POINT('Ctrl Pts',(-0.759080037802243,1.,1.98771456680806));
#26262=CARTESIAN_POINT('Ctrl Pts',(-0.758281796766377,-1.,1.9939983109871));
#26263=CARTESIAN_POINT('Ctrl Pts',(-0.758281796766377,1.,1.9939983109871));
#26264=CARTESIAN_POINT('Ctrl Pts',(-0.757442676862341,-1.,2.00028834739072));
#26265=CARTESIAN_POINT('Ctrl Pts',(-0.757442676862341,1.,2.00028834739072));
#26266=CARTESIAN_POINT('Ctrl Pts',(-0.756562904646496,-1.,2.00658431587682));
#26267=CARTESIAN_POINT('Ctrl Pts',(-0.756562904646496,1.,2.00658431587682));
#26268=CARTESIAN_POINT('Ctrl Pts',(-0.7556427049581,-1.,2.01288584328149));
#26269=CARTESIAN_POINT('Ctrl Pts',(-0.7556427049581,1.,2.01288584328149));
#26270=CARTESIAN_POINT('Ctrl Pts',(-0.75468233072352,-1.,2.01919259406003));
#26271=CARTESIAN_POINT('Ctrl Pts',(-0.75468233072352,1.,2.01919259406003));
#26272=CARTESIAN_POINT('Ctrl Pts',(-0.753682061113766,-1.,2.02550428623587));
#26273=CARTESIAN_POINT('Ctrl Pts',(-0.753682061113766,1.,2.02550428623587));
#26274=CARTESIAN_POINT('Ctrl Pts',(-0.752642180488104,-1.,2.03182068456467));
#26275=CARTESIAN_POINT('Ctrl Pts',(-0.752642180488104,1.,2.03182068456467));
#26276=CARTESIAN_POINT('Ctrl Pts',(-0.751562963361384,-1.,2.03814160092173));
#26277=CARTESIAN_POINT('Ctrl Pts',(-0.751562963361384,1.,2.03814160092173));
#26278=CARTESIAN_POINT('Ctrl Pts',(-0.750444657874758,-1.,2.04446689147754));
#26279=CARTESIAN_POINT('Ctrl Pts',(-0.750444657874758,1.,2.04446689147754));
#26280=CARTESIAN_POINT('Ctrl Pts',(-0.749287468663053,-1.,2.05079645591606));
#26281=CARTESIAN_POINT('Ctrl Pts',(-0.749287468663053,1.,2.05079645591606));
#26282=CARTESIAN_POINT('Ctrl Pts',(-0.748091554181101,-1.,2.05713023030263));
#26283=CARTESIAN_POINT('Ctrl Pts',(-0.748091554181101,1.,2.05713023030263));
#26284=CARTESIAN_POINT('Ctrl Pts',(-0.747103932785504,-1.,2.06220058927162));
#26285=CARTESIAN_POINT('Ctrl Pts',(-0.747103932785504,1.,2.06220058927162));
#26286=CARTESIAN_POINT('Ctrl Pts',(-0.746345871542696,-1.,2.06600523016401));
#26287=CARTESIAN_POINT('Ctrl Pts',(-0.746345871542696,1.,2.06600523016401));
#26288=CARTESIAN_POINT('Ctrl Pts',(-0.74583279137781,-1.,2.06854248895575));
#26289=CARTESIAN_POINT('Ctrl Pts',(-0.74583279137781,1.,2.06854248895575));
#26290=CARTESIAN_POINT('Ctrl Pts',(-0.745574324794401,-1.,2.0698113262342));
#26291=CARTESIAN_POINT('Ctrl Pts',(-0.745574324794401,1.,2.0698113262342));
#26292=CARTESIAN_POINT('',(-0.693717979106306,1.,1.60662857109684));
#26293=CARTESIAN_POINT('Ctrl Pts',(-0.693717979106306,1.,1.60662857109684));
#26294=CARTESIAN_POINT('Ctrl Pts',(-0.695712097881194,1.,1.61106790958151));
#26295=CARTESIAN_POINT('Ctrl Pts',(-0.699605146405088,1.,1.61974673472612));
#26296=CARTESIAN_POINT('Ctrl Pts',(-0.705159151988319,1.,1.63216541664676));
#26297=CARTESIAN_POINT('Ctrl Pts',(-0.711993139355394,1.,1.64752408832016));
#26298=CARTESIAN_POINT('Ctrl Pts',(-0.719585433804282,1.,1.6647288055568));
#26299=CARTESIAN_POINT('Ctrl Pts',(-0.726235967997433,1.,1.67996158455503));
#26300=CARTESIAN_POINT('Ctrl Pts',(-0.731963238697195,1.,1.69326921975743));
#26301=CARTESIAN_POINT('Ctrl Pts',(-0.736799665724771,1.,1.70473309006121));
#26302=CARTESIAN_POINT('Ctrl Pts',(-0.740795162032088,1.,1.71447789751927));
#26303=CARTESIAN_POINT('Ctrl Pts',(-0.744021445433764,1.,1.7226822991693));
#26304=CARTESIAN_POINT('Ctrl Pts',(-0.746574710096436,1.,1.72958533647399));
#26305=CARTESIAN_POINT('Ctrl Pts',(-0.748582462954855,1.,1.73550351679848));
#26306=CARTESIAN_POINT('Ctrl Pts',(-0.75019343597954,1.,1.74080458266705));
#26307=CARTESIAN_POINT('Ctrl Pts',(-0.751555614163629,1.,1.74585086852298));
#26308=CARTESIAN_POINT('Ctrl Pts',(-0.752797683531377,1.,1.75095139468809));
#26309=CARTESIAN_POINT('Ctrl Pts',(-0.75400925402848,1.,1.75631083600175));
#26310=CARTESIAN_POINT('Ctrl Pts',(-0.755220979975262,1.,1.7619781724032));
#26311=CARTESIAN_POINT('Ctrl Pts',(-0.756421896028403,1.,1.76789396003141));
#26312=CARTESIAN_POINT('Ctrl Pts',(-0.757578264077238,1.,1.77394167108342));
#26313=CARTESIAN_POINT('Ctrl Pts',(-0.75865062667738,1.,1.77999411220912));
#26314=CARTESIAN_POINT('Ctrl Pts',(-0.759614401109868,1.,1.78596964884526));
#26315=CARTESIAN_POINT('Ctrl Pts',(-0.760469555880425,1.,1.79185815610802));
#26316=CARTESIAN_POINT('Ctrl Pts',(-0.761229695230359,1.,1.79768986997735));
#26317=CARTESIAN_POINT('Ctrl Pts',(-0.761915336443516,1.,1.80351583877334));
#26318=CARTESIAN_POINT('Ctrl Pts',(-0.762546129464036,1.,1.80938551463989));
#26319=CARTESIAN_POINT('Ctrl Pts',(-0.763132003836783,1.,1.81532118405566));
#26320=CARTESIAN_POINT('Ctrl Pts',(-0.763673465462854,1.,1.82131873145297));
#26321=CARTESIAN_POINT('Ctrl Pts',(-0.764165902606055,1.,1.8273599120008));
#26322=CARTESIAN_POINT('Ctrl Pts',(-0.764602549687845,1.,1.8334207722714));
#26323=CARTESIAN_POINT('Ctrl Pts',(-0.764978057881687,1.,1.83948181064823));
#26324=CARTESIAN_POINT('Ctrl Pts',(-0.765291664861971,1.,1.8455369887591));
#26325=CARTESIAN_POINT('Ctrl Pts',(-0.765545710619023,1.,1.85158945130054));
#26326=CARTESIAN_POINT('Ctrl Pts',(-0.765744212909305,1.,1.85764741390391));
#26327=CARTESIAN_POINT('Ctrl Pts',(-0.765891519092557,1.,1.86372027063314));
#26328=CARTESIAN_POINT('Ctrl Pts',(-0.765990708546111,1.,1.86981398314345));
#26329=CARTESIAN_POINT('Ctrl Pts',(-0.766042837036759,1.,1.87592888967886));
#26330=CARTESIAN_POINT('Ctrl Pts',(-0.766047794851869,1.,1.88206215302561));
#26331=CARTESIAN_POINT('Ctrl Pts',(-0.76600483706209,1.,1.88820926433409));
#26332=CARTESIAN_POINT('Ctrl Pts',(-0.765913193856979,1.,1.89436577771389));
#26333=CARTESIAN_POINT('Ctrl Pts',(-0.765772772593395,1.,1.90052930393599));
#26334=CARTESIAN_POINT('Ctrl Pts',(-0.765584196937936,1.,1.90669961402362));
#26335=CARTESIAN_POINT('Ctrl Pts',(-0.765348465884739,1.,1.91287765805174));
#26336=CARTESIAN_POINT('Ctrl Pts',(-0.765066729667095,1.,1.91906491634197));
#26337=CARTESIAN_POINT('Ctrl Pts',(-0.764740025488189,1.,1.92526263537041));
#26338=CARTESIAN_POINT('Ctrl Pts',(-0.764369010673889,1.,1.93147105496367));
#26339=CARTESIAN_POINT('Ctrl Pts',(-0.763954049121393,1.,1.93768964875867));
#26340=CARTESIAN_POINT('Ctrl Pts',(-0.76349533353858,1.,1.94391746617626));
#26341=CARTESIAN_POINT('Ctrl Pts',(-0.762992990878774,1.,1.95015342590025));
#26342=CARTESIAN_POINT('Ctrl Pts',(-0.762447203806263,1.,1.95639665309893));
#26343=CARTESIAN_POINT('Ctrl Pts',(-0.761858300014575,1.,1.96264672744229));
#26344=CARTESIAN_POINT('Ctrl Pts',(-0.761226690483986,1.,1.96890351582545));
#26345=CARTESIAN_POINT('Ctrl Pts',(-0.760552825409855,1.,1.97516705321521));
#26346=CARTESIAN_POINT('Ctrl Pts',(-0.759837147452135,1.,1.98143741418156));
#26347=CARTESIAN_POINT('Ctrl Pts',(-0.759080037802243,1.,1.98771456680806));
#26348=CARTESIAN_POINT('Ctrl Pts',(-0.758281796766377,1.,1.9939983109871));
#26349=CARTESIAN_POINT('Ctrl Pts',(-0.757442676862341,1.,2.00028834739072));
#26350=CARTESIAN_POINT('Ctrl Pts',(-0.756562904646496,1.,2.00658431587682));
#26351=CARTESIAN_POINT('Ctrl Pts',(-0.7556427049581,1.,2.01288584328149));
#26352=CARTESIAN_POINT('Ctrl Pts',(-0.75468233072352,1.,2.01919259406003));
#26353=CARTESIAN_POINT('Ctrl Pts',(-0.753682061113766,1.,2.02550428623587));
#26354=CARTESIAN_POINT('Ctrl Pts',(-0.752642180488104,1.,2.03182068456467));
#26355=CARTESIAN_POINT('Ctrl Pts',(-0.751562963361384,1.,2.03814160092173));
#26356=CARTESIAN_POINT('Ctrl Pts',(-0.750444657874758,1.,2.04446689147754));
#26357=CARTESIAN_POINT('Ctrl Pts',(-0.749287468663053,1.,2.05079645591606));
#26358=CARTESIAN_POINT('Ctrl Pts',(-0.748091554181101,1.,2.05713023030263));
#26359=CARTESIAN_POINT('Ctrl Pts',(-0.747103932785504,1.,2.06220058927162));
#26360=CARTESIAN_POINT('Ctrl Pts',(-0.746345871542696,1.,2.06600523016401));
#26361=CARTESIAN_POINT('Ctrl Pts',(-0.74583279137781,1.,2.06854248895575));
#26362=CARTESIAN_POINT('Ctrl Pts',(-0.745574324794401,1.,2.0698113262342));
#26363=CARTESIAN_POINT('',(-0.693717979106306,0.,1.60662857109684));
#26364=CARTESIAN_POINT('Origin',(0.,0.,0.));
#26365=CARTESIAN_POINT('',(-0.892032620296855,1.,1.5055822144029));
#26366=CARTESIAN_POINT('Origin',(0.,1.,0.));
#26367=CARTESIAN_POINT('',(-0.892032620296855,0.,1.5055822144029));
#26368=CARTESIAN_POINT('Ctrl Pts',(-1.23627494547115,-1.,1.81978687191668));
#26369=CARTESIAN_POINT('Ctrl Pts',(-1.23627494547115,1.,1.81978687191668));
#26370=CARTESIAN_POINT('Ctrl Pts',(-1.23509651170476,-1.,1.81925017193666));
#26371=CARTESIAN_POINT('Ctrl Pts',(-1.23509651170476,1.,1.81925017193666));
#26372=CARTESIAN_POINT('Ctrl Pts',(-1.2327422452705,-1.,1.81817389921279));
#26373=CARTESIAN_POINT('Ctrl Pts',(-1.2327422452705,1.,1.81817389921279));
#26374=CARTESIAN_POINT('Ctrl Pts',(-1.2292186489137,-1.,1.8165508718364));
#26375=CARTESIAN_POINT('Ctrl Pts',(-1.2292186489137,1.,1.8165508718364));
#26376=CARTESIAN_POINT('Ctrl Pts',(-1.2245361330495,-1.,1.81436959210434));
#26377=CARTESIAN_POINT('Ctrl Pts',(-1.2245361330495,1.,1.81436959210434));
#26378=CARTESIAN_POINT('Ctrl Pts',(-1.21870906103557,-1.,1.81161420806656));
#26379=CARTESIAN_POINT('Ctrl Pts',(-1.21870906103557,1.,1.81161420806656));
#26380=CARTESIAN_POINT('Ctrl Pts',(-1.21290815708314,-1.,1.80882996917129));
#26381=CARTESIAN_POINT('Ctrl Pts',(-1.21290815708314,1.,1.80882996917129));
#26382=CARTESIAN_POINT('Ctrl Pts',(-1.20713356605475,-1.,1.80601678480707));
#26383=CARTESIAN_POINT('Ctrl Pts',(-1.20713356605475,1.,1.80601678480707));
#26384=CARTESIAN_POINT('Ctrl Pts',(-1.20138548938974,-1.,1.80317454838603));
#26385=CARTESIAN_POINT('Ctrl Pts',(-1.20138548938974,1.,1.80317454838603));
#26386=CARTESIAN_POINT('Ctrl Pts',(-1.19566418930242,-1.,1.80030314369879));
#26387=CARTESIAN_POINT('Ctrl Pts',(-1.19566418930242,1.,1.80030314369879));
#26388=CARTESIAN_POINT('Ctrl Pts',(-1.18996997934445,-1.,1.79740245923478));
#26389=CARTESIAN_POINT('Ctrl Pts',(-1.18996997934445,1.,1.79740245923478));
#26390=CARTESIAN_POINT('Ctrl Pts',(-1.18430321697432,-1.,1.79447240321515));
#26391=CARTESIAN_POINT('Ctrl Pts',(-1.18430321697432,1.,1.79447240321515));
#26392=CARTESIAN_POINT('Ctrl Pts',(-1.17866429440809,-1.,1.79151291552689));
#26393=CARTESIAN_POINT('Ctrl Pts',(-1.17866429440809,1.,1.79151291552689));
#26394=CARTESIAN_POINT('Ctrl Pts',(-1.17305363177328,-1.,1.78852398877616));
#26395=CARTESIAN_POINT('Ctrl Pts',(-1.17305363177328,1.,1.78852398877616));
#26396=CARTESIAN_POINT('Ctrl Pts',(-1.16747166312303,-1.,1.78550566040443));
#26397=CARTESIAN_POINT('Ctrl Pts',(-1.16747166312303,1.,1.78550566040443));
#26398=CARTESIAN_POINT('Ctrl Pts',(-1.16191881298499,-1.,1.78245795881009));
#26399=CARTESIAN_POINT('Ctrl Pts',(-1.16191881298499,1.,1.78245795881009));
#26400=CARTESIAN_POINT('Ctrl Pts',(-1.15639547194698,-1.,1.77938085564275));
#26401=CARTESIAN_POINT('Ctrl Pts',(-1.15639547194698,1.,1.77938085564275));
#26402=CARTESIAN_POINT('Ctrl Pts',(-1.15090197841515,-1.,1.7762742255701));
#26403=CARTESIAN_POINT('Ctrl Pts',(-1.15090197841515,1.,1.7762742255701));
#26404=CARTESIAN_POINT('Ctrl Pts',(-1.1454385822692,-1.,1.77313777896194));
#26405=CARTESIAN_POINT('Ctrl Pts',(-1.1454385822692,1.,1.77313777896194));
#26406=CARTESIAN_POINT('Ctrl Pts',(-1.14000548336975,-1.,1.76997111386769));
#26407=CARTESIAN_POINT('Ctrl Pts',(-1.14000548336975,1.,1.76997111386769));
#26408=CARTESIAN_POINT('Ctrl Pts',(-1.1346029180462,-1.,1.76677384551862));
#26409=CARTESIAN_POINT('Ctrl Pts',(-1.1346029180462,1.,1.76677384551862));
#26410=CARTESIAN_POINT('Ctrl Pts',(-1.12923123555075,-1.,1.7635457196617));
#26411=CARTESIAN_POINT('Ctrl Pts',(-1.12923123555075,1.,1.7635457196617));
#26412=CARTESIAN_POINT('Ctrl Pts',(-1.12389096855086,-1.,1.76028671825096));
#26413=CARTESIAN_POINT('Ctrl Pts',(-1.12389096855086,1.,1.76028671825096));
#26414=CARTESIAN_POINT('Ctrl Pts',(-1.11858293216763,-1.,1.75699720772105));
#26415=CARTESIAN_POINT('Ctrl Pts',(-1.11858293216763,1.,1.75699720772105));
#26416=CARTESIAN_POINT('Ctrl Pts',(-1.11330807582551,-1.,1.7536777209463));
#26417=CARTESIAN_POINT('Ctrl Pts',(-1.11330807582551,1.,1.7536777209463));
#26418=CARTESIAN_POINT('Ctrl Pts',(-1.10806728183007,-1.,1.7503286607592));
#26419=CARTESIAN_POINT('Ctrl Pts',(-1.10806728183007,1.,1.7503286607592));
#26420=CARTESIAN_POINT('Ctrl Pts',(-1.10286118991143,-1.,1.74695004214923));
#26421=CARTESIAN_POINT('Ctrl Pts',(-1.10286118991143,1.,1.74695004214923));
#26422=CARTESIAN_POINT('Ctrl Pts',(-1.09768999241225,-1.,1.74354119236208));
#26423=CARTESIAN_POINT('Ctrl Pts',(-1.09768999241225,1.,1.74354119236208));
#26424=CARTESIAN_POINT('Ctrl Pts',(-1.09255329056493,-1.,1.74010053962247));
#26425=CARTESIAN_POINT('Ctrl Pts',(-1.09255329056493,1.,1.74010053962247));
#26426=CARTESIAN_POINT('Ctrl Pts',(-1.08745056285427,-1.,1.73662628326091));
#26427=CARTESIAN_POINT('Ctrl Pts',(-1.08745056285427,1.,1.73662628326091));
#26428=CARTESIAN_POINT('Ctrl Pts',(-1.08238162784749,-1.,1.73311705663407));
#26429=CARTESIAN_POINT('Ctrl Pts',(-1.08238162784749,1.,1.73311705663407));
#26430=CARTESIAN_POINT('Ctrl Pts',(-1.0773470373727,-1.,1.72957248977424));
#26431=CARTESIAN_POINT('Ctrl Pts',(-1.0773470373727,1.,1.72957248977424));
#26432=CARTESIAN_POINT('Ctrl Pts',(-1.07234866990252,-1.,1.72599406198488));
#26433=CARTESIAN_POINT('Ctrl Pts',(-1.07234866990252,1.,1.72599406198488));
#26434=CARTESIAN_POINT('Ctrl Pts',(-1.06738966975462,-1.,1.72238500928453));
#26435=CARTESIAN_POINT('Ctrl Pts',(-1.06738966975462,1.,1.72238500928453));
#26436=CARTESIAN_POINT('Ctrl Pts',(-1.06247324680647,-1.,1.71874858456904));
#26437=CARTESIAN_POINT('Ctrl Pts',(-1.06247324680647,1.,1.71874858456904));
#26438=CARTESIAN_POINT('Ctrl Pts',(-1.05760163192479,-1.,1.7150865442702));
#26439=CARTESIAN_POINT('Ctrl Pts',(-1.05760163192479,1.,1.7150865442702));
#26440=CARTESIAN_POINT('Ctrl Pts',(-1.05277517202855,-1.,1.71139783543989));
#26441=CARTESIAN_POINT('Ctrl Pts',(-1.05277517202855,1.,1.71139783543989));
#26442=CARTESIAN_POINT('Ctrl Pts',(-1.04799085404995,-1.,1.70767646263649));
#26443=CARTESIAN_POINT('Ctrl Pts',(-1.04799085404995,1.,1.70767646263649));
#26444=CARTESIAN_POINT('Ctrl Pts',(-1.04324363334554,-1.,1.70391338707982));
#26445=CARTESIAN_POINT('Ctrl Pts',(-1.04324363334554,1.,1.70391338707982));
#26446=CARTESIAN_POINT('Ctrl Pts',(-1.03852922490789,-1.,1.70010052930962));
#26447=CARTESIAN_POINT('Ctrl Pts',(-1.03852922490789,1.,1.70010052930962));
#26448=CARTESIAN_POINT('Ctrl Pts',(-1.03384646003588,-1.,1.69623414782771));
#26449=CARTESIAN_POINT('Ctrl Pts',(-1.03384646003588,1.,1.69623414782771));
#26450=CARTESIAN_POINT('Ctrl Pts',(-1.02919977579147,-1.,1.69231840863458));
#26451=CARTESIAN_POINT('Ctrl Pts',(-1.02919977579147,1.,1.69231840863458));
#26452=CARTESIAN_POINT('Ctrl Pts',(-1.02460180535255,-1.,1.68836910178447));
#26453=CARTESIAN_POINT('Ctrl Pts',(-1.02460180535255,1.,1.68836910178447));
#26454=CARTESIAN_POINT('Ctrl Pts',(-1.02006795074201,-1.,1.68440578021706));
#26455=CARTESIAN_POINT('Ctrl Pts',(-1.02006795074201,1.,1.68440578021706));
#26456=CARTESIAN_POINT('Ctrl Pts',(-1.01561026162773,-1.,1.68044289894798));
#26457=CARTESIAN_POINT('Ctrl Pts',(-1.01561026162773,1.,1.68044289894798));
#26458=CARTESIAN_POINT('Ctrl Pts',(-1.01123236493511,-1.,1.67648246776464));
#26459=CARTESIAN_POINT('Ctrl Pts',(-1.01123236493511,1.,1.67648246776464));
#26460=CARTESIAN_POINT('Ctrl Pts',(-1.00692206696414,-1.,1.67250335383293));
#26461=CARTESIAN_POINT('Ctrl Pts',(-1.00692206696414,1.,1.67250335383293));
#26462=CARTESIAN_POINT('Ctrl Pts',(-1.00265091003727,-1.,1.66846059277303));
#26463=CARTESIAN_POINT('Ctrl Pts',(-1.00265091003727,1.,1.66846059277303));
#26464=CARTESIAN_POINT('Ctrl Pts',(-0.998389654952758,-1.,1.66430758030376));
#26465=CARTESIAN_POINT('Ctrl Pts',(-0.998389654952758,1.,1.66430758030376));
#26466=CARTESIAN_POINT('Ctrl Pts',(-0.994121836661306,-1.,1.66001553809947));
#26467=CARTESIAN_POINT('Ctrl Pts',(-0.994121836661306,1.,1.66001553809947));
#26468=CARTESIAN_POINT('Ctrl Pts',(-0.989855627854165,-1.,1.65559044289699));
#26469=CARTESIAN_POINT('Ctrl Pts',(-0.989855627854165,1.,1.65559044289699));
#26470=CARTESIAN_POINT('Ctrl Pts',(-0.985642622920821,-1.,1.65110016612638));
#26471=CARTESIAN_POINT('Ctrl Pts',(-0.985642622920821,1.,1.65110016612638));
#26472=CARTESIAN_POINT('Ctrl Pts',(-0.981562530939489,-1.,1.64665139190656));
#26473=CARTESIAN_POINT('Ctrl Pts',(-0.981562530939489,1.,1.64665139190656));
#26474=CARTESIAN_POINT('Ctrl Pts',(-0.977689794119416,-1.,1.64233990826687));
#26475=CARTESIAN_POINT('Ctrl Pts',(-0.977689794119416,1.,1.64233990826687));
#26476=CARTESIAN_POINT('Ctrl Pts',(-0.974066058287418,-1.,1.63820952658144));
#26477=CARTESIAN_POINT('Ctrl Pts',(-0.974066058287418,1.,1.63820952658144));
#26478=CARTESIAN_POINT('Ctrl Pts',(-0.970669715997509,-1.,1.63420665729798));
#26479=CARTESIAN_POINT('Ctrl Pts',(-0.970669715997509,1.,1.63420665729798));
#26480=CARTESIAN_POINT('Ctrl Pts',(-0.967387853230345,-1.,1.63013849959461));
#26481=CARTESIAN_POINT('Ctrl Pts',(-0.967387853230345,1.,1.63013849959461));
#26482=CARTESIAN_POINT('Ctrl Pts',(-0.964046107040536,-1.,1.62571930670187));
#26483=CARTESIAN_POINT('Ctrl Pts',(-0.964046107040536,1.,1.62571930670187));
#26484=CARTESIAN_POINT('Ctrl Pts',(-0.960438326101729,-1.,1.62061638140221));
#26485=CARTESIAN_POINT('Ctrl Pts',(-0.960438326101729,1.,1.62061638140221));
#26486=CARTESIAN_POINT('Ctrl Pts',(-0.956354422920671,-1.,1.61449324337085));
#26487=CARTESIAN_POINT('Ctrl Pts',(-0.956354422920671,1.,1.61449324337085));
#26488=CARTESIAN_POINT('Ctrl Pts',(-0.951613284356035,-1.,1.60706069896936));
#26489=CARTESIAN_POINT('Ctrl Pts',(-0.951613284356035,1.,1.60706069896936));
#26490=CARTESIAN_POINT('Ctrl Pts',(-0.946078063315257,-1.,1.59810042043673));
#26491=CARTESIAN_POINT('Ctrl Pts',(-0.946078063315257,1.,1.59810042043673));
#26492=CARTESIAN_POINT('Ctrl Pts',(-0.939646377893399,-1.,1.58744937487176));
#26493=CARTESIAN_POINT('Ctrl Pts',(-0.939646377893399,1.,1.58744937487176));
#26494=CARTESIAN_POINT('Ctrl Pts',(-0.932246680108685,-1.,1.57499388382243));
#26495=CARTESIAN_POINT('Ctrl Pts',(-0.932246680108685,1.,1.57499388382243));
#26496=CARTESIAN_POINT('Ctrl Pts',(-0.923832188944341,-1.,1.56065988578893));
#26497=CARTESIAN_POINT('Ctrl Pts',(-0.923832188944341,1.,1.56065988578893));
#26498=CARTESIAN_POINT('Ctrl Pts',(-0.914375919026456,-1.,1.54440491149498));
#26499=CARTESIAN_POINT('Ctrl Pts',(-0.914375919026456,1.,1.54440491149498));
#26500=CARTESIAN_POINT('Ctrl Pts',(-0.905967409625651,-1.,1.52984849887993));
#26501=CARTESIAN_POINT('Ctrl Pts',(-0.905967409625651,1.,1.52984849887993));
#26502=CARTESIAN_POINT('Ctrl Pts',(-0.899185047483511,-1.,1.51805569590094));
#26503=CARTESIAN_POINT('Ctrl Pts',(-0.899185047483511,1.,1.51805569590094));
#26504=CARTESIAN_POINT('Ctrl Pts',(-0.894452006964543,-1.,1.50980486806688));
#26505=CARTESIAN_POINT('Ctrl Pts',(-0.894452006964543,1.,1.50980486806688));
#26506=CARTESIAN_POINT('Ctrl Pts',(-0.892032620296855,-1.,1.5055822144029));
#26507=CARTESIAN_POINT('Ctrl Pts',(-0.892032620296855,1.,1.5055822144029));
#26508=CARTESIAN_POINT('',(-1.23627494547115,1.,1.81978687191668));
#26509=CARTESIAN_POINT('Ctrl Pts',(-1.23627494547115,1.,1.81978687191668));
#26510=CARTESIAN_POINT('Ctrl Pts',(-1.23509651170476,1.,1.81925017193666));
#26511=CARTESIAN_POINT('Ctrl Pts',(-1.2327422452705,1.,1.81817389921279));
#26512=CARTESIAN_POINT('Ctrl Pts',(-1.2292186489137,1.,1.8165508718364));
#26513=CARTESIAN_POINT('Ctrl Pts',(-1.2245361330495,1.,1.81436959210434));
#26514=CARTESIAN_POINT('Ctrl Pts',(-1.21870906103557,1.,1.81161420806656));
#26515=CARTESIAN_POINT('Ctrl Pts',(-1.21290815708314,1.,1.80882996917129));
#26516=CARTESIAN_POINT('Ctrl Pts',(-1.20713356605475,1.,1.80601678480707));
#26517=CARTESIAN_POINT('Ctrl Pts',(-1.20138548938974,1.,1.80317454838603));
#26518=CARTESIAN_POINT('Ctrl Pts',(-1.19566418930242,1.,1.80030314369879));
#26519=CARTESIAN_POINT('Ctrl Pts',(-1.18996997934445,1.,1.79740245923478));
#26520=CARTESIAN_POINT('Ctrl Pts',(-1.18430321697432,1.,1.79447240321515));
#26521=CARTESIAN_POINT('Ctrl Pts',(-1.17866429440809,1.,1.79151291552689));
#26522=CARTESIAN_POINT('Ctrl Pts',(-1.17305363177328,1.,1.78852398877616));
#26523=CARTESIAN_POINT('Ctrl Pts',(-1.16747166312303,1.,1.78550566040443));
#26524=CARTESIAN_POINT('Ctrl Pts',(-1.16191881298499,1.,1.78245795881009));
#26525=CARTESIAN_POINT('Ctrl Pts',(-1.15639547194698,1.,1.77938085564275));
#26526=CARTESIAN_POINT('Ctrl Pts',(-1.15090197841515,1.,1.7762742255701));
#26527=CARTESIAN_POINT('Ctrl Pts',(-1.1454385822692,1.,1.77313777896194));
#26528=CARTESIAN_POINT('Ctrl Pts',(-1.14000548336975,1.,1.76997111386769));
#26529=CARTESIAN_POINT('Ctrl Pts',(-1.1346029180462,1.,1.76677384551862));
#26530=CARTESIAN_POINT('Ctrl Pts',(-1.12923123555075,1.,1.7635457196617));
#26531=CARTESIAN_POINT('Ctrl Pts',(-1.12389096855086,1.,1.76028671825096));
#26532=CARTESIAN_POINT('Ctrl Pts',(-1.11858293216763,1.,1.75699720772105));
#26533=CARTESIAN_POINT('Ctrl Pts',(-1.11330807582551,1.,1.7536777209463));
#26534=CARTESIAN_POINT('Ctrl Pts',(-1.10806728183007,1.,1.7503286607592));
#26535=CARTESIAN_POINT('Ctrl Pts',(-1.10286118991143,1.,1.74695004214923));
#26536=CARTESIAN_POINT('Ctrl Pts',(-1.09768999241225,1.,1.74354119236208));
#26537=CARTESIAN_POINT('Ctrl Pts',(-1.09255329056493,1.,1.74010053962247));
#26538=CARTESIAN_POINT('Ctrl Pts',(-1.08745056285427,1.,1.73662628326091));
#26539=CARTESIAN_POINT('Ctrl Pts',(-1.08238162784749,1.,1.73311705663407));
#26540=CARTESIAN_POINT('Ctrl Pts',(-1.0773470373727,1.,1.72957248977424));
#26541=CARTESIAN_POINT('Ctrl Pts',(-1.07234866990252,1.,1.72599406198488));
#26542=CARTESIAN_POINT('Ctrl Pts',(-1.06738966975462,1.,1.72238500928453));
#26543=CARTESIAN_POINT('Ctrl Pts',(-1.06247324680647,1.,1.71874858456904));
#26544=CARTESIAN_POINT('Ctrl Pts',(-1.05760163192479,1.,1.7150865442702));
#26545=CARTESIAN_POINT('Ctrl Pts',(-1.05277517202855,1.,1.71139783543989));
#26546=CARTESIAN_POINT('Ctrl Pts',(-1.04799085404995,1.,1.70767646263649));
#26547=CARTESIAN_POINT('Ctrl Pts',(-1.04324363334554,1.,1.70391338707982));
#26548=CARTESIAN_POINT('Ctrl Pts',(-1.03852922490789,1.,1.70010052930962));
#26549=CARTESIAN_POINT('Ctrl Pts',(-1.03384646003588,1.,1.69623414782771));
#26550=CARTESIAN_POINT('Ctrl Pts',(-1.02919977579147,1.,1.69231840863458));
#26551=CARTESIAN_POINT('Ctrl Pts',(-1.02460180535255,1.,1.68836910178447));
#26552=CARTESIAN_POINT('Ctrl Pts',(-1.02006795074201,1.,1.68440578021706));
#26553=CARTESIAN_POINT('Ctrl Pts',(-1.01561026162773,1.,1.68044289894798));
#26554=CARTESIAN_POINT('Ctrl Pts',(-1.01123236493511,1.,1.67648246776464));
#26555=CARTESIAN_POINT('Ctrl Pts',(-1.00692206696414,1.,1.67250335383293));
#26556=CARTESIAN_POINT('Ctrl Pts',(-1.00265091003727,1.,1.66846059277303));
#26557=CARTESIAN_POINT('Ctrl Pts',(-0.998389654952758,1.,1.66430758030376));
#26558=CARTESIAN_POINT('Ctrl Pts',(-0.994121836661306,1.,1.66001553809947));
#26559=CARTESIAN_POINT('Ctrl Pts',(-0.989855627854165,1.,1.65559044289699));
#26560=CARTESIAN_POINT('Ctrl Pts',(-0.985642622920821,1.,1.65110016612638));
#26561=CARTESIAN_POINT('Ctrl Pts',(-0.981562530939489,1.,1.64665139190656));
#26562=CARTESIAN_POINT('Ctrl Pts',(-0.977689794119416,1.,1.64233990826687));
#26563=CARTESIAN_POINT('Ctrl Pts',(-0.974066058287418,1.,1.63820952658144));
#26564=CARTESIAN_POINT('Ctrl Pts',(-0.970669715997509,1.,1.63420665729798));
#26565=CARTESIAN_POINT('Ctrl Pts',(-0.967387853230345,1.,1.63013849959461));
#26566=CARTESIAN_POINT('Ctrl Pts',(-0.964046107040536,1.,1.62571930670187));
#26567=CARTESIAN_POINT('Ctrl Pts',(-0.960438326101729,1.,1.62061638140221));
#26568=CARTESIAN_POINT('Ctrl Pts',(-0.956354422920671,1.,1.61449324337085));
#26569=CARTESIAN_POINT('Ctrl Pts',(-0.951613284356035,1.,1.60706069896936));
#26570=CARTESIAN_POINT('Ctrl Pts',(-0.946078063315257,1.,1.59810042043673));
#26571=CARTESIAN_POINT('Ctrl Pts',(-0.939646377893399,1.,1.58744937487176));
#26572=CARTESIAN_POINT('Ctrl Pts',(-0.932246680108685,1.,1.57499388382243));
#26573=CARTESIAN_POINT('Ctrl Pts',(-0.923832188944341,1.,1.56065988578893));
#26574=CARTESIAN_POINT('Ctrl Pts',(-0.914375919026456,1.,1.54440491149498));
#26575=CARTESIAN_POINT('Ctrl Pts',(-0.905967409625651,1.,1.52984849887993));
#26576=CARTESIAN_POINT('Ctrl Pts',(-0.899185047483511,1.,1.51805569590094));
#26577=CARTESIAN_POINT('Ctrl Pts',(-0.894452006964543,1.,1.50980486806688));
#26578=CARTESIAN_POINT('Ctrl Pts',(-0.892032620296855,1.,1.5055822144029));
#26579=CARTESIAN_POINT('',(-1.23627494547115,0.,1.81978687191668));
#26580=CARTESIAN_POINT('Origin',(-1.34869019493419,0.,1.73811241238545));
#26581=CARTESIAN_POINT('',(-1.34869019493419,1.,1.73811241238545));
#26582=CARTESIAN_POINT('',(-1.23627494547115,1.,1.81978687191668));
#26583=CARTESIAN_POINT('',(-1.34869019493419,0.,1.73811241238545));
#26584=CARTESIAN_POINT('Ctrl Pts',(-1.15624053661742,-1.,1.31362392696032));
#26585=CARTESIAN_POINT('Ctrl Pts',(-1.15624053661742,1.,1.31362392696032));
#26586=CARTESIAN_POINT('Ctrl Pts',(-1.15950888730809,-1.,1.31722977216397));
#26587=CARTESIAN_POINT('Ctrl Pts',(-1.15950888730809,1.,1.31722977216397));
#26588=CARTESIAN_POINT('Ctrl Pts',(-1.16589330093588,-1.,1.32428080721772));
#26589=CARTESIAN_POINT('Ctrl Pts',(-1.16589330093588,1.,1.32428080721772));
#26590=CARTESIAN_POINT('Ctrl Pts',(-1.17501305789857,-1.,1.33437539347008));
#26591=CARTESIAN_POINT('Ctrl Pts',(-1.17501305789857,1.,1.33437539347008));
#26592=CARTESIAN_POINT('Ctrl Pts',(-1.18625865667441,-1.,1.34687054001093));
#26593=CARTESIAN_POINT('Ctrl Pts',(-1.18625865667441,1.,1.34687054001093));
#26594=CARTESIAN_POINT('Ctrl Pts',(-1.1987959077932,-1.,1.36088705043885));
#26595=CARTESIAN_POINT('Ctrl Pts',(-1.1987959077932,1.,1.36088705043885));
#26596=CARTESIAN_POINT('Ctrl Pts',(-1.20982812925645,-1.,1.37331915607905));
#26597=CARTESIAN_POINT('Ctrl Pts',(-1.20982812925645,1.,1.37331915607905));
#26598=CARTESIAN_POINT('Ctrl Pts',(-1.21938737280852,-1.,1.38420564527715));
#26599=CARTESIAN_POINT('Ctrl Pts',(-1.21938737280852,1.,1.38420564527715));
#26600=CARTESIAN_POINT('Ctrl Pts',(-1.22752961899387,-1.,1.39361389568796));
#26601=CARTESIAN_POINT('Ctrl Pts',(-1.22752961899387,1.,1.39361389568796));
#26602=CARTESIAN_POINT('Ctrl Pts',(-1.23434087290423,-1.,1.40164708206106));
#26603=CARTESIAN_POINT('Ctrl Pts',(-1.23434087290423,1.,1.40164708206106));
#26604=CARTESIAN_POINT('Ctrl Pts',(-1.23994455029534,-1.,1.40845295531283));
#26605=CARTESIAN_POINT('Ctrl Pts',(-1.23994455029534,1.,1.40845295531283));
#26606=CARTESIAN_POINT('Ctrl Pts',(-1.24450600513056,-1.,1.41422913175179));
#26607=CARTESIAN_POINT('Ctrl Pts',(-1.24450600513056,1.,1.41422913175179));
#26608=CARTESIAN_POINT('Ctrl Pts',(-1.24824430986571,-1.,1.41923722596025));
#26609=CARTESIAN_POINT('Ctrl Pts',(-1.24824430986571,1.,1.41923722596025));
#26610=CARTESIAN_POINT('Ctrl Pts',(-1.2514145557001,-1.,1.42378102115575));
#26611=CARTESIAN_POINT('Ctrl Pts',(-1.2514145557001,1.,1.42378102115575));
#26612=CARTESIAN_POINT('Ctrl Pts',(-1.25426945222639,-1.,1.42815938799387));
#26613=CARTESIAN_POINT('Ctrl Pts',(-1.25426945222639,1.,1.42815938799387));
#26614=CARTESIAN_POINT('Ctrl Pts',(-1.25702687965755,-1.,1.43262645609691));
#26615=CARTESIAN_POINT('Ctrl Pts',(-1.25702687965755,1.,1.43262645609691));
#26616=CARTESIAN_POINT('Ctrl Pts',(-1.25983531012005,-1.,1.43734919180848));
#26617=CARTESIAN_POINT('Ctrl Pts',(-1.25983531012005,1.,1.43734919180848));
#26618=CARTESIAN_POINT('Ctrl Pts',(-1.26273903323859,-1.,1.44236470511303));
#26619=CARTESIAN_POINT('Ctrl Pts',(-1.26273903323859,1.,1.44236470511303));
#26620=CARTESIAN_POINT('Ctrl Pts',(-1.26570925118868,-1.,1.44761985001662));
#26621=CARTESIAN_POINT('Ctrl Pts',(-1.26570925118868,1.,1.44761985001662));
#26622=CARTESIAN_POINT('Ctrl Pts',(-1.2686778680489,-1.,1.45301422764247));
#26623=CARTESIAN_POINT('Ctrl Pts',(-1.2686778680489,1.,1.45301422764247));
#26624=CARTESIAN_POINT('Ctrl Pts',(-1.27156805265289,-1.,1.45843906294697));
#26625=CARTESIAN_POINT('Ctrl Pts',(-1.27156805265289,1.,1.45843906294697));
#26626=CARTESIAN_POINT('Ctrl Pts',(-1.27433119897822,-1.,1.46382431332476));
#26627=CARTESIAN_POINT('Ctrl Pts',(-1.27433119897822,1.,1.46382431332476));
#26628=CARTESIAN_POINT('Ctrl Pts',(-1.27696414831089,-1.,1.46916035917133));
#26629=CARTESIAN_POINT('Ctrl Pts',(-1.27696414831089,1.,1.46916035917133));
#26630=CARTESIAN_POINT('Ctrl Pts',(-1.2794891824849,-1.,1.4744717526707));
#26631=CARTESIAN_POINT('Ctrl Pts',(-1.2794891824849,1.,1.4744717526707));
#26632=CARTESIAN_POINT('Ctrl Pts',(-1.28194158939517,-1.,1.47980070347095));
#26633=CARTESIAN_POINT('Ctrl Pts',(-1.28194158939517,1.,1.47980070347095));
#26634=CARTESIAN_POINT('Ctrl Pts',(-1.28435533880201,-1.,1.4851881711891));
#26635=CARTESIAN_POINT('Ctrl Pts',(-1.28435533880201,1.,1.4851881711891));
#26636=CARTESIAN_POINT('Ctrl Pts',(-1.2867467611644,-1.,1.4906522831278));
#26637=CARTESIAN_POINT('Ctrl Pts',(-1.2867467611644,1.,1.4906522831278));
#26638=CARTESIAN_POINT('Ctrl Pts',(-1.28911506584254,-1.,1.49618896881754));
#26639=CARTESIAN_POINT('Ctrl Pts',(-1.28911506584254,1.,1.49618896881754));
#26640=CARTESIAN_POINT('Ctrl Pts',(-1.29145022885181,-1.,1.50178230149776));
#26641=CARTESIAN_POINT('Ctrl Pts',(-1.29145022885181,1.,1.50178230149776));
#26642=CARTESIAN_POINT('Ctrl Pts',(-1.29373841372842,-1.,1.50741159078365));
#26643=CARTESIAN_POINT('Ctrl Pts',(-1.29373841372842,1.,1.50741159078365));
#26644=CARTESIAN_POINT('Ctrl Pts',(-1.29596850710509,-1.,1.51305994241402));
#26645=CARTESIAN_POINT('Ctrl Pts',(-1.29596850710509,1.,1.51305994241402));
#26646=CARTESIAN_POINT('Ctrl Pts',(-1.29813791800747,-1.,1.51872184912724));
#26647=CARTESIAN_POINT('Ctrl Pts',(-1.29813791800747,1.,1.51872184912724));
#26648=CARTESIAN_POINT('Ctrl Pts',(-1.30024984366328,-1.,1.52439957861062));
#26649=CARTESIAN_POINT('Ctrl Pts',(-1.30024984366328,1.,1.52439957861062));
#26650=CARTESIAN_POINT('Ctrl Pts',(-1.30231064395568,-1.,1.53009970283891));
#26651=CARTESIAN_POINT('Ctrl Pts',(-1.30231064395568,1.,1.53009970283891));
#26652=CARTESIAN_POINT('Ctrl Pts',(-1.30432735639489,-1.,1.53582981268977));
#26653=CARTESIAN_POINT('Ctrl Pts',(-1.30432735639489,1.,1.53582981268977));
#26654=CARTESIAN_POINT('Ctrl Pts',(-1.30630475189556,-1.,1.54159462645432));
#26655=CARTESIAN_POINT('Ctrl Pts',(-1.30630475189556,1.,1.54159462645432));
#26656=CARTESIAN_POINT('Ctrl Pts',(-1.30824393907473,-1.,1.54739413957185));
#26657=CARTESIAN_POINT('Ctrl Pts',(-1.30824393907473,1.,1.54739413957185));
#26658=CARTESIAN_POINT('Ctrl Pts',(-1.31014393684222,-1.,1.55322568759481));
#26659=CARTESIAN_POINT('Ctrl Pts',(-1.31014393684222,1.,1.55322568759481));
#26660=CARTESIAN_POINT('Ctrl Pts',(-1.31200264341696,-1.,1.55908521254821));
#26661=CARTESIAN_POINT('Ctrl Pts',(-1.31200264341696,1.,1.55908521254821));
#26662=CARTESIAN_POINT('Ctrl Pts',(-1.31381795281002,-1.,1.56496872402353));
#26663=CARTESIAN_POINT('Ctrl Pts',(-1.31381795281002,1.,1.56496872402353));
#26664=CARTESIAN_POINT('Ctrl Pts',(-1.31558903860016,-1.,1.57087397835723));
#26665=CARTESIAN_POINT('Ctrl Pts',(-1.31558903860016,1.,1.57087397835723));
#26666=CARTESIAN_POINT('Ctrl Pts',(-1.31731642317187,-1.,1.5768005650559));
#26667=CARTESIAN_POINT('Ctrl Pts',(-1.31731642317187,1.,1.5768005650559));
#26668=CARTESIAN_POINT('Ctrl Pts',(-1.31900135021432,-1.,1.58274907898834));
#26669=CARTESIAN_POINT('Ctrl Pts',(-1.31900135021432,1.,1.58274907898834));
#26670=CARTESIAN_POINT('Ctrl Pts',(-1.32064537110892,-1.,1.58872057258245));
#26671=CARTESIAN_POINT('Ctrl Pts',(-1.32064537110892,1.,1.58872057258245));
#26672=CARTESIAN_POINT('Ctrl Pts',(-1.32224985747682,-1.,1.59471591079403));
#26673=CARTESIAN_POINT('Ctrl Pts',(-1.32224985747682,1.,1.59471591079403));
#26674=CARTESIAN_POINT('Ctrl Pts',(-1.32381550858256,-1.,1.60073511858687));
#26675=CARTESIAN_POINT('Ctrl Pts',(-1.32381550858256,1.,1.60073511858687));
#26676=CARTESIAN_POINT('Ctrl Pts',(-1.32534250785782,-1.,1.60677758290954));
#26677=CARTESIAN_POINT('Ctrl Pts',(-1.32534250785782,1.,1.60677758290954));
#26678=CARTESIAN_POINT('Ctrl Pts',(-1.32683074483356,-1.,1.6128423401575));
#26679=CARTESIAN_POINT('Ctrl Pts',(-1.32683074483356,1.,1.6128423401575));
#26680=CARTESIAN_POINT('Ctrl Pts',(-1.32828000610449,-1.,1.61892832270724));
#26681=CARTESIAN_POINT('Ctrl Pts',(-1.32828000610449,1.,1.61892832270724));
#26682=CARTESIAN_POINT('Ctrl Pts',(-1.3296901950568,-1.,1.62503464209797));
#26683=CARTESIAN_POINT('Ctrl Pts',(-1.3296901950568,1.,1.62503464209797));
#26684=CARTESIAN_POINT('Ctrl Pts',(-1.33106149345645,-1.,1.63116079730923));
#26685=CARTESIAN_POINT('Ctrl Pts',(-1.33106149345645,1.,1.63116079730923));
#26686=CARTESIAN_POINT('Ctrl Pts',(-1.33239425103724,-1.,1.63730653475089));
#26687=CARTESIAN_POINT('Ctrl Pts',(-1.33239425103724,1.,1.63730653475089));
#26688=CARTESIAN_POINT('Ctrl Pts',(-1.33368890676572,-1.,1.6434717485603));
#26689=CARTESIAN_POINT('Ctrl Pts',(-1.33368890676572,1.,1.6434717485603));
#26690=CARTESIAN_POINT('Ctrl Pts',(-1.33494590467993,-1.,1.6496563728683));
#26691=CARTESIAN_POINT('Ctrl Pts',(-1.33494590467993,1.,1.6496563728683));
#26692=CARTESIAN_POINT('Ctrl Pts',(-1.33616559745172,-1.,1.65586025952593));
#26693=CARTESIAN_POINT('Ctrl Pts',(-1.33616559745172,1.,1.65586025952593));
#26694=CARTESIAN_POINT('Ctrl Pts',(-1.33734820885262,-1.,1.66208312541983));
#26695=CARTESIAN_POINT('Ctrl Pts',(-1.33734820885262,1.,1.66208312541983));
#26696=CARTESIAN_POINT('Ctrl Pts',(-1.33849388654388,-1.,1.66832460783989));
#26697=CARTESIAN_POINT('Ctrl Pts',(-1.33849388654388,1.,1.66832460783989));
#26698=CARTESIAN_POINT('Ctrl Pts',(-1.3396027347034,-1.,1.67458429426086));
#26699=CARTESIAN_POINT('Ctrl Pts',(-1.3396027347034,1.,1.67458429426086));
#26700=CARTESIAN_POINT('Ctrl Pts',(-1.34067485185203,-1.,1.68086176030362));
#26701=CARTESIAN_POINT('Ctrl Pts',(-1.34067485185203,1.,1.68086176030362));
#26702=CARTESIAN_POINT('Ctrl Pts',(-1.341710374848,-1.,1.68715660868764));
#26703=CARTESIAN_POINT('Ctrl Pts',(-1.341710374848,1.,1.68715660868764));
#26704=CARTESIAN_POINT('Ctrl Pts',(-1.34270948206319,-1.,1.6934684849687));
#26705=CARTESIAN_POINT('Ctrl Pts',(-1.34270948206319,1.,1.6934684849687));
#26706=CARTESIAN_POINT('Ctrl Pts',(-1.34367237124483,-1.,1.69979707754427));
#26707=CARTESIAN_POINT('Ctrl Pts',(-1.34367237124483,1.,1.69979707754427));
#26708=CARTESIAN_POINT('Ctrl Pts',(-1.34459924533831,-1.,1.70614212266738));
#26709=CARTESIAN_POINT('Ctrl Pts',(-1.34459924533831,1.,1.70614212266738));
#26710=CARTESIAN_POINT('Ctrl Pts',(-1.34549029589416,-1.,1.71250340686822));
#26711=CARTESIAN_POINT('Ctrl Pts',(-1.34549029589416,1.,1.71250340686822));
#26712=CARTESIAN_POINT('Ctrl Pts',(-1.34634568653227,-1.,1.7188807715049));
#26713=CARTESIAN_POINT('Ctrl Pts',(-1.34634568653227,1.,1.7188807715049));
#26714=CARTESIAN_POINT('Ctrl Pts',(-1.34716554819527,-1.,1.72527410680674));
#26715=CARTESIAN_POINT('Ctrl Pts',(-1.34716554819527,1.,1.72527410680674));
#26716=CARTESIAN_POINT('Ctrl Pts',(-1.34779309152035,-1.,1.7304014965394));
#26717=CARTESIAN_POINT('Ctrl Pts',(-1.34779309152035,1.,1.7304014965394));
#26718=CARTESIAN_POINT('Ctrl Pts',(-1.34824783112887,-1.,1.73425417885907));
#26719=CARTESIAN_POINT('Ctrl Pts',(-1.34824783112887,1.,1.73425417885907));
#26720=CARTESIAN_POINT('Ctrl Pts',(-1.34854391898045,-1.,1.73682580585691));
#26721=CARTESIAN_POINT('Ctrl Pts',(-1.34854391898045,1.,1.73682580585691));
#26722=CARTESIAN_POINT('Ctrl Pts',(-1.34869019493419,-1.,1.73811241238545));
#26723=CARTESIAN_POINT('Ctrl Pts',(-1.34869019493419,1.,1.73811241238545));
#26724=CARTESIAN_POINT('',(-1.15624053661742,1.,1.31362392696032));
#26725=CARTESIAN_POINT('Ctrl Pts',(-1.15624053661742,1.,1.31362392696032));
#26726=CARTESIAN_POINT('Ctrl Pts',(-1.15950888730809,1.,1.31722977216397));
#26727=CARTESIAN_POINT('Ctrl Pts',(-1.16589330093588,1.,1.32428080721772));
#26728=CARTESIAN_POINT('Ctrl Pts',(-1.17501305789857,1.,1.33437539347008));
#26729=CARTESIAN_POINT('Ctrl Pts',(-1.18625865667441,1.,1.34687054001093));
#26730=CARTESIAN_POINT('Ctrl Pts',(-1.1987959077932,1.,1.36088705043885));
#26731=CARTESIAN_POINT('Ctrl Pts',(-1.20982812925645,1.,1.37331915607905));
#26732=CARTESIAN_POINT('Ctrl Pts',(-1.21938737280852,1.,1.38420564527715));
#26733=CARTESIAN_POINT('Ctrl Pts',(-1.22752961899387,1.,1.39361389568796));
#26734=CARTESIAN_POINT('Ctrl Pts',(-1.23434087290423,1.,1.40164708206106));
#26735=CARTESIAN_POINT('Ctrl Pts',(-1.23994455029534,1.,1.40845295531283));
#26736=CARTESIAN_POINT('Ctrl Pts',(-1.24450600513056,1.,1.41422913175179));
#26737=CARTESIAN_POINT('Ctrl Pts',(-1.24824430986571,1.,1.41923722596025));
#26738=CARTESIAN_POINT('Ctrl Pts',(-1.2514145557001,1.,1.42378102115575));
#26739=CARTESIAN_POINT('Ctrl Pts',(-1.25426945222639,1.,1.42815938799387));
#26740=CARTESIAN_POINT('Ctrl Pts',(-1.25702687965755,1.,1.43262645609691));
#26741=CARTESIAN_POINT('Ctrl Pts',(-1.25983531012005,1.,1.43734919180848));
#26742=CARTESIAN_POINT('Ctrl Pts',(-1.26273903323859,1.,1.44236470511303));
#26743=CARTESIAN_POINT('Ctrl Pts',(-1.26570925118868,1.,1.44761985001662));
#26744=CARTESIAN_POINT('Ctrl Pts',(-1.2686778680489,1.,1.45301422764247));
#26745=CARTESIAN_POINT('Ctrl Pts',(-1.27156805265289,1.,1.45843906294697));
#26746=CARTESIAN_POINT('Ctrl Pts',(-1.27433119897822,1.,1.46382431332476));
#26747=CARTESIAN_POINT('Ctrl Pts',(-1.27696414831089,1.,1.46916035917133));
#26748=CARTESIAN_POINT('Ctrl Pts',(-1.2794891824849,1.,1.4744717526707));
#26749=CARTESIAN_POINT('Ctrl Pts',(-1.28194158939517,1.,1.47980070347095));
#26750=CARTESIAN_POINT('Ctrl Pts',(-1.28435533880201,1.,1.4851881711891));
#26751=CARTESIAN_POINT('Ctrl Pts',(-1.2867467611644,1.,1.4906522831278));
#26752=CARTESIAN_POINT('Ctrl Pts',(-1.28911506584254,1.,1.49618896881754));
#26753=CARTESIAN_POINT('Ctrl Pts',(-1.29145022885181,1.,1.50178230149776));
#26754=CARTESIAN_POINT('Ctrl Pts',(-1.29373841372842,1.,1.50741159078365));
#26755=CARTESIAN_POINT('Ctrl Pts',(-1.29596850710509,1.,1.51305994241402));
#26756=CARTESIAN_POINT('Ctrl Pts',(-1.29813791800747,1.,1.51872184912724));
#26757=CARTESIAN_POINT('Ctrl Pts',(-1.30024984366328,1.,1.52439957861062));
#26758=CARTESIAN_POINT('Ctrl Pts',(-1.30231064395568,1.,1.53009970283891));
#26759=CARTESIAN_POINT('Ctrl Pts',(-1.30432735639489,1.,1.53582981268977));
#26760=CARTESIAN_POINT('Ctrl Pts',(-1.30630475189556,1.,1.54159462645432));
#26761=CARTESIAN_POINT('Ctrl Pts',(-1.30824393907473,1.,1.54739413957185));
#26762=CARTESIAN_POINT('Ctrl Pts',(-1.31014393684222,1.,1.55322568759481));
#26763=CARTESIAN_POINT('Ctrl Pts',(-1.31200264341696,1.,1.55908521254821));
#26764=CARTESIAN_POINT('Ctrl Pts',(-1.31381795281002,1.,1.56496872402353));
#26765=CARTESIAN_POINT('Ctrl Pts',(-1.31558903860016,1.,1.57087397835723));
#26766=CARTESIAN_POINT('Ctrl Pts',(-1.31731642317187,1.,1.5768005650559));
#26767=CARTESIAN_POINT('Ctrl Pts',(-1.31900135021432,1.,1.58274907898834));
#26768=CARTESIAN_POINT('Ctrl Pts',(-1.32064537110892,1.,1.58872057258245));
#26769=CARTESIAN_POINT('Ctrl Pts',(-1.32224985747682,1.,1.59471591079403));
#26770=CARTESIAN_POINT('Ctrl Pts',(-1.32381550858256,1.,1.60073511858687));
#26771=CARTESIAN_POINT('Ctrl Pts',(-1.32534250785782,1.,1.60677758290954));
#26772=CARTESIAN_POINT('Ctrl Pts',(-1.32683074483356,1.,1.6128423401575));
#26773=CARTESIAN_POINT('Ctrl Pts',(-1.32828000610449,1.,1.61892832270724));
#26774=CARTESIAN_POINT('Ctrl Pts',(-1.3296901950568,1.,1.62503464209797));
#26775=CARTESIAN_POINT('Ctrl Pts',(-1.33106149345645,1.,1.63116079730923));
#26776=CARTESIAN_POINT('Ctrl Pts',(-1.33239425103724,1.,1.63730653475089));
#26777=CARTESIAN_POINT('Ctrl Pts',(-1.33368890676572,1.,1.6434717485603));
#26778=CARTESIAN_POINT('Ctrl Pts',(-1.33494590467993,1.,1.6496563728683));
#26779=CARTESIAN_POINT('Ctrl Pts',(-1.33616559745172,1.,1.65586025952593));
#26780=CARTESIAN_POINT('Ctrl Pts',(-1.33734820885262,1.,1.66208312541983));
#26781=CARTESIAN_POINT('Ctrl Pts',(-1.33849388654388,1.,1.66832460783989));
#26782=CARTESIAN_POINT('Ctrl Pts',(-1.3396027347034,1.,1.67458429426086));
#26783=CARTESIAN_POINT('Ctrl Pts',(-1.34067485185203,1.,1.68086176030362));
#26784=CARTESIAN_POINT('Ctrl Pts',(-1.341710374848,1.,1.68715660868764));
#26785=CARTESIAN_POINT('Ctrl Pts',(-1.34270948206319,1.,1.6934684849687));
#26786=CARTESIAN_POINT('Ctrl Pts',(-1.34367237124483,1.,1.69979707754427));
#26787=CARTESIAN_POINT('Ctrl Pts',(-1.34459924533831,1.,1.70614212266738));
#26788=CARTESIAN_POINT('Ctrl Pts',(-1.34549029589416,1.,1.71250340686822));
#26789=CARTESIAN_POINT('Ctrl Pts',(-1.34634568653227,1.,1.7188807715049));
#26790=CARTESIAN_POINT('Ctrl Pts',(-1.34716554819527,1.,1.72527410680674));
#26791=CARTESIAN_POINT('Ctrl Pts',(-1.34779309152035,1.,1.7304014965394));
#26792=CARTESIAN_POINT('Ctrl Pts',(-1.34824783112887,1.,1.73425417885907));
#26793=CARTESIAN_POINT('Ctrl Pts',(-1.34854391898045,1.,1.73682580585691));
#26794=CARTESIAN_POINT('Ctrl Pts',(-1.34869019493419,1.,1.73811241238545));
#26795=CARTESIAN_POINT('',(-1.15624053661742,0.,1.31362392696032));
#26796=CARTESIAN_POINT('Origin',(0.,0.,0.));
#26797=CARTESIAN_POINT('',(-1.31362392696033,1.,1.15624053661742));
#26798=CARTESIAN_POINT('Origin',(0.,1.,0.));
#26799=CARTESIAN_POINT('',(-1.31362392696033,0.,1.15624053661742));
#26800=CARTESIAN_POINT('Ctrl Pts',(-1.73811241238545,-1.,1.34869019493419));
#26801=CARTESIAN_POINT('Ctrl Pts',(-1.73811241238545,1.,1.34869019493419));
#26802=CARTESIAN_POINT('Ctrl Pts',(-1.73682580585819,-1.,1.34854391898145));
#26803=CARTESIAN_POINT('Ctrl Pts',(-1.73682580585819,1.,1.34854391898145));
#26804=CARTESIAN_POINT('Ctrl Pts',(-1.73425417886255,-1.,1.34824783113158));
#26805=CARTESIAN_POINT('Ctrl Pts',(-1.73425417886255,1.,1.34824783113158));
#26806=CARTESIAN_POINT('Ctrl Pts',(-1.73040149654497,-1.,1.3477930915247));
#26807=CARTESIAN_POINT('Ctrl Pts',(-1.73040149654497,1.,1.3477930915247));
#26808=CARTESIAN_POINT('Ctrl Pts',(-1.72527410681298,-1.,1.34716554820013));
#26809=CARTESIAN_POINT('Ctrl Pts',(-1.72527410681298,1.,1.34716554820013));
#26810=CARTESIAN_POINT('Ctrl Pts',(-1.7188807715095,-1.,1.34634568653586));
#26811=CARTESIAN_POINT('Ctrl Pts',(-1.7188807715095,1.,1.34634568653586));
#26812=CARTESIAN_POINT('Ctrl Pts',(-1.71250340687011,-1.,1.34549029589563));
#26813=CARTESIAN_POINT('Ctrl Pts',(-1.71250340687011,1.,1.34549029589563));
#26814=CARTESIAN_POINT('Ctrl Pts',(-1.70614212266676,-1.,1.34459924533783));
#26815=CARTESIAN_POINT('Ctrl Pts',(-1.70614212266676,1.,1.34459924533783));
#26816=CARTESIAN_POINT('Ctrl Pts',(-1.69979707754221,-1.,1.34367237124322));
#26817=CARTESIAN_POINT('Ctrl Pts',(-1.69979707754221,1.,1.34367237124322));
#26818=CARTESIAN_POINT('Ctrl Pts',(-1.6934684849664,-1.,1.34270948206139));
#26819=CARTESIAN_POINT('Ctrl Pts',(-1.6934684849664,1.,1.34270948206139));
#26820=CARTESIAN_POINT('Ctrl Pts',(-1.68715660868602,-1.,1.34171037484673));
#26821=CARTESIAN_POINT('Ctrl Pts',(-1.68715660868602,1.,1.34171037484673));
#26822=CARTESIAN_POINT('Ctrl Pts',(-1.68086176030308,-1.,1.3406748518516));
#26823=CARTESIAN_POINT('Ctrl Pts',(-1.68086176030308,1.,1.3406748518516));
#26824=CARTESIAN_POINT('Ctrl Pts',(-1.67458429426126,-1.,1.33960273470372));
#26825=CARTESIAN_POINT('Ctrl Pts',(-1.67458429426126,1.,1.33960273470372));
#26826=CARTESIAN_POINT('Ctrl Pts',(-1.66832460784078,-1.,1.33849388654458));
#26827=CARTESIAN_POINT('Ctrl Pts',(-1.66832460784078,1.,1.33849388654458));
#26828=CARTESIAN_POINT('Ctrl Pts',(-1.66208312542073,-1.,1.33734820885331));
#26829=CARTESIAN_POINT('Ctrl Pts',(-1.66208312542073,1.,1.33734820885331));
#26830=CARTESIAN_POINT('Ctrl Pts',(-1.65586025952651,-1.,1.33616559745217));
#26831=CARTESIAN_POINT('Ctrl Pts',(-1.65586025952651,1.,1.33616559745217));
#26832=CARTESIAN_POINT('Ctrl Pts',(-1.64965637286843,-1.,1.33494590468003));
#26833=CARTESIAN_POINT('Ctrl Pts',(-1.64965637286843,1.,1.33494590468003));
#26834=CARTESIAN_POINT('Ctrl Pts',(-1.64347174856007,-1.,1.33368890676554));
#26835=CARTESIAN_POINT('Ctrl Pts',(-1.64347174856007,1.,1.33368890676554));
#26836=CARTESIAN_POINT('Ctrl Pts',(-1.6373065347505,-1.,1.33239425103694));
#26837=CARTESIAN_POINT('Ctrl Pts',(-1.6373065347505,1.,1.33239425103694));
#26838=CARTESIAN_POINT('Ctrl Pts',(-1.63116079730887,-1.,1.33106149345618));
#26839=CARTESIAN_POINT('Ctrl Pts',(-1.63116079730887,1.,1.33106149345618));
#26840=CARTESIAN_POINT('Ctrl Pts',(-1.62503464209777,-1.,1.32969019505665));
#26841=CARTESIAN_POINT('Ctrl Pts',(-1.62503464209777,1.,1.32969019505665));
#26842=CARTESIAN_POINT('Ctrl Pts',(-1.61892832270723,-1.,1.32828000610448));
#26843=CARTESIAN_POINT('Ctrl Pts',(-1.61892832270723,1.,1.32828000610448));
#26844=CARTESIAN_POINT('Ctrl Pts',(-1.61284234015762,-1.,1.32683074483365));
#26845=CARTESIAN_POINT('Ctrl Pts',(-1.61284234015762,1.,1.32683074483365));
#26846=CARTESIAN_POINT('Ctrl Pts',(-1.6067775829097,-1.,1.32534250785794));
#26847=CARTESIAN_POINT('Ctrl Pts',(-1.6067775829097,1.,1.32534250785794));
#26848=CARTESIAN_POINT('Ctrl Pts',(-1.600735118587,-1.,1.32381550858266));
#26849=CARTESIAN_POINT('Ctrl Pts',(-1.600735118587,1.,1.32381550858266));
#26850=CARTESIAN_POINT('Ctrl Pts',(-1.59471591079408,-1.,1.32224985747686));
#26851=CARTESIAN_POINT('Ctrl Pts',(-1.59471591079408,1.,1.32224985747686));
#26852=CARTESIAN_POINT('Ctrl Pts',(-1.58872057258244,-1.,1.32064537110891));
#26853=CARTESIAN_POINT('Ctrl Pts',(-1.58872057258244,1.,1.32064537110891));
#26854=CARTESIAN_POINT('Ctrl Pts',(-1.58274907898829,-1.,1.31900135021428));
#26855=CARTESIAN_POINT('Ctrl Pts',(-1.58274907898829,1.,1.31900135021428));
#26856=CARTESIAN_POINT('Ctrl Pts',(-1.57680056505585,-1.,1.31731642317183));
#26857=CARTESIAN_POINT('Ctrl Pts',(-1.57680056505585,1.,1.31731642317183));
#26858=CARTESIAN_POINT('Ctrl Pts',(-1.57087397835721,-1.,1.31558903860015));
#26859=CARTESIAN_POINT('Ctrl Pts',(-1.57087397835721,1.,1.31558903860015));
#26860=CARTESIAN_POINT('Ctrl Pts',(-1.56496872402352,-1.,1.31381795281002));
#26861=CARTESIAN_POINT('Ctrl Pts',(-1.56496872402352,1.,1.31381795281002));
#26862=CARTESIAN_POINT('Ctrl Pts',(-1.55908521254822,-1.,1.31200264341696));
#26863=CARTESIAN_POINT('Ctrl Pts',(-1.55908521254822,1.,1.31200264341696));
#26864=CARTESIAN_POINT('Ctrl Pts',(-1.55322568759481,-1.,1.31014393684221));
#26865=CARTESIAN_POINT('Ctrl Pts',(-1.55322568759481,1.,1.31014393684221));
#26866=CARTESIAN_POINT('Ctrl Pts',(-1.54739413957183,-1.,1.30824393907471));
#26867=CARTESIAN_POINT('Ctrl Pts',(-1.54739413957183,1.,1.30824393907471));
#26868=CARTESIAN_POINT('Ctrl Pts',(-1.54159462645428,-1.,1.30630475189553));
#26869=CARTESIAN_POINT('Ctrl Pts',(-1.54159462645428,1.,1.30630475189553));
#26870=CARTESIAN_POINT('Ctrl Pts',(-1.53582981268976,-1.,1.30432735639487));
#26871=CARTESIAN_POINT('Ctrl Pts',(-1.53582981268976,1.,1.30432735639487));
#26872=CARTESIAN_POINT('Ctrl Pts',(-1.53009970283893,-1.,1.3023106439557));
#26873=CARTESIAN_POINT('Ctrl Pts',(-1.53009970283893,1.,1.3023106439557));
#26874=CARTESIAN_POINT('Ctrl Pts',(-1.5243995786107,-1.,1.30024984366334));
#26875=CARTESIAN_POINT('Ctrl Pts',(-1.5243995786107,1.,1.30024984366334));
#26876=CARTESIAN_POINT('Ctrl Pts',(-1.51872184912735,-1.,1.29813791800757));
#26877=CARTESIAN_POINT('Ctrl Pts',(-1.51872184912735,1.,1.29813791800757));
#26878=CARTESIAN_POINT('Ctrl Pts',(-1.51305994241412,-1.,1.29596850710518));
#26879=CARTESIAN_POINT('Ctrl Pts',(-1.51305994241412,1.,1.29596850710518));
#26880=CARTESIAN_POINT('Ctrl Pts',(-1.50741159078367,-1.,1.29373841372843));
#26881=CARTESIAN_POINT('Ctrl Pts',(-1.50741159078367,1.,1.29373841372843));
#26882=CARTESIAN_POINT('Ctrl Pts',(-1.50178230149764,-1.,1.29145022885171));
#26883=CARTESIAN_POINT('Ctrl Pts',(-1.50178230149764,1.,1.29145022885171));
#26884=CARTESIAN_POINT('Ctrl Pts',(-1.49618896881729,-1.,1.28911506584232));
#26885=CARTESIAN_POINT('Ctrl Pts',(-1.49618896881729,1.,1.28911506584232));
#26886=CARTESIAN_POINT('Ctrl Pts',(-1.4906522831275,-1.,1.28674676116415));
#26887=CARTESIAN_POINT('Ctrl Pts',(-1.4906522831275,1.,1.28674676116415));
#26888=CARTESIAN_POINT('Ctrl Pts',(-1.48518817118891,-1.,1.28435533880184));
#26889=CARTESIAN_POINT('Ctrl Pts',(-1.48518817118891,1.,1.28435533880184));
#26890=CARTESIAN_POINT('Ctrl Pts',(-1.47980070347102,-1.,1.28194158939522));
#26891=CARTESIAN_POINT('Ctrl Pts',(-1.47980070347102,1.,1.28194158939522));
#26892=CARTESIAN_POINT('Ctrl Pts',(-1.4744717526711,-1.,1.27948918248524));
#26893=CARTESIAN_POINT('Ctrl Pts',(-1.4744717526711,1.,1.27948918248524));
#26894=CARTESIAN_POINT('Ctrl Pts',(-1.46916035917197,-1.,1.27696414831144));
#26895=CARTESIAN_POINT('Ctrl Pts',(-1.46916035917197,1.,1.27696414831144));
#26896=CARTESIAN_POINT('Ctrl Pts',(-1.4638243133254,-1.,1.27433119897877));
#26897=CARTESIAN_POINT('Ctrl Pts',(-1.4638243133254,1.,1.27433119897877));
#26898=CARTESIAN_POINT('Ctrl Pts',(-1.45843906294725,-1.,1.27156805265312));
#26899=CARTESIAN_POINT('Ctrl Pts',(-1.45843906294725,1.,1.27156805265312));
#26900=CARTESIAN_POINT('Ctrl Pts',(-1.45301422764205,-1.,1.26867786804854));
#26901=CARTESIAN_POINT('Ctrl Pts',(-1.45301422764205,1.,1.26867786804854));
#26902=CARTESIAN_POINT('Ctrl Pts',(-1.44761985001544,-1.,1.26570925118767));
#26903=CARTESIAN_POINT('Ctrl Pts',(-1.44761985001544,1.,1.26570925118767));
#26904=CARTESIAN_POINT('Ctrl Pts',(-1.44236470511145,-1.,1.26273903323723));
#26905=CARTESIAN_POINT('Ctrl Pts',(-1.44236470511145,1.,1.26273903323723));
#26906=CARTESIAN_POINT('Ctrl Pts',(-1.43734919180719,-1.,1.25983531011894));
#26907=CARTESIAN_POINT('Ctrl Pts',(-1.43734919180719,1.,1.25983531011894));
#26908=CARTESIAN_POINT('Ctrl Pts',(-1.43262645609679,-1.,1.25702687965744));
#26909=CARTESIAN_POINT('Ctrl Pts',(-1.43262645609679,1.,1.25702687965744));
#26910=CARTESIAN_POINT('Ctrl Pts',(-1.42815938799555,-1.,1.25426945222783));
#26911=CARTESIAN_POINT('Ctrl Pts',(-1.42815938799555,1.,1.25426945222783));
#26912=CARTESIAN_POINT('Ctrl Pts',(-1.42378102115911,-1.,1.25141455570299));
#26913=CARTESIAN_POINT('Ctrl Pts',(-1.42378102115911,1.,1.25141455570299));
#26914=CARTESIAN_POINT('Ctrl Pts',(-1.41923722596421,-1.,1.24824430986911));
#26915=CARTESIAN_POINT('Ctrl Pts',(-1.41923722596421,1.,1.24824430986911));
#26916=CARTESIAN_POINT('Ctrl Pts',(-1.41422913175437,-1.,1.24450600513278));
#26917=CARTESIAN_POINT('Ctrl Pts',(-1.41422913175437,1.,1.24450600513278));
#26918=CARTESIAN_POINT('Ctrl Pts',(-1.40845295531151,-1.,1.23994455029421));
#26919=CARTESIAN_POINT('Ctrl Pts',(-1.40845295531151,1.,1.23994455029421));
#26920=CARTESIAN_POINT('Ctrl Pts',(-1.40164708205345,-1.,1.23434087289768));
#26921=CARTESIAN_POINT('Ctrl Pts',(-1.40164708205345,1.,1.23434087289768));
#26922=CARTESIAN_POINT('Ctrl Pts',(-1.39361389567257,-1.,1.22752961898063));
#26923=CARTESIAN_POINT('Ctrl Pts',(-1.39361389567257,1.,1.22752961898063));
#26924=CARTESIAN_POINT('Ctrl Pts',(-1.38420564525391,-1.,1.21938737278853));
#26925=CARTESIAN_POINT('Ctrl Pts',(-1.38420564525391,1.,1.21938737278853));
#26926=CARTESIAN_POINT('Ctrl Pts',(-1.37331915604962,-1.,1.20982812923113));
#26927=CARTESIAN_POINT('Ctrl Pts',(-1.37331915604962,1.,1.20982812923113));
#26928=CARTESIAN_POINT('Ctrl Pts',(-1.36088705040677,-1.,1.1987959077656));
#26929=CARTESIAN_POINT('Ctrl Pts',(-1.36088705040677,1.,1.1987959077656));
#26930=CARTESIAN_POINT('Ctrl Pts',(-1.34687053998157,-1.,1.18625865664915));
#26931=CARTESIAN_POINT('Ctrl Pts',(-1.34687053998157,1.,1.18625865664915));
#26932=CARTESIAN_POINT('Ctrl Pts',(-1.33437539344842,-1.,1.17501305787994));
#26933=CARTESIAN_POINT('Ctrl Pts',(-1.33437539344842,1.,1.17501305787994));
#26934=CARTESIAN_POINT('Ctrl Pts',(-1.32428080720544,-1.,1.16589330092532));
#26935=CARTESIAN_POINT('Ctrl Pts',(-1.32428080720544,1.,1.16589330092532));
#26936=CARTESIAN_POINT('Ctrl Pts',(-1.3172297721596,-1.,1.15950888730433));
#26937=CARTESIAN_POINT('Ctrl Pts',(-1.3172297721596,1.,1.15950888730433));
#26938=CARTESIAN_POINT('Ctrl Pts',(-1.31362392696033,-1.,1.15624053661742));
#26939=CARTESIAN_POINT('Ctrl Pts',(-1.31362392696033,1.,1.15624053661742));
#26940=CARTESIAN_POINT('',(-1.73811241238545,1.,1.34869019493419));
#26941=CARTESIAN_POINT('Ctrl Pts',(-1.73811241238545,1.,1.34869019493419));
#26942=CARTESIAN_POINT('Ctrl Pts',(-1.73682580585819,1.,1.34854391898145));
#26943=CARTESIAN_POINT('Ctrl Pts',(-1.73425417886255,1.,1.34824783113158));
#26944=CARTESIAN_POINT('Ctrl Pts',(-1.73040149654497,1.,1.3477930915247));
#26945=CARTESIAN_POINT('Ctrl Pts',(-1.72527410681298,1.,1.34716554820013));
#26946=CARTESIAN_POINT('Ctrl Pts',(-1.7188807715095,1.,1.34634568653586));
#26947=CARTESIAN_POINT('Ctrl Pts',(-1.71250340687011,1.,1.34549029589563));
#26948=CARTESIAN_POINT('Ctrl Pts',(-1.70614212266676,1.,1.34459924533783));
#26949=CARTESIAN_POINT('Ctrl Pts',(-1.69979707754221,1.,1.34367237124322));
#26950=CARTESIAN_POINT('Ctrl Pts',(-1.6934684849664,1.,1.34270948206139));
#26951=CARTESIAN_POINT('Ctrl Pts',(-1.68715660868602,1.,1.34171037484673));
#26952=CARTESIAN_POINT('Ctrl Pts',(-1.68086176030308,1.,1.3406748518516));
#26953=CARTESIAN_POINT('Ctrl Pts',(-1.67458429426126,1.,1.33960273470372));
#26954=CARTESIAN_POINT('Ctrl Pts',(-1.66832460784078,1.,1.33849388654458));
#26955=CARTESIAN_POINT('Ctrl Pts',(-1.66208312542073,1.,1.33734820885331));
#26956=CARTESIAN_POINT('Ctrl Pts',(-1.65586025952651,1.,1.33616559745217));
#26957=CARTESIAN_POINT('Ctrl Pts',(-1.64965637286843,1.,1.33494590468003));
#26958=CARTESIAN_POINT('Ctrl Pts',(-1.64347174856007,1.,1.33368890676554));
#26959=CARTESIAN_POINT('Ctrl Pts',(-1.6373065347505,1.,1.33239425103694));
#26960=CARTESIAN_POINT('Ctrl Pts',(-1.63116079730887,1.,1.33106149345618));
#26961=CARTESIAN_POINT('Ctrl Pts',(-1.62503464209777,1.,1.32969019505665));
#26962=CARTESIAN_POINT('Ctrl Pts',(-1.61892832270723,1.,1.32828000610448));
#26963=CARTESIAN_POINT('Ctrl Pts',(-1.61284234015762,1.,1.32683074483365));
#26964=CARTESIAN_POINT('Ctrl Pts',(-1.6067775829097,1.,1.32534250785794));
#26965=CARTESIAN_POINT('Ctrl Pts',(-1.600735118587,1.,1.32381550858266));
#26966=CARTESIAN_POINT('Ctrl Pts',(-1.59471591079408,1.,1.32224985747686));
#26967=CARTESIAN_POINT('Ctrl Pts',(-1.58872057258244,1.,1.32064537110891));
#26968=CARTESIAN_POINT('Ctrl Pts',(-1.58274907898829,1.,1.31900135021428));
#26969=CARTESIAN_POINT('Ctrl Pts',(-1.57680056505585,1.,1.31731642317183));
#26970=CARTESIAN_POINT('Ctrl Pts',(-1.57087397835721,1.,1.31558903860015));
#26971=CARTESIAN_POINT('Ctrl Pts',(-1.56496872402352,1.,1.31381795281002));
#26972=CARTESIAN_POINT('Ctrl Pts',(-1.55908521254822,1.,1.31200264341696));
#26973=CARTESIAN_POINT('Ctrl Pts',(-1.55322568759481,1.,1.31014393684221));
#26974=CARTESIAN_POINT('Ctrl Pts',(-1.54739413957183,1.,1.30824393907471));
#26975=CARTESIAN_POINT('Ctrl Pts',(-1.54159462645428,1.,1.30630475189553));
#26976=CARTESIAN_POINT('Ctrl Pts',(-1.53582981268976,1.,1.30432735639487));
#26977=CARTESIAN_POINT('Ctrl Pts',(-1.53009970283893,1.,1.3023106439557));
#26978=CARTESIAN_POINT('Ctrl Pts',(-1.5243995786107,1.,1.30024984366334));
#26979=CARTESIAN_POINT('Ctrl Pts',(-1.51872184912735,1.,1.29813791800757));
#26980=CARTESIAN_POINT('Ctrl Pts',(-1.51305994241412,1.,1.29596850710518));
#26981=CARTESIAN_POINT('Ctrl Pts',(-1.50741159078367,1.,1.29373841372843));
#26982=CARTESIAN_POINT('Ctrl Pts',(-1.50178230149764,1.,1.29145022885171));
#26983=CARTESIAN_POINT('Ctrl Pts',(-1.49618896881729,1.,1.28911506584232));
#26984=CARTESIAN_POINT('Ctrl Pts',(-1.4906522831275,1.,1.28674676116415));
#26985=CARTESIAN_POINT('Ctrl Pts',(-1.48518817118891,1.,1.28435533880184));
#26986=CARTESIAN_POINT('Ctrl Pts',(-1.47980070347102,1.,1.28194158939522));
#26987=CARTESIAN_POINT('Ctrl Pts',(-1.4744717526711,1.,1.27948918248524));
#26988=CARTESIAN_POINT('Ctrl Pts',(-1.46916035917197,1.,1.27696414831144));
#26989=CARTESIAN_POINT('Ctrl Pts',(-1.4638243133254,1.,1.27433119897877));
#26990=CARTESIAN_POINT('Ctrl Pts',(-1.45843906294725,1.,1.27156805265312));
#26991=CARTESIAN_POINT('Ctrl Pts',(-1.45301422764205,1.,1.26867786804854));
#26992=CARTESIAN_POINT('Ctrl Pts',(-1.44761985001544,1.,1.26570925118767));
#26993=CARTESIAN_POINT('Ctrl Pts',(-1.44236470511145,1.,1.26273903323723));
#26994=CARTESIAN_POINT('Ctrl Pts',(-1.43734919180719,1.,1.25983531011894));
#26995=CARTESIAN_POINT('Ctrl Pts',(-1.43262645609679,1.,1.25702687965744));
#26996=CARTESIAN_POINT('Ctrl Pts',(-1.42815938799555,1.,1.25426945222783));
#26997=CARTESIAN_POINT('Ctrl Pts',(-1.42378102115911,1.,1.25141455570299));
#26998=CARTESIAN_POINT('Ctrl Pts',(-1.41923722596421,1.,1.24824430986911));
#26999=CARTESIAN_POINT('Ctrl Pts',(-1.41422913175437,1.,1.24450600513278));
#27000=CARTESIAN_POINT('Ctrl Pts',(-1.40845295531151,1.,1.23994455029421));
#27001=CARTESIAN_POINT('Ctrl Pts',(-1.40164708205345,1.,1.23434087289768));
#27002=CARTESIAN_POINT('Ctrl Pts',(-1.39361389567257,1.,1.22752961898063));
#27003=CARTESIAN_POINT('Ctrl Pts',(-1.38420564525391,1.,1.21938737278853));
#27004=CARTESIAN_POINT('Ctrl Pts',(-1.37331915604962,1.,1.20982812923113));
#27005=CARTESIAN_POINT('Ctrl Pts',(-1.36088705040677,1.,1.1987959077656));
#27006=CARTESIAN_POINT('Ctrl Pts',(-1.34687053998157,1.,1.18625865664915));
#27007=CARTESIAN_POINT('Ctrl Pts',(-1.33437539344842,1.,1.17501305787994));
#27008=CARTESIAN_POINT('Ctrl Pts',(-1.32428080720544,1.,1.16589330092532));
#27009=CARTESIAN_POINT('Ctrl Pts',(-1.3172297721596,1.,1.15950888730433));
#27010=CARTESIAN_POINT('Ctrl Pts',(-1.31362392696033,1.,1.15624053661742));
#27011=CARTESIAN_POINT('',(-1.73811241238545,0.,1.34869019493419));
#27012=CARTESIAN_POINT('Origin',(-1.81978687191668,0.,1.23627494547115));
#27013=CARTESIAN_POINT('',(-1.81978687191668,1.,1.23627494547115));
#27014=CARTESIAN_POINT('',(-1.73811241238545,1.,1.34869019493419));
#27015=CARTESIAN_POINT('',(-1.81978687191668,0.,1.23627494547115));
#27016=CARTESIAN_POINT('Ctrl Pts',(-1.5055822144029,-1.,0.892032620296855));
#27017=CARTESIAN_POINT('Ctrl Pts',(-1.5055822144029,1.,0.892032620296855));
#27018=CARTESIAN_POINT('Ctrl Pts',(-1.50980486807181,-1.,0.894452006967538));
#27019=CARTESIAN_POINT('Ctrl Pts',(-1.50980486807181,1.,0.894452006967538));
#27020=CARTESIAN_POINT('Ctrl Pts',(-1.51805569591479,-1.,0.89918504749193));
#27021=CARTESIAN_POINT('Ctrl Pts',(-1.51805569591479,1.,0.89918504749193));
#27022=CARTESIAN_POINT('Ctrl Pts',(-1.52984849890434,-1.,0.905967409640499));
#27023=CARTESIAN_POINT('Ctrl Pts',(-1.52984849890434,1.,0.905967409640499));
#27024=CARTESIAN_POINT('Ctrl Pts',(-1.54440491152808,-1.,0.91437591904658));
#27025=CARTESIAN_POINT('Ctrl Pts',(-1.54440491152808,1.,0.91437591904658));
#27026=CARTESIAN_POINT('Ctrl Pts',(-1.56065988582509,-1.,0.923832188966322));
#27027=CARTESIAN_POINT('Ctrl Pts',(-1.56065988582509,1.,0.923832188966322));
#27028=CARTESIAN_POINT('Ctrl Pts',(-1.57499388385561,-1.,0.932246680128849));
#27029=CARTESIAN_POINT('Ctrl Pts',(-1.57499388385561,1.,0.932246680128849));
#27030=CARTESIAN_POINT('Ctrl Pts',(-1.58744937489796,-1.,0.939646377909319));
#27031=CARTESIAN_POINT('Ctrl Pts',(-1.58744937489796,1.,0.939646377909319));
#27032=CARTESIAN_POINT('Ctrl Pts',(-1.59810042045408,-1.,0.946078063325796));
#27033=CARTESIAN_POINT('Ctrl Pts',(-1.59810042045408,1.,0.946078063325796));
#27034=CARTESIAN_POINT('Ctrl Pts',(-1.60706069897794,-1.,0.951613284361248));
#27035=CARTESIAN_POINT('Ctrl Pts',(-1.60706069897794,1.,0.951613284361248));
#27036=CARTESIAN_POINT('Ctrl Pts',(-1.61449324337233,-1.,0.956354422921573));
#27037=CARTESIAN_POINT('Ctrl Pts',(-1.61449324337233,1.,0.956354422921573));
#27038=CARTESIAN_POINT('Ctrl Pts',(-1.62061638139929,-1.,0.960438326099958));
#27039=CARTESIAN_POINT('Ctrl Pts',(-1.62061638139929,1.,0.960438326099958));
#27040=CARTESIAN_POINT('Ctrl Pts',(-1.6257193066974,-1.,0.964046107037821));
#27041=CARTESIAN_POINT('Ctrl Pts',(-1.6257193066974,1.,0.964046107037821));
#27042=CARTESIAN_POINT('Ctrl Pts',(-1.63013849959083,-1.,0.967387853228041));
#27043=CARTESIAN_POINT('Ctrl Pts',(-1.63013849959083,1.,0.967387853228041));
#27044=CARTESIAN_POINT('Ctrl Pts',(-1.63420665729609,-1.,0.970669715996356));
#27045=CARTESIAN_POINT('Ctrl Pts',(-1.63420665729609,1.,0.970669715996356));
#27046=CARTESIAN_POINT('Ctrl Pts',(-1.63820952658157,-1.,0.974066058287501));
#27047=CARTESIAN_POINT('Ctrl Pts',(-1.63820952658157,1.,0.974066058287501));
#27048=CARTESIAN_POINT('Ctrl Pts',(-1.64233990826831,-1.,0.977689794120297));
#27049=CARTESIAN_POINT('Ctrl Pts',(-1.64233990826831,1.,0.977689794120297));
#27050=CARTESIAN_POINT('Ctrl Pts',(-1.64665139190834,-1.,0.981562530940574));
#27051=CARTESIAN_POINT('Ctrl Pts',(-1.64665139190834,1.,0.981562530940574));
#27052=CARTESIAN_POINT('Ctrl Pts',(-1.6511001661277,-1.,0.985642622921626));
#27053=CARTESIAN_POINT('Ctrl Pts',(-1.6511001661277,1.,0.985642622921626));
#27054=CARTESIAN_POINT('Ctrl Pts',(-1.65559044289746,-1.,0.98985562785445));
#27055=CARTESIAN_POINT('Ctrl Pts',(-1.65559044289746,1.,0.98985562785445));
#27056=CARTESIAN_POINT('Ctrl Pts',(-1.66001553809916,-1.,0.994121836661116));
#27057=CARTESIAN_POINT('Ctrl Pts',(-1.66001553809916,1.,0.994121836661116));
#27058=CARTESIAN_POINT('Ctrl Pts',(-1.66430758030304,-1.,0.998389654952317));
#27059=CARTESIAN_POINT('Ctrl Pts',(-1.66430758030304,1.,0.998389654952317));
#27060=CARTESIAN_POINT('Ctrl Pts',(-1.66846059277231,-1.,1.00265091003682));
#27061=CARTESIAN_POINT('Ctrl Pts',(-1.66846059277231,1.,1.00265091003682));
#27062=CARTESIAN_POINT('Ctrl Pts',(-1.67250335383248,-1.,1.00692206696387));
#27063=CARTESIAN_POINT('Ctrl Pts',(-1.67250335383248,1.,1.00692206696387));
#27064=CARTESIAN_POINT('Ctrl Pts',(-1.67648246776457,-1.,1.01123236493507));
#27065=CARTESIAN_POINT('Ctrl Pts',(-1.67648246776457,1.,1.01123236493507));
#27066=CARTESIAN_POINT('Ctrl Pts',(-1.6804428989482,-1.,1.01561026162787));
#27067=CARTESIAN_POINT('Ctrl Pts',(-1.6804428989482,1.,1.01561026162787));
#27068=CARTESIAN_POINT('Ctrl Pts',(-1.68440578021739,-1.,1.02006795074222));
#27069=CARTESIAN_POINT('Ctrl Pts',(-1.68440578021739,1.,1.02006795074222));
#27070=CARTESIAN_POINT('Ctrl Pts',(-1.68836910178475,-1.,1.02460180535272));
#27071=CARTESIAN_POINT('Ctrl Pts',(-1.68836910178475,1.,1.02460180535272));
#27072=CARTESIAN_POINT('Ctrl Pts',(-1.69231840863471,-1.,1.02919977579155));
#27073=CARTESIAN_POINT('Ctrl Pts',(-1.69231840863471,1.,1.02919977579155));
#27074=CARTESIAN_POINT('Ctrl Pts',(-1.69623414782769,-1.,1.03384646003587));
#27075=CARTESIAN_POINT('Ctrl Pts',(-1.69623414782769,1.,1.03384646003587));
#27076=CARTESIAN_POINT('Ctrl Pts',(-1.70010052930951,-1.,1.03852922490782));
#27077=CARTESIAN_POINT('Ctrl Pts',(-1.70010052930951,1.,1.03852922490782));
#27078=CARTESIAN_POINT('Ctrl Pts',(-1.70391338707969,-1.,1.04324363334546));
#27079=CARTESIAN_POINT('Ctrl Pts',(-1.70391338707969,1.,1.04324363334546));
#27080=CARTESIAN_POINT('Ctrl Pts',(-1.70767646263641,-1.,1.0479908540499));
#27081=CARTESIAN_POINT('Ctrl Pts',(-1.70767646263641,1.,1.0479908540499));
#27082=CARTESIAN_POINT('Ctrl Pts',(-1.71139783543986,-1.,1.05277517202854));
#27083=CARTESIAN_POINT('Ctrl Pts',(-1.71139783543986,1.,1.05277517202854));
#27084=CARTESIAN_POINT('Ctrl Pts',(-1.71508654427022,-1.,1.05760163192481));
#27085=CARTESIAN_POINT('Ctrl Pts',(-1.71508654427022,1.,1.05760163192481));
#27086=CARTESIAN_POINT('Ctrl Pts',(-1.71874858456908,-1.,1.0624732468065));
#27087=CARTESIAN_POINT('Ctrl Pts',(-1.71874858456908,1.,1.0624732468065));
#27088=CARTESIAN_POINT('Ctrl Pts',(-1.72238500928456,-1.,1.06738966975463));
#27089=CARTESIAN_POINT('Ctrl Pts',(-1.72238500928456,1.,1.06738966975463));
#27090=CARTESIAN_POINT('Ctrl Pts',(-1.72599406198489,-1.,1.07234866990252));
#27091=CARTESIAN_POINT('Ctrl Pts',(-1.72599406198489,1.,1.07234866990252));
#27092=CARTESIAN_POINT('Ctrl Pts',(-1.72957248977424,-1.,1.0773470373727));
#27093=CARTESIAN_POINT('Ctrl Pts',(-1.72957248977424,1.,1.0773470373727));
#27094=CARTESIAN_POINT('Ctrl Pts',(-1.73311705663407,-1.,1.08238162784749));
#27095=CARTESIAN_POINT('Ctrl Pts',(-1.73311705663407,1.,1.08238162784749));
#27096=CARTESIAN_POINT('Ctrl Pts',(-1.73662628326093,-1.,1.08745056285429));
#27097=CARTESIAN_POINT('Ctrl Pts',(-1.73662628326093,1.,1.08745056285429));
#27098=CARTESIAN_POINT('Ctrl Pts',(-1.74010053962252,-1.,1.09255329056496));
#27099=CARTESIAN_POINT('Ctrl Pts',(-1.74010053962252,1.,1.09255329056496));
#27100=CARTESIAN_POINT('Ctrl Pts',(-1.74354119236212,-1.,1.09768999241229));
#27101=CARTESIAN_POINT('Ctrl Pts',(-1.74354119236212,1.,1.09768999241229));
#27102=CARTESIAN_POINT('Ctrl Pts',(-1.74695004214924,-1.,1.10286118991144));
#27103=CARTESIAN_POINT('Ctrl Pts',(-1.74695004214924,1.,1.10286118991144));
#27104=CARTESIAN_POINT('Ctrl Pts',(-1.75032866075914,-1.,1.10806728183003));
#27105=CARTESIAN_POINT('Ctrl Pts',(-1.75032866075914,1.,1.10806728183003));
#27106=CARTESIAN_POINT('Ctrl Pts',(-1.75367772094617,-1.,1.11330807582542));
#27107=CARTESIAN_POINT('Ctrl Pts',(-1.75367772094617,1.,1.11330807582542));
#27108=CARTESIAN_POINT('Ctrl Pts',(-1.75699720772089,-1.,1.11858293216752));
#27109=CARTESIAN_POINT('Ctrl Pts',(-1.75699720772089,1.,1.11858293216752));
#27110=CARTESIAN_POINT('Ctrl Pts',(-1.76028671825084,-1.,1.12389096855078));
#27111=CARTESIAN_POINT('Ctrl Pts',(-1.76028671825084,1.,1.12389096855078));
#27112=CARTESIAN_POINT('Ctrl Pts',(-1.76354571966171,-1.,1.12923123555076));
#27113=CARTESIAN_POINT('Ctrl Pts',(-1.76354571966171,1.,1.12923123555076));
#27114=CARTESIAN_POINT('Ctrl Pts',(-1.76677384551883,-1.,1.13460291804635));
#27115=CARTESIAN_POINT('Ctrl Pts',(-1.76677384551883,1.,1.13460291804635));
#27116=CARTESIAN_POINT('Ctrl Pts',(-1.76997111386806,-1.,1.14000548337));
#27117=CARTESIAN_POINT('Ctrl Pts',(-1.76997111386806,1.,1.14000548337));
#27118=CARTESIAN_POINT('Ctrl Pts',(-1.77313777896234,-1.,1.14543858226948));
#27119=CARTESIAN_POINT('Ctrl Pts',(-1.77313777896234,1.,1.14543858226948));
#27120=CARTESIAN_POINT('Ctrl Pts',(-1.77627422557034,-1.,1.15090197841531));
#27121=CARTESIAN_POINT('Ctrl Pts',(-1.77627422557034,1.,1.15090197841531));
#27122=CARTESIAN_POINT('Ctrl Pts',(-1.77938085564261,-1.,1.15639547194689));
#27123=CARTESIAN_POINT('Ctrl Pts',(-1.77938085564261,1.,1.15639547194689));
#27124=CARTESIAN_POINT('Ctrl Pts',(-1.78245795880949,-1.,1.16191881298458));
#27125=CARTESIAN_POINT('Ctrl Pts',(-1.78245795880949,1.,1.16191881298458));
#27126=CARTESIAN_POINT('Ctrl Pts',(-1.78550566040349,-1.,1.16747166312239));
#27127=CARTESIAN_POINT('Ctrl Pts',(-1.78550566040349,1.,1.16747166312239));
#27128=CARTESIAN_POINT('Ctrl Pts',(-1.78852398877523,-1.,1.17305363177265));
#27129=CARTESIAN_POINT('Ctrl Pts',(-1.78852398877523,1.,1.17305363177265));
#27130=CARTESIAN_POINT('Ctrl Pts',(-1.79151291552646,-1.,1.17866429440781));
#27131=CARTESIAN_POINT('Ctrl Pts',(-1.79151291552646,1.,1.17866429440781));
#27132=CARTESIAN_POINT('Ctrl Pts',(-1.79447240321572,-1.,1.18430321697471));
#27133=CARTESIAN_POINT('Ctrl Pts',(-1.79447240321572,1.,1.18430321697471));
#27134=CARTESIAN_POINT('Ctrl Pts',(-1.79740245923649,-1.,1.1899699793456));
#27135=CARTESIAN_POINT('Ctrl Pts',(-1.79740245923649,1.,1.1899699793456));
#27136=CARTESIAN_POINT('Ctrl Pts',(-1.80030314370121,-1.,1.19566418930405));
#27137=CARTESIAN_POINT('Ctrl Pts',(-1.80030314370121,1.,1.19566418930405));
#27138=CARTESIAN_POINT('Ctrl Pts',(-1.8031745483882,-1.,1.2013854893912));
#27139=CARTESIAN_POINT('Ctrl Pts',(-1.8031745483882,1.,1.2013854893912));
#27140=CARTESIAN_POINT('Ctrl Pts',(-1.80601678480772,-1.,1.20713356605519));
#27141=CARTESIAN_POINT('Ctrl Pts',(-1.80601678480772,1.,1.20713356605519));
#27142=CARTESIAN_POINT('Ctrl Pts',(-1.80882996916931,-1.,1.2129081570818));
#27143=CARTESIAN_POINT('Ctrl Pts',(-1.80882996916931,1.,1.2129081570818));
#27144=CARTESIAN_POINT('Ctrl Pts',(-1.81161420806172,-1.,1.2187090610323));
#27145=CARTESIAN_POINT('Ctrl Pts',(-1.81161420806172,1.,1.2187090610323));
#27146=CARTESIAN_POINT('Ctrl Pts',(-1.81436959209778,-1.,1.22453613304507));
#27147=CARTESIAN_POINT('Ctrl Pts',(-1.81436959209778,1.,1.22453613304507));
#27148=CARTESIAN_POINT('Ctrl Pts',(-1.81655087183054,-1.,1.22921864890975));
#27149=CARTESIAN_POINT('Ctrl Pts',(-1.81655087183054,1.,1.22921864890975));
#27150=CARTESIAN_POINT('Ctrl Pts',(-1.81817389920914,-1.,1.23274224526804));
#27151=CARTESIAN_POINT('Ctrl Pts',(-1.81817389920914,1.,1.23274224526804));
#27152=CARTESIAN_POINT('Ctrl Pts',(-1.81925017193531,-1.,1.23509651170384));
#27153=CARTESIAN_POINT('Ctrl Pts',(-1.81925017193531,1.,1.23509651170384));
#27154=CARTESIAN_POINT('Ctrl Pts',(-1.81978687191668,-1.,1.23627494547115));
#27155=CARTESIAN_POINT('Ctrl Pts',(-1.81978687191668,1.,1.23627494547115));
#27156=CARTESIAN_POINT('',(-1.5055822144029,1.,0.892032620296855));
#27157=CARTESIAN_POINT('Ctrl Pts',(-1.5055822144029,1.,0.892032620296855));
#27158=CARTESIAN_POINT('Ctrl Pts',(-1.50980486807181,1.,0.894452006967538));
#27159=CARTESIAN_POINT('Ctrl Pts',(-1.51805569591479,1.,0.89918504749193));
#27160=CARTESIAN_POINT('Ctrl Pts',(-1.52984849890434,1.,0.905967409640499));
#27161=CARTESIAN_POINT('Ctrl Pts',(-1.54440491152808,1.,0.91437591904658));
#27162=CARTESIAN_POINT('Ctrl Pts',(-1.56065988582509,1.,0.923832188966322));
#27163=CARTESIAN_POINT('Ctrl Pts',(-1.57499388385561,1.,0.932246680128849));
#27164=CARTESIAN_POINT('Ctrl Pts',(-1.58744937489796,1.,0.939646377909319));
#27165=CARTESIAN_POINT('Ctrl Pts',(-1.59810042045408,1.,0.946078063325796));
#27166=CARTESIAN_POINT('Ctrl Pts',(-1.60706069897794,1.,0.951613284361248));
#27167=CARTESIAN_POINT('Ctrl Pts',(-1.61449324337233,1.,0.956354422921573));
#27168=CARTESIAN_POINT('Ctrl Pts',(-1.62061638139929,1.,0.960438326099958));
#27169=CARTESIAN_POINT('Ctrl Pts',(-1.6257193066974,1.,0.964046107037821));
#27170=CARTESIAN_POINT('Ctrl Pts',(-1.63013849959083,1.,0.967387853228041));
#27171=CARTESIAN_POINT('Ctrl Pts',(-1.63420665729609,1.,0.970669715996356));
#27172=CARTESIAN_POINT('Ctrl Pts',(-1.63820952658157,1.,0.974066058287501));
#27173=CARTESIAN_POINT('Ctrl Pts',(-1.64233990826831,1.,0.977689794120297));
#27174=CARTESIAN_POINT('Ctrl Pts',(-1.64665139190834,1.,0.981562530940574));
#27175=CARTESIAN_POINT('Ctrl Pts',(-1.6511001661277,1.,0.985642622921626));
#27176=CARTESIAN_POINT('Ctrl Pts',(-1.65559044289746,1.,0.98985562785445));
#27177=CARTESIAN_POINT('Ctrl Pts',(-1.66001553809916,1.,0.994121836661116));
#27178=CARTESIAN_POINT('Ctrl Pts',(-1.66430758030304,1.,0.998389654952317));
#27179=CARTESIAN_POINT('Ctrl Pts',(-1.66846059277231,1.,1.00265091003682));
#27180=CARTESIAN_POINT('Ctrl Pts',(-1.67250335383248,1.,1.00692206696387));
#27181=CARTESIAN_POINT('Ctrl Pts',(-1.67648246776457,1.,1.01123236493507));
#27182=CARTESIAN_POINT('Ctrl Pts',(-1.6804428989482,1.,1.01561026162787));
#27183=CARTESIAN_POINT('Ctrl Pts',(-1.68440578021739,1.,1.02006795074222));
#27184=CARTESIAN_POINT('Ctrl Pts',(-1.68836910178475,1.,1.02460180535272));
#27185=CARTESIAN_POINT('Ctrl Pts',(-1.69231840863471,1.,1.02919977579155));
#27186=CARTESIAN_POINT('Ctrl Pts',(-1.69623414782769,1.,1.03384646003587));
#27187=CARTESIAN_POINT('Ctrl Pts',(-1.70010052930951,1.,1.03852922490782));
#27188=CARTESIAN_POINT('Ctrl Pts',(-1.70391338707969,1.,1.04324363334546));
#27189=CARTESIAN_POINT('Ctrl Pts',(-1.70767646263641,1.,1.0479908540499));
#27190=CARTESIAN_POINT('Ctrl Pts',(-1.71139783543986,1.,1.05277517202854));
#27191=CARTESIAN_POINT('Ctrl Pts',(-1.71508654427022,1.,1.05760163192481));
#27192=CARTESIAN_POINT('Ctrl Pts',(-1.71874858456908,1.,1.0624732468065));
#27193=CARTESIAN_POINT('Ctrl Pts',(-1.72238500928456,1.,1.06738966975463));
#27194=CARTESIAN_POINT('Ctrl Pts',(-1.72599406198489,1.,1.07234866990252));
#27195=CARTESIAN_POINT('Ctrl Pts',(-1.72957248977424,1.,1.0773470373727));
#27196=CARTESIAN_POINT('Ctrl Pts',(-1.73311705663407,1.,1.08238162784749));
#27197=CARTESIAN_POINT('Ctrl Pts',(-1.73662628326093,1.,1.08745056285429));
#27198=CARTESIAN_POINT('Ctrl Pts',(-1.74010053962252,1.,1.09255329056496));
#27199=CARTESIAN_POINT('Ctrl Pts',(-1.74354119236212,1.,1.09768999241229));
#27200=CARTESIAN_POINT('Ctrl Pts',(-1.74695004214924,1.,1.10286118991144));
#27201=CARTESIAN_POINT('Ctrl Pts',(-1.75032866075914,1.,1.10806728183003));
#27202=CARTESIAN_POINT('Ctrl Pts',(-1.75367772094617,1.,1.11330807582542));
#27203=CARTESIAN_POINT('Ctrl Pts',(-1.75699720772089,1.,1.11858293216752));
#27204=CARTESIAN_POINT('Ctrl Pts',(-1.76028671825084,1.,1.12389096855078));
#27205=CARTESIAN_POINT('Ctrl Pts',(-1.76354571966171,1.,1.12923123555076));
#27206=CARTESIAN_POINT('Ctrl Pts',(-1.76677384551883,1.,1.13460291804635));
#27207=CARTESIAN_POINT('Ctrl Pts',(-1.76997111386806,1.,1.14000548337));
#27208=CARTESIAN_POINT('Ctrl Pts',(-1.77313777896234,1.,1.14543858226948));
#27209=CARTESIAN_POINT('Ctrl Pts',(-1.77627422557034,1.,1.15090197841531));
#27210=CARTESIAN_POINT('Ctrl Pts',(-1.77938085564261,1.,1.15639547194689));
#27211=CARTESIAN_POINT('Ctrl Pts',(-1.78245795880949,1.,1.16191881298458));
#27212=CARTESIAN_POINT('Ctrl Pts',(-1.78550566040349,1.,1.16747166312239));
#27213=CARTESIAN_POINT('Ctrl Pts',(-1.78852398877523,1.,1.17305363177265));
#27214=CARTESIAN_POINT('Ctrl Pts',(-1.79151291552646,1.,1.17866429440781));
#27215=CARTESIAN_POINT('Ctrl Pts',(-1.79447240321572,1.,1.18430321697471));
#27216=CARTESIAN_POINT('Ctrl Pts',(-1.79740245923649,1.,1.1899699793456));
#27217=CARTESIAN_POINT('Ctrl Pts',(-1.80030314370121,1.,1.19566418930405));
#27218=CARTESIAN_POINT('Ctrl Pts',(-1.8031745483882,1.,1.2013854893912));
#27219=CARTESIAN_POINT('Ctrl Pts',(-1.80601678480772,1.,1.20713356605519));
#27220=CARTESIAN_POINT('Ctrl Pts',(-1.80882996916931,1.,1.2129081570818));
#27221=CARTESIAN_POINT('Ctrl Pts',(-1.81161420806172,1.,1.2187090610323));
#27222=CARTESIAN_POINT('Ctrl Pts',(-1.81436959209778,1.,1.22453613304507));
#27223=CARTESIAN_POINT('Ctrl Pts',(-1.81655087183054,1.,1.22921864890975));
#27224=CARTESIAN_POINT('Ctrl Pts',(-1.81817389920914,1.,1.23274224526804));
#27225=CARTESIAN_POINT('Ctrl Pts',(-1.81925017193531,1.,1.23509651170384));
#27226=CARTESIAN_POINT('Ctrl Pts',(-1.81978687191668,1.,1.23627494547115));
#27227=CARTESIAN_POINT('',(-1.5055822144029,0.,0.892032620296856));
#27228=CARTESIAN_POINT('Origin',(0.,0.,0.));
#27229=CARTESIAN_POINT('',(-1.60662857109684,1.,0.693717979106305));
#27230=CARTESIAN_POINT('Origin',(0.,1.,0.));
#27231=CARTESIAN_POINT('',(-1.60662857109684,0.,0.693717979106306));
#27232=CARTESIAN_POINT('Ctrl Pts',(-2.0698113262342,-1.,0.7455743247944));
#27233=CARTESIAN_POINT('Ctrl Pts',(-2.0698113262342,1.,0.7455743247944));
#27234=CARTESIAN_POINT('Ctrl Pts',(-2.06854248895728,-1.,0.745832791378367));
#27235=CARTESIAN_POINT('Ctrl Pts',(-2.06854248895728,1.,0.745832791378367));
#27236=CARTESIAN_POINT('Ctrl Pts',(-2.06600523016815,-1.,0.7463458715442));
#27237=CARTESIAN_POINT('Ctrl Pts',(-2.06600523016815,1.,0.7463458715442));
#27238=CARTESIAN_POINT('Ctrl Pts',(-2.06220058927826,-1.,0.747103932787919));
#27239=CARTESIAN_POINT('Ctrl Pts',(-2.06220058927826,1.,0.747103932787919));
#27240=CARTESIAN_POINT('Ctrl Pts',(-2.05713023031006,-1.,0.748091554183802));
#27241=CARTESIAN_POINT('Ctrl Pts',(-2.05713023031006,1.,0.748091554183802));
#27242=CARTESIAN_POINT('Ctrl Pts',(-2.05079645592154,-1.,0.749287468665046));
#27243=CARTESIAN_POINT('Ctrl Pts',(-2.05079645592154,1.,0.749287468665046));
#27244=CARTESIAN_POINT('Ctrl Pts',(-2.04446689147979,-1.,0.750444657875576));
#27245=CARTESIAN_POINT('Ctrl Pts',(-2.04446689147979,1.,0.750444657875576));
#27246=CARTESIAN_POINT('Ctrl Pts',(-2.03814160092099,-1.,0.751562963361115));
#27247=CARTESIAN_POINT('Ctrl Pts',(-2.03814160092099,1.,0.751562963361115));
#27248=CARTESIAN_POINT('Ctrl Pts',(-2.03182068456221,-1.,0.752642180487211));
#27249=CARTESIAN_POINT('Ctrl Pts',(-2.03182068456221,1.,0.752642180487211));
#27250=CARTESIAN_POINT('Ctrl Pts',(-2.02550428623313,-1.,0.753682061112768));
#27251=CARTESIAN_POINT('Ctrl Pts',(-2.02550428623313,1.,0.753682061112768));
#27252=CARTESIAN_POINT('Ctrl Pts',(-2.01919259405809,-1.,0.754682330722816));
#27253=CARTESIAN_POINT('Ctrl Pts',(-2.01919259405809,1.,0.754682330722816));
#27254=CARTESIAN_POINT('Ctrl Pts',(-2.01288584328084,-1.,0.755642704957865));
#27255=CARTESIAN_POINT('Ctrl Pts',(-2.01288584328084,1.,0.755642704957865));
#27256=CARTESIAN_POINT('Ctrl Pts',(-2.0065843158773,-1.,0.75656290464667));
#27257=CARTESIAN_POINT('Ctrl Pts',(-2.0065843158773,1.,0.75656290464667));
#27258=CARTESIAN_POINT('Ctrl Pts',(-2.00028834739178,-1.,0.757442676862724));
#27259=CARTESIAN_POINT('Ctrl Pts',(-2.00028834739178,1.,0.757442676862724));
#27260=CARTESIAN_POINT('Ctrl Pts',(-1.99399831098817,-1.,0.758281796766761));
#27261=CARTESIAN_POINT('Ctrl Pts',(-1.99399831098817,1.,0.758281796766761));
#27262=CARTESIAN_POINT('Ctrl Pts',(-1.98771456680874,-1.,0.759080037802488));
#27263=CARTESIAN_POINT('Ctrl Pts',(-1.98771456680874,1.,0.759080037802488));
#27264=CARTESIAN_POINT('Ctrl Pts',(-1.98143741418172,-1.,0.75983714745219));
#27265=CARTESIAN_POINT('Ctrl Pts',(-1.98143741418172,1.,0.75983714745219));
#27266=CARTESIAN_POINT('Ctrl Pts',(-1.97516705321494,-1.,0.760552825409757));
#27267=CARTESIAN_POINT('Ctrl Pts',(-1.97516705321494,1.,0.760552825409757));
#27268=CARTESIAN_POINT('Ctrl Pts',(-1.96890351582499,-1.,0.76122669048382));
#27269=CARTESIAN_POINT('Ctrl Pts',(-1.96890351582499,1.,0.76122669048382));
#27270=CARTESIAN_POINT('Ctrl Pts',(-1.96264672744186,-1.,0.761858300014423));
#27271=CARTESIAN_POINT('Ctrl Pts',(-1.96264672744186,1.,0.761858300014423));
#27272=CARTESIAN_POINT('Ctrl Pts',(-1.95639665309869,-1.,0.762447203806179));
#27273=CARTESIAN_POINT('Ctrl Pts',(-1.95639665309869,1.,0.762447203806179));
#27274=CARTESIAN_POINT('Ctrl Pts',(-1.95015342590024,-1.,0.762992990878769));
#27275=CARTESIAN_POINT('Ctrl Pts',(-1.95015342590024,1.,0.762992990878769));
#27276=CARTESIAN_POINT('Ctrl Pts',(-1.9439174661764,-1.,0.763495333538629));
#27277=CARTESIAN_POINT('Ctrl Pts',(-1.9439174661764,1.,0.763495333538629));
#27278=CARTESIAN_POINT('Ctrl Pts',(-1.93768964875886,-1.,0.763954049121458));
#27279=CARTESIAN_POINT('Ctrl Pts',(-1.93768964875886,1.,0.763954049121458));
#27280=CARTESIAN_POINT('Ctrl Pts',(-1.93147105496382,-1.,0.76436901067394));
#27281=CARTESIAN_POINT('Ctrl Pts',(-1.93147105496382,1.,0.76436901067394));
#27282=CARTESIAN_POINT('Ctrl Pts',(-1.92526263537048,-1.,0.764740025488211));
#27283=CARTESIAN_POINT('Ctrl Pts',(-1.92526263537048,1.,0.764740025488211));
#27284=CARTESIAN_POINT('Ctrl Pts',(-1.91906491634196,-1.,0.765066729667088));
#27285=CARTESIAN_POINT('Ctrl Pts',(-1.91906491634196,1.,0.765066729667088));
#27286=CARTESIAN_POINT('Ctrl Pts',(-1.91287765805169,-1.,0.765348465884722));
#27287=CARTESIAN_POINT('Ctrl Pts',(-1.91287765805169,1.,0.765348465884722));
#27288=CARTESIAN_POINT('Ctrl Pts',(-1.90669961402356,-1.,0.765584196937919));
#27289=CARTESIAN_POINT('Ctrl Pts',(-1.90669961402356,1.,0.765584196937919));
#27290=CARTESIAN_POINT('Ctrl Pts',(-1.90052930393596,-1.,0.765772772593386));
#27291=CARTESIAN_POINT('Ctrl Pts',(-1.90052930393596,1.,0.765772772593386));
#27292=CARTESIAN_POINT('Ctrl Pts',(-1.89436577771388,-1.,0.765913193856978));
#27293=CARTESIAN_POINT('Ctrl Pts',(-1.89436577771388,1.,0.765913193856978));
#27294=CARTESIAN_POINT('Ctrl Pts',(-1.88820926433409,-1.,0.766004837062091));
#27295=CARTESIAN_POINT('Ctrl Pts',(-1.88820926433409,1.,0.766004837062091));
#27296=CARTESIAN_POINT('Ctrl Pts',(-1.88206215302561,-1.,0.766047794851864));
#27297=CARTESIAN_POINT('Ctrl Pts',(-1.88206215302561,1.,0.766047794851864));
#27298=CARTESIAN_POINT('Ctrl Pts',(-1.87592888967883,-1.,0.766042837036744));
#27299=CARTESIAN_POINT('Ctrl Pts',(-1.87592888967883,1.,0.766042837036744));
#27300=CARTESIAN_POINT('Ctrl Pts',(-1.86981398314341,-1.,0.765990708546091));
#27301=CARTESIAN_POINT('Ctrl Pts',(-1.86981398314341,1.,0.765990708546091));
#27302=CARTESIAN_POINT('Ctrl Pts',(-1.86372027063312,-1.,0.765891519092547));
#27303=CARTESIAN_POINT('Ctrl Pts',(-1.86372027063312,1.,0.765891519092547));
#27304=CARTESIAN_POINT('Ctrl Pts',(-1.85764741390394,-1.,0.765744212909318));
#27305=CARTESIAN_POINT('Ctrl Pts',(-1.85764741390394,1.,0.765744212909318));
#27306=CARTESIAN_POINT('Ctrl Pts',(-1.85158945130063,-1.,0.765545710619062));
#27307=CARTESIAN_POINT('Ctrl Pts',(-1.85158945130063,1.,0.765545710619062));
#27308=CARTESIAN_POINT('Ctrl Pts',(-1.84553698875924,-1.,0.765291664862029));
#27309=CARTESIAN_POINT('Ctrl Pts',(-1.84553698875924,1.,0.765291664862029));
#27310=CARTESIAN_POINT('Ctrl Pts',(-1.83948181064835,-1.,0.764978057881737));
#27311=CARTESIAN_POINT('Ctrl Pts',(-1.83948181064835,1.,0.764978057881737));
#27312=CARTESIAN_POINT('Ctrl Pts',(-1.83342077227142,-1.,0.764602549687853));
#27313=CARTESIAN_POINT('Ctrl Pts',(-1.83342077227142,1.,0.764602549687853));
#27314=CARTESIAN_POINT('Ctrl Pts',(-1.82735991200065,-1.,0.764165902605995));
#27315=CARTESIAN_POINT('Ctrl Pts',(-1.82735991200065,1.,0.764165902605995));
#27316=CARTESIAN_POINT('Ctrl Pts',(-1.82131873145266,-1.,0.763673465462726));
#27317=CARTESIAN_POINT('Ctrl Pts',(-1.82131873145266,1.,0.763673465462726));
#27318=CARTESIAN_POINT('Ctrl Pts',(-1.8153211840553,-1.,0.763132003836634));
#27319=CARTESIAN_POINT('Ctrl Pts',(-1.8153211840553,1.,0.763132003836634));
#27320=CARTESIAN_POINT('Ctrl Pts',(-1.80938551463965,-1.,0.762546129463938));
#27321=CARTESIAN_POINT('Ctrl Pts',(-1.80938551463965,1.,0.762546129463938));
#27322=CARTESIAN_POINT('Ctrl Pts',(-1.80351583877342,-1.,0.761915336443547));
#27323=CARTESIAN_POINT('Ctrl Pts',(-1.80351583877342,1.,0.761915336443547));
#27324=CARTESIAN_POINT('Ctrl Pts',(-1.79768986997783,-1.,0.761229695230558));
#27325=CARTESIAN_POINT('Ctrl Pts',(-1.79768986997783,1.,0.761229695230558));
#27326=CARTESIAN_POINT('Ctrl Pts',(-1.7918581561088,-1.,0.760469555880749));
#27327=CARTESIAN_POINT('Ctrl Pts',(-1.7918581561088,1.,0.760469555880749));
#27328=CARTESIAN_POINT('Ctrl Pts',(-1.78596964884604,-1.,0.759614401110189));
#27329=CARTESIAN_POINT('Ctrl Pts',(-1.78596964884604,1.,0.759614401110189));
#27330=CARTESIAN_POINT('Ctrl Pts',(-1.77999411220945,-1.,0.758650626677518));
#27331=CARTESIAN_POINT('Ctrl Pts',(-1.77999411220945,1.,0.758650626677518));
#27332=CARTESIAN_POINT('Ctrl Pts',(-1.77394167108292,-1.,0.757578264077029));
#27333=CARTESIAN_POINT('Ctrl Pts',(-1.77394167108292,1.,0.757578264077029));
#27334=CARTESIAN_POINT('Ctrl Pts',(-1.76789396002998,-1.,0.75642189602781));
#27335=CARTESIAN_POINT('Ctrl Pts',(-1.76789396002998,1.,0.75642189602781));
#27336=CARTESIAN_POINT('Ctrl Pts',(-1.76197817240128,-1.,0.755220979974461));
#27337=CARTESIAN_POINT('Ctrl Pts',(-1.76197817240128,1.,0.755220979974461));
#27338=CARTESIAN_POINT('Ctrl Pts',(-1.75631083600019,-1.,0.754009254027829));
#27339=CARTESIAN_POINT('Ctrl Pts',(-1.75631083600019,1.,0.754009254027829));
#27340=CARTESIAN_POINT('Ctrl Pts',(-1.75095139468794,-1.,0.752797683531314));
#27341=CARTESIAN_POINT('Ctrl Pts',(-1.75095139468794,1.,0.752797683531314));
#27342=CARTESIAN_POINT('Ctrl Pts',(-1.74585086852502,-1.,0.751555614164482));
#27343=CARTESIAN_POINT('Ctrl Pts',(-1.74585086852502,1.,0.751555614164482));
#27344=CARTESIAN_POINT('Ctrl Pts',(-1.74080458267114,-1.,0.750193435981249));
#27345=CARTESIAN_POINT('Ctrl Pts',(-1.74080458267114,1.,0.750193435981249));
#27346=CARTESIAN_POINT('Ctrl Pts',(-1.7355035168033,-1.,0.74858246295687));
#27347=CARTESIAN_POINT('Ctrl Pts',(-1.7355035168033,1.,0.74858246295687));
#27348=CARTESIAN_POINT('Ctrl Pts',(-1.72958533647714,-1.,0.746574710097752));
#27349=CARTESIAN_POINT('Ctrl Pts',(-1.72958533647714,1.,0.746574710097752));
#27350=CARTESIAN_POINT('Ctrl Pts',(-1.72268229916769,-1.,0.744021445433093));
#27351=CARTESIAN_POINT('Ctrl Pts',(-1.72268229916769,1.,0.744021445433093));
#27352=CARTESIAN_POINT('Ctrl Pts',(-1.71447789751001,-1.,0.74079516202821));
#27353=CARTESIAN_POINT('Ctrl Pts',(-1.71447789751001,1.,0.74079516202821));
#27354=CARTESIAN_POINT('Ctrl Pts',(-1.70473309004249,-1.,0.736799665716932));
#27355=CARTESIAN_POINT('Ctrl Pts',(-1.70473309004249,1.,0.736799665716932));
#27356=CARTESIAN_POINT('Ctrl Pts',(-1.69326921972915,-1.,0.731963238685357));
#27357=CARTESIAN_POINT('Ctrl Pts',(-1.69326921972915,1.,0.731963238685357));
#27358=CARTESIAN_POINT('Ctrl Pts',(-1.67996158451922,-1.,0.726235967982445));
#27359=CARTESIAN_POINT('Ctrl Pts',(-1.67996158451922,1.,0.726235967982445));
#27360=CARTESIAN_POINT('Ctrl Pts',(-1.66472880551777,-1.,0.71958543378795));
#27361=CARTESIAN_POINT('Ctrl Pts',(-1.66472880551777,1.,0.71958543378795));
#27362=CARTESIAN_POINT('Ctrl Pts',(-1.64752408828442,-1.,0.711993139340447));
#27363=CARTESIAN_POINT('Ctrl Pts',(-1.64752408828442,1.,0.711993139340447));
#27364=CARTESIAN_POINT('Ctrl Pts',(-1.6321654166204,-1.,0.705159151977294));
#27365=CARTESIAN_POINT('Ctrl Pts',(-1.6321654166204,1.,0.705159151977294));
#27366=CARTESIAN_POINT('Ctrl Pts',(-1.61974673471117,-1.,0.699605146398837));
#27367=CARTESIAN_POINT('Ctrl Pts',(-1.61974673471117,1.,0.699605146398837));
#27368=CARTESIAN_POINT('Ctrl Pts',(-1.61106790957619,-1.,0.69571209787897));
#27369=CARTESIAN_POINT('Ctrl Pts',(-1.61106790957619,1.,0.69571209787897));
#27370=CARTESIAN_POINT('Ctrl Pts',(-1.60662857109684,-1.,0.693717979106305));
#27371=CARTESIAN_POINT('Ctrl Pts',(-1.60662857109684,1.,0.693717979106305));
#27372=CARTESIAN_POINT('',(-2.0698113262342,1.,0.7455743247944));
#27373=CARTESIAN_POINT('Ctrl Pts',(-2.0698113262342,1.,0.7455743247944));
#27374=CARTESIAN_POINT('Ctrl Pts',(-2.06854248895728,1.,0.745832791378367));
#27375=CARTESIAN_POINT('Ctrl Pts',(-2.06600523016815,1.,0.7463458715442));
#27376=CARTESIAN_POINT('Ctrl Pts',(-2.06220058927826,1.,0.747103932787919));
#27377=CARTESIAN_POINT('Ctrl Pts',(-2.05713023031006,1.,0.748091554183802));
#27378=CARTESIAN_POINT('Ctrl Pts',(-2.05079645592154,1.,0.749287468665046));
#27379=CARTESIAN_POINT('Ctrl Pts',(-2.04446689147979,1.,0.750444657875576));
#27380=CARTESIAN_POINT('Ctrl Pts',(-2.03814160092099,1.,0.751562963361115));
#27381=CARTESIAN_POINT('Ctrl Pts',(-2.03182068456221,1.,0.752642180487211));
#27382=CARTESIAN_POINT('Ctrl Pts',(-2.02550428623313,1.,0.753682061112768));
#27383=CARTESIAN_POINT('Ctrl Pts',(-2.01919259405809,1.,0.754682330722816));
#27384=CARTESIAN_POINT('Ctrl Pts',(-2.01288584328084,1.,0.755642704957865));
#27385=CARTESIAN_POINT('Ctrl Pts',(-2.0065843158773,1.,0.75656290464667));
#27386=CARTESIAN_POINT('Ctrl Pts',(-2.00028834739178,1.,0.757442676862724));
#27387=CARTESIAN_POINT('Ctrl Pts',(-1.99399831098817,1.,0.758281796766761));
#27388=CARTESIAN_POINT('Ctrl Pts',(-1.98771456680874,1.,0.759080037802488));
#27389=CARTESIAN_POINT('Ctrl Pts',(-1.98143741418172,1.,0.75983714745219));
#27390=CARTESIAN_POINT('Ctrl Pts',(-1.97516705321494,1.,0.760552825409757));
#27391=CARTESIAN_POINT('Ctrl Pts',(-1.96890351582499,1.,0.76122669048382));
#27392=CARTESIAN_POINT('Ctrl Pts',(-1.96264672744186,1.,0.761858300014423));
#27393=CARTESIAN_POINT('Ctrl Pts',(-1.95639665309869,1.,0.762447203806179));
#27394=CARTESIAN_POINT('Ctrl Pts',(-1.95015342590024,1.,0.762992990878769));
#27395=CARTESIAN_POINT('Ctrl Pts',(-1.9439174661764,1.,0.763495333538629));
#27396=CARTESIAN_POINT('Ctrl Pts',(-1.93768964875886,1.,0.763954049121458));
#27397=CARTESIAN_POINT('Ctrl Pts',(-1.93147105496382,1.,0.76436901067394));
#27398=CARTESIAN_POINT('Ctrl Pts',(-1.92526263537048,1.,0.764740025488211));
#27399=CARTESIAN_POINT('Ctrl Pts',(-1.91906491634196,1.,0.765066729667088));
#27400=CARTESIAN_POINT('Ctrl Pts',(-1.91287765805169,1.,0.765348465884722));
#27401=CARTESIAN_POINT('Ctrl Pts',(-1.90669961402356,1.,0.765584196937919));
#27402=CARTESIAN_POINT('Ctrl Pts',(-1.90052930393596,1.,0.765772772593386));
#27403=CARTESIAN_POINT('Ctrl Pts',(-1.89436577771388,1.,0.765913193856978));
#27404=CARTESIAN_POINT('Ctrl Pts',(-1.88820926433409,1.,0.766004837062091));
#27405=CARTESIAN_POINT('Ctrl Pts',(-1.88206215302561,1.,0.766047794851864));
#27406=CARTESIAN_POINT('Ctrl Pts',(-1.87592888967883,1.,0.766042837036744));
#27407=CARTESIAN_POINT('Ctrl Pts',(-1.86981398314341,1.,0.765990708546091));
#27408=CARTESIAN_POINT('Ctrl Pts',(-1.86372027063312,1.,0.765891519092547));
#27409=CARTESIAN_POINT('Ctrl Pts',(-1.85764741390394,1.,0.765744212909318));
#27410=CARTESIAN_POINT('Ctrl Pts',(-1.85158945130063,1.,0.765545710619062));
#27411=CARTESIAN_POINT('Ctrl Pts',(-1.84553698875924,1.,0.765291664862029));
#27412=CARTESIAN_POINT('Ctrl Pts',(-1.83948181064835,1.,0.764978057881737));
#27413=CARTESIAN_POINT('Ctrl Pts',(-1.83342077227142,1.,0.764602549687853));
#27414=CARTESIAN_POINT('Ctrl Pts',(-1.82735991200065,1.,0.764165902605995));
#27415=CARTESIAN_POINT('Ctrl Pts',(-1.82131873145266,1.,0.763673465462726));
#27416=CARTESIAN_POINT('Ctrl Pts',(-1.8153211840553,1.,0.763132003836634));
#27417=CARTESIAN_POINT('Ctrl Pts',(-1.80938551463965,1.,0.762546129463938));
#27418=CARTESIAN_POINT('Ctrl Pts',(-1.80351583877342,1.,0.761915336443547));
#27419=CARTESIAN_POINT('Ctrl Pts',(-1.79768986997783,1.,0.761229695230558));
#27420=CARTESIAN_POINT('Ctrl Pts',(-1.7918581561088,1.,0.760469555880749));
#27421=CARTESIAN_POINT('Ctrl Pts',(-1.78596964884604,1.,0.759614401110189));
#27422=CARTESIAN_POINT('Ctrl Pts',(-1.77999411220945,1.,0.758650626677518));
#27423=CARTESIAN_POINT('Ctrl Pts',(-1.77394167108292,1.,0.757578264077029));
#27424=CARTESIAN_POINT('Ctrl Pts',(-1.76789396002998,1.,0.75642189602781));
#27425=CARTESIAN_POINT('Ctrl Pts',(-1.76197817240128,1.,0.755220979974461));
#27426=CARTESIAN_POINT('Ctrl Pts',(-1.75631083600019,1.,0.754009254027829));
#27427=CARTESIAN_POINT('Ctrl Pts',(-1.75095139468794,1.,0.752797683531314));
#27428=CARTESIAN_POINT('Ctrl Pts',(-1.74585086852502,1.,0.751555614164482));
#27429=CARTESIAN_POINT('Ctrl Pts',(-1.74080458267114,1.,0.750193435981249));
#27430=CARTESIAN_POINT('Ctrl Pts',(-1.7355035168033,1.,0.74858246295687));
#27431=CARTESIAN_POINT('Ctrl Pts',(-1.72958533647714,1.,0.746574710097752));
#27432=CARTESIAN_POINT('Ctrl Pts',(-1.72268229916769,1.,0.744021445433093));
#27433=CARTESIAN_POINT('Ctrl Pts',(-1.71447789751001,1.,0.74079516202821));
#27434=CARTESIAN_POINT('Ctrl Pts',(-1.70473309004249,1.,0.736799665716932));
#27435=CARTESIAN_POINT('Ctrl Pts',(-1.69326921972915,1.,0.731963238685357));
#27436=CARTESIAN_POINT('Ctrl Pts',(-1.67996158451922,1.,0.726235967982445));
#27437=CARTESIAN_POINT('Ctrl Pts',(-1.66472880551777,1.,0.71958543378795));
#27438=CARTESIAN_POINT('Ctrl Pts',(-1.64752408828442,1.,0.711993139340447));
#27439=CARTESIAN_POINT('Ctrl Pts',(-1.6321654166204,1.,0.705159151977294));
#27440=CARTESIAN_POINT('Ctrl Pts',(-1.61974673471117,1.,0.699605146398837));
#27441=CARTESIAN_POINT('Ctrl Pts',(-1.61106790957619,1.,0.69571209787897));
#27442=CARTESIAN_POINT('Ctrl Pts',(-1.60662857109684,1.,0.693717979106305));
#27443=CARTESIAN_POINT('',(-2.0698113262342,0.,0.7455743247944));
#27444=CARTESIAN_POINT('Origin',(-2.11275013067528,0.,0.61342227326009));
#27445=CARTESIAN_POINT('',(-2.11275013067528,1.,0.61342227326009));
#27446=CARTESIAN_POINT('',(-2.0698113262342,1.,0.7455743247944));
#27447=CARTESIAN_POINT('',(-2.11275013067528,0.,0.61342227326009));
#27448=CARTESIAN_POINT('Ctrl Pts',(-1.7075470150345,-1.,0.383122945602004));
#27449=CARTESIAN_POINT('Ctrl Pts',(-1.7075470150345,1.,0.383122945602004));
#27450=CARTESIAN_POINT('Ctrl Pts',(-1.71231062891958,-1.,0.384119047315542));
#27451=CARTESIAN_POINT('Ctrl Pts',(-1.71231062891958,1.,0.384119047315542));
#27452=CARTESIAN_POINT('Ctrl Pts',(-1.72162022246158,-1.,0.38607079032701));
#27453=CARTESIAN_POINT('Ctrl Pts',(-1.72162022246158,1.,0.38607079032701));
#27454=CARTESIAN_POINT('Ctrl Pts',(-1.7349317097561,-1.,0.388877023509191));
#27455=CARTESIAN_POINT('Ctrl Pts',(-1.7349317097561,1.,0.388877023509191));
#27456=CARTESIAN_POINT('Ctrl Pts',(-1.75137405313962,-1.,0.392375812294307));
#27457=CARTESIAN_POINT('Ctrl Pts',(-1.75137405313962,1.,0.392375812294307));
#27458=CARTESIAN_POINT('Ctrl Pts',(-1.7697556004756,-1.,0.39634619612042));
#27459=CARTESIAN_POINT('Ctrl Pts',(-1.7697556004756,1.,0.39634619612042));
#27460=CARTESIAN_POINT('Ctrl Pts',(-1.78598826347533,-1.,0.39991940378308));
#27461=CARTESIAN_POINT('Ctrl Pts',(-1.78598826347533,1.,0.39991940378308));
#27462=CARTESIAN_POINT('Ctrl Pts',(-1.80012077176221,-1.,0.403107976170441));
#27463=CARTESIAN_POINT('Ctrl Pts',(-1.80012077176221,1.,0.403107976170441));
#27464=CARTESIAN_POINT('Ctrl Pts',(-1.81223801813988,-1.,0.405933518411838));
#27465=CARTESIAN_POINT('Ctrl Pts',(-1.81223801813988,1.,0.405933518411838));
#27466=CARTESIAN_POINT('Ctrl Pts',(-1.8224702267854,-1.,0.408428948108533));
#27467=CARTESIAN_POINT('Ctrl Pts',(-1.8224702267854,1.,0.408428948108533));
#27468=CARTESIAN_POINT('Ctrl Pts',(-1.83100408895216,-1.,0.410641256301675));
#27469=CARTESIAN_POINT('Ctrl Pts',(-1.83100408895216,1.,0.410641256301675));
#27470=CARTESIAN_POINT('Ctrl Pts',(-1.83808953475839,-1.,0.412633125322161));
#27471=CARTESIAN_POINT('Ctrl Pts',(-1.83808953475839,1.,0.412633125322161));
#27472=CARTESIAN_POINT('Ctrl Pts',(-1.8440575707371,-1.,0.41448743825434));
#27473=CARTESIAN_POINT('Ctrl Pts',(-1.8440575707371,1.,0.41448743825434));
#27474=CARTESIAN_POINT('Ctrl Pts',(-1.84929312929882,-1.,0.416300022038864));
#27475=CARTESIAN_POINT('Ctrl Pts',(-1.84929312929882,1.,0.416300022038864));
#27476=CARTESIAN_POINT('Ctrl Pts',(-1.85417632856234,-1.,0.418164129143534));
#27477=CARTESIAN_POINT('Ctrl Pts',(-1.85417632856234,1.,0.418164129143534));
#27478=CARTESIAN_POINT('Ctrl Pts',(-1.85903281096686,-1.,0.420157287975619));
#27479=CARTESIAN_POINT('Ctrl Pts',(-1.85903281096686,1.,0.420157287975619));
#27480=CARTESIAN_POINT('Ctrl Pts',(-1.86408083334028,-1.,0.422327307418275));
#27481=CARTESIAN_POINT('Ctrl Pts',(-1.86408083334028,1.,0.422327307418275));
#27482=CARTESIAN_POINT('Ctrl Pts',(-1.86937803944323,-1.,0.424678177291359));
#27483=CARTESIAN_POINT('Ctrl Pts',(-1.86937803944323,1.,0.424678177291359));
#27484=CARTESIAN_POINT('Ctrl Pts',(-1.87486989291484,-1.,0.427183828519102));
#27485=CARTESIAN_POINT('Ctrl Pts',(-1.87486989291484,1.,0.427183828519102));
#27486=CARTESIAN_POINT('Ctrl Pts',(-1.88044229001832,-1.,0.429803062482344));
#27487=CARTESIAN_POINT('Ctrl Pts',(-1.88044229001832,1.,0.429803062482344));
#27488=CARTESIAN_POINT('Ctrl Pts',(-1.88596913666793,-1.,0.432493038548748));
#27489=CARTESIAN_POINT('Ctrl Pts',(-1.88596913666793,1.,0.432493038548748));
#27490=CARTESIAN_POINT('Ctrl Pts',(-1.89136993975504,-1.,0.435225660963383));
#27491=CARTESIAN_POINT('Ctrl Pts',(-1.89136993975504,1.,0.435225660963383));
#27492=CARTESIAN_POINT('Ctrl Pts',(-1.89663648956466,-1.,0.437995003948244));
#27493=CARTESIAN_POINT('Ctrl Pts',(-1.89663648956466,1.,0.437995003948244));
#27494=CARTESIAN_POINT('Ctrl Pts',(-1.90180124389086,-1.,0.440807833704038));
#27495=CARTESIAN_POINT('Ctrl Pts',(-1.90180124389086,1.,0.440807833704038));
#27496=CARTESIAN_POINT('Ctrl Pts',(-1.90691756144898,-1.,0.44367755684915));
#27497=CARTESIAN_POINT('Ctrl Pts',(-1.90691756144898,1.,0.44367755684915));
#27498=CARTESIAN_POINT('Ctrl Pts',(-1.9120369998112,-1.,0.446617343485711));
#27499=CARTESIAN_POINT('Ctrl Pts',(-1.9120369998112,1.,0.446617343485711));
#27500=CARTESIAN_POINT('Ctrl Pts',(-1.91718342555755,-1.,0.449632260106662));
#27501=CARTESIAN_POINT('Ctrl Pts',(-1.91718342555755,1.,0.449632260106662));
#27502=CARTESIAN_POINT('Ctrl Pts',(-1.92235380648502,-1.,0.452719478359432));
#27503=CARTESIAN_POINT('Ctrl Pts',(-1.92235380648502,1.,0.452719478359432));
#27504=CARTESIAN_POINT('Ctrl Pts',(-1.92753067150476,-1.,0.455872005174371));
#27505=CARTESIAN_POINT('Ctrl Pts',(-1.92753067150476,1.,0.455872005174371));
#27506=CARTESIAN_POINT('Ctrl Pts',(-1.93269066517934,-1.,0.459081234547926));
#27507=CARTESIAN_POINT('Ctrl Pts',(-1.93269066517934,1.,0.459081234547926));
#27508=CARTESIAN_POINT('Ctrl Pts',(-1.93781486640821,-1.,0.462340031009056));
#27509=CARTESIAN_POINT('Ctrl Pts',(-1.93781486640821,1.,0.462340031009056));
#27510=CARTESIAN_POINT('Ctrl Pts',(-1.9428979419619,-1.,0.46564546202603));
#27511=CARTESIAN_POINT('Ctrl Pts',(-1.9428979419619,1.,0.46564546202603));
#27512=CARTESIAN_POINT('Ctrl Pts',(-1.94794381136514,-1.,0.468997482913135));
#27513=CARTESIAN_POINT('Ctrl Pts',(-1.94794381136514,1.,0.468997482913135));
#27514=CARTESIAN_POINT('Ctrl Pts',(-1.95296148278133,-1.,0.472397672264072));
#27515=CARTESIAN_POINT('Ctrl Pts',(-1.95296148278133,1.,0.472397672264072));
#27516=CARTESIAN_POINT('Ctrl Pts',(-1.95796111148177,-1.,0.475848034683176));
#27517=CARTESIAN_POINT('Ctrl Pts',(-1.95796111148177,1.,0.475848034683176));
#27518=CARTESIAN_POINT('Ctrl Pts',(-1.96294933055943,-1.,0.479349583074855));
#27519=CARTESIAN_POINT('Ctrl Pts',(-1.96294933055943,1.,0.479349583074855));
#27520=CARTESIAN_POINT('Ctrl Pts',(-1.96792703422362,-1.,0.48290166212069));
#27521=CARTESIAN_POINT('Ctrl Pts',(-1.96792703422362,1.,0.48290166212069));
#27522=CARTESIAN_POINT('Ctrl Pts',(-1.97289186263272,-1.,0.486502692907659));
#27523=CARTESIAN_POINT('Ctrl Pts',(-1.97289186263272,1.,0.486502692907659));
#27524=CARTESIAN_POINT('Ctrl Pts',(-1.97783973019229,-1.,0.490150627860952));
#27525=CARTESIAN_POINT('Ctrl Pts',(-1.97783973019229,1.,0.490150627860952));
#27526=CARTESIAN_POINT('Ctrl Pts',(-1.98276658761821,-1.,0.493843476541494));
#27527=CARTESIAN_POINT('Ctrl Pts',(-1.98276658761821,1.,0.493843476541494));
#27528=CARTESIAN_POINT('Ctrl Pts',(-1.98767044752932,-1.,0.497579909545574));
#27529=CARTESIAN_POINT('Ctrl Pts',(-1.98767044752932,1.,0.497579909545574));
#27530=CARTESIAN_POINT('Ctrl Pts',(-1.99255149126155,-1.,0.501359287727146));
#27531=CARTESIAN_POINT('Ctrl Pts',(-1.99255149126155,1.,0.501359287727146));
#27532=CARTESIAN_POINT('Ctrl Pts',(-1.99741107463572,-1.,0.505181361323026));
#27533=CARTESIAN_POINT('Ctrl Pts',(-1.99741107463572,1.,0.505181361323026));
#27534=CARTESIAN_POINT('Ctrl Pts',(-2.00225107134734,-1.,0.509046069886157));
#27535=CARTESIAN_POINT('Ctrl Pts',(-2.00225107134734,1.,0.509046069886157));
#27536=CARTESIAN_POINT('Ctrl Pts',(-2.00707309946949,-1.,0.512953306961792));
#27537=CARTESIAN_POINT('Ctrl Pts',(-2.00707309946949,1.,0.512953306961792));
#27538=CARTESIAN_POINT('Ctrl Pts',(-2.01187773939242,-1.,0.516902681728687));
#27539=CARTESIAN_POINT('Ctrl Pts',(-2.01187773939242,1.,0.516902681728687));
#27540=CARTESIAN_POINT('Ctrl Pts',(-2.01666477917286,-1.,0.52089359039937));
#27541=CARTESIAN_POINT('Ctrl Pts',(-2.01666477917286,1.,0.52089359039937));
#27542=CARTESIAN_POINT('Ctrl Pts',(-2.02143356304698,-1.,0.524925318333476));
#27543=CARTESIAN_POINT('Ctrl Pts',(-2.02143356304698,1.,0.524925318333476));
#27544=CARTESIAN_POINT('Ctrl Pts',(-2.0261832908329,-1.,0.528997127241914));
#27545=CARTESIAN_POINT('Ctrl Pts',(-2.0261832908329,1.,0.528997127241914));
#27546=CARTESIAN_POINT('Ctrl Pts',(-2.03091336214426,-1.,0.533108355132976));
#27547=CARTESIAN_POINT('Ctrl Pts',(-2.03091336214426,1.,0.533108355132976));
#27548=CARTESIAN_POINT('Ctrl Pts',(-2.03562362954037,-1.,0.537258489833262));
#27549=CARTESIAN_POINT('Ctrl Pts',(-2.03562362954037,1.,0.537258489833262));
#27550=CARTESIAN_POINT('Ctrl Pts',(-2.04031422690527,-1.,0.541447120615659));
#27551=CARTESIAN_POINT('Ctrl Pts',(-2.04031422690527,1.,0.541447120615659));
#27552=CARTESIAN_POINT('Ctrl Pts',(-2.04498544714588,-1.,0.54567390381743));
#27553=CARTESIAN_POINT('Ctrl Pts',(-2.04498544714588,1.,0.54567390381743));
#27554=CARTESIAN_POINT('Ctrl Pts',(-2.04963761077958,-1.,0.549938525150295));
#27555=CARTESIAN_POINT('Ctrl Pts',(-2.04963761077958,1.,0.549938525150295));
#27556=CARTESIAN_POINT('Ctrl Pts',(-2.05427091604413,-1.,0.554240657463906));
#27557=CARTESIAN_POINT('Ctrl Pts',(-2.05427091604413,1.,0.554240657463906));
#27558=CARTESIAN_POINT('Ctrl Pts',(-2.05888537756462,-1.,0.558579940185151));
#27559=CARTESIAN_POINT('Ctrl Pts',(-2.05888537756462,1.,0.558579940185151));
#27560=CARTESIAN_POINT('Ctrl Pts',(-2.06348090160589,-1.,0.562955993082261));
#27561=CARTESIAN_POINT('Ctrl Pts',(-2.06348090160589,1.,0.562955993082261));
#27562=CARTESIAN_POINT('Ctrl Pts',(-2.06805732997334,-1.,0.567368421181087));
#27563=CARTESIAN_POINT('Ctrl Pts',(-2.06805732997334,1.,0.567368421181087));
#27564=CARTESIAN_POINT('Ctrl Pts',(-2.07261449292824,-1.,0.571816823242603));
#27565=CARTESIAN_POINT('Ctrl Pts',(-2.07261449292824,1.,0.571816823242603));
#27566=CARTESIAN_POINT('Ctrl Pts',(-2.07715226767559,-1.,0.576300797416844));
#27567=CARTESIAN_POINT('Ctrl Pts',(-2.07715226767559,1.,0.576300797416844));
#27568=CARTESIAN_POINT('Ctrl Pts',(-2.08167059018418,-1.,0.580819952108063));
#27569=CARTESIAN_POINT('Ctrl Pts',(-2.08167059018418,1.,0.580819952108063));
#27570=CARTESIAN_POINT('Ctrl Pts',(-2.08616943727951,-1.,0.585373918991617));
#27571=CARTESIAN_POINT('Ctrl Pts',(-2.08616943727951,1.,0.585373918991617));
#27572=CARTESIAN_POINT('Ctrl Pts',(-2.09064881812129,-1.,0.589962365403406));
#27573=CARTESIAN_POINT('Ctrl Pts',(-2.09064881812129,1.,0.589962365403406));
#27574=CARTESIAN_POINT('Ctrl Pts',(-2.0951087622027,-1.,0.594585006052162));
#27575=CARTESIAN_POINT('Ctrl Pts',(-2.0951087622027,1.,0.594585006052162));
#27576=CARTESIAN_POINT('Ctrl Pts',(-2.0995493086477,-1.,0.599241616420533));
#27577=CARTESIAN_POINT('Ctrl Pts',(-2.0995493086477,1.,0.599241616420533));
#27578=CARTESIAN_POINT('Ctrl Pts',(-2.10397049886949,-1.,0.60393203073603));
#27579=CARTESIAN_POINT('Ctrl Pts',(-2.10397049886949,1.,0.60393203073603));
#27580=CARTESIAN_POINT('Ctrl Pts',(-2.1074919961518,-1.,0.607711315454876));
#27581=CARTESIAN_POINT('Ctrl Pts',(-2.1074919961518,1.,0.607711315454876));
#27582=CARTESIAN_POINT('Ctrl Pts',(-2.11012443807238,-1.,0.610560911689899));
#27583=CARTESIAN_POINT('Ctrl Pts',(-2.11012443807238,1.,0.610560911689899));
#27584=CARTESIAN_POINT('Ctrl Pts',(-2.11187554259986,-1.,0.6124673655618));
#27585=CARTESIAN_POINT('Ctrl Pts',(-2.11187554259986,1.,0.6124673655618));
#27586=CARTESIAN_POINT('Ctrl Pts',(-2.11275013067528,-1.,0.61342227326009));
#27587=CARTESIAN_POINT('Ctrl Pts',(-2.11275013067528,1.,0.61342227326009));
#27588=CARTESIAN_POINT('',(-1.7075470150345,1.,0.383122945602004));
#27589=CARTESIAN_POINT('Ctrl Pts',(-1.7075470150345,1.,0.383122945602004));
#27590=CARTESIAN_POINT('Ctrl Pts',(-1.71231062891958,1.,0.384119047315542));
#27591=CARTESIAN_POINT('Ctrl Pts',(-1.72162022246158,1.,0.38607079032701));
#27592=CARTESIAN_POINT('Ctrl Pts',(-1.7349317097561,1.,0.388877023509191));
#27593=CARTESIAN_POINT('Ctrl Pts',(-1.75137405313962,1.,0.392375812294307));
#27594=CARTESIAN_POINT('Ctrl Pts',(-1.7697556004756,1.,0.39634619612042));
#27595=CARTESIAN_POINT('Ctrl Pts',(-1.78598826347533,1.,0.39991940378308));
#27596=CARTESIAN_POINT('Ctrl Pts',(-1.80012077176221,1.,0.403107976170441));
#27597=CARTESIAN_POINT('Ctrl Pts',(-1.81223801813988,1.,0.405933518411838));
#27598=CARTESIAN_POINT('Ctrl Pts',(-1.8224702267854,1.,0.408428948108533));
#27599=CARTESIAN_POINT('Ctrl Pts',(-1.83100408895216,1.,0.410641256301675));
#27600=CARTESIAN_POINT('Ctrl Pts',(-1.83808953475839,1.,0.412633125322161));
#27601=CARTESIAN_POINT('Ctrl Pts',(-1.8440575707371,1.,0.41448743825434));
#27602=CARTESIAN_POINT('Ctrl Pts',(-1.84929312929882,1.,0.416300022038864));
#27603=CARTESIAN_POINT('Ctrl Pts',(-1.85417632856234,1.,0.418164129143534));
#27604=CARTESIAN_POINT('Ctrl Pts',(-1.85903281096686,1.,0.420157287975619));
#27605=CARTESIAN_POINT('Ctrl Pts',(-1.86408083334028,1.,0.422327307418275));
#27606=CARTESIAN_POINT('Ctrl Pts',(-1.86937803944323,1.,0.424678177291359));
#27607=CARTESIAN_POINT('Ctrl Pts',(-1.87486989291484,1.,0.427183828519102));
#27608=CARTESIAN_POINT('Ctrl Pts',(-1.88044229001832,1.,0.429803062482344));
#27609=CARTESIAN_POINT('Ctrl Pts',(-1.88596913666793,1.,0.432493038548748));
#27610=CARTESIAN_POINT('Ctrl Pts',(-1.89136993975504,1.,0.435225660963383));
#27611=CARTESIAN_POINT('Ctrl Pts',(-1.89663648956466,1.,0.437995003948244));
#27612=CARTESIAN_POINT('Ctrl Pts',(-1.90180124389086,1.,0.440807833704038));
#27613=CARTESIAN_POINT('Ctrl Pts',(-1.90691756144898,1.,0.44367755684915));
#27614=CARTESIAN_POINT('Ctrl Pts',(-1.9120369998112,1.,0.446617343485711));
#27615=CARTESIAN_POINT('Ctrl Pts',(-1.91718342555755,1.,0.449632260106662));
#27616=CARTESIAN_POINT('Ctrl Pts',(-1.92235380648502,1.,0.452719478359432));
#27617=CARTESIAN_POINT('Ctrl Pts',(-1.92753067150476,1.,0.455872005174371));
#27618=CARTESIAN_POINT('Ctrl Pts',(-1.93269066517934,1.,0.459081234547926));
#27619=CARTESIAN_POINT('Ctrl Pts',(-1.93781486640821,1.,0.462340031009056));
#27620=CARTESIAN_POINT('Ctrl Pts',(-1.9428979419619,1.,0.46564546202603));
#27621=CARTESIAN_POINT('Ctrl Pts',(-1.94794381136514,1.,0.468997482913135));
#27622=CARTESIAN_POINT('Ctrl Pts',(-1.95296148278133,1.,0.472397672264072));
#27623=CARTESIAN_POINT('Ctrl Pts',(-1.95796111148177,1.,0.475848034683176));
#27624=CARTESIAN_POINT('Ctrl Pts',(-1.96294933055943,1.,0.479349583074855));
#27625=CARTESIAN_POINT('Ctrl Pts',(-1.96792703422362,1.,0.48290166212069));
#27626=CARTESIAN_POINT('Ctrl Pts',(-1.97289186263272,1.,0.486502692907659));
#27627=CARTESIAN_POINT('Ctrl Pts',(-1.97783973019229,1.,0.490150627860952));
#27628=CARTESIAN_POINT('Ctrl Pts',(-1.98276658761821,1.,0.493843476541494));
#27629=CARTESIAN_POINT('Ctrl Pts',(-1.98767044752932,1.,0.497579909545574));
#27630=CARTESIAN_POINT('Ctrl Pts',(-1.99255149126155,1.,0.501359287727146));
#27631=CARTESIAN_POINT('Ctrl Pts',(-1.99741107463572,1.,0.505181361323026));
#27632=CARTESIAN_POINT('Ctrl Pts',(-2.00225107134734,1.,0.509046069886157));
#27633=CARTESIAN_POINT('Ctrl Pts',(-2.00707309946949,1.,0.512953306961792));
#27634=CARTESIAN_POINT('Ctrl Pts',(-2.01187773939242,1.,0.516902681728687));
#27635=CARTESIAN_POINT('Ctrl Pts',(-2.01666477917286,1.,0.52089359039937));
#27636=CARTESIAN_POINT('Ctrl Pts',(-2.02143356304698,1.,0.524925318333476));
#27637=CARTESIAN_POINT('Ctrl Pts',(-2.0261832908329,1.,0.528997127241914));
#27638=CARTESIAN_POINT('Ctrl Pts',(-2.03091336214426,1.,0.533108355132976));
#27639=CARTESIAN_POINT('Ctrl Pts',(-2.03562362954037,1.,0.537258489833262));
#27640=CARTESIAN_POINT('Ctrl Pts',(-2.04031422690527,1.,0.541447120615659));
#27641=CARTESIAN_POINT('Ctrl Pts',(-2.04498544714588,1.,0.54567390381743));
#27642=CARTESIAN_POINT('Ctrl Pts',(-2.04963761077958,1.,0.549938525150295));
#27643=CARTESIAN_POINT('Ctrl Pts',(-2.05427091604413,1.,0.554240657463906));
#27644=CARTESIAN_POINT('Ctrl Pts',(-2.05888537756462,1.,0.558579940185151));
#27645=CARTESIAN_POINT('Ctrl Pts',(-2.06348090160589,1.,0.562955993082261));
#27646=CARTESIAN_POINT('Ctrl Pts',(-2.06805732997334,1.,0.567368421181087));
#27647=CARTESIAN_POINT('Ctrl Pts',(-2.07261449292824,1.,0.571816823242603));
#27648=CARTESIAN_POINT('Ctrl Pts',(-2.07715226767559,1.,0.576300797416844));
#27649=CARTESIAN_POINT('Ctrl Pts',(-2.08167059018418,1.,0.580819952108063));
#27650=CARTESIAN_POINT('Ctrl Pts',(-2.08616943727951,1.,0.585373918991617));
#27651=CARTESIAN_POINT('Ctrl Pts',(-2.09064881812129,1.,0.589962365403406));
#27652=CARTESIAN_POINT('Ctrl Pts',(-2.0951087622027,1.,0.594585006052162));
#27653=CARTESIAN_POINT('Ctrl Pts',(-2.0995493086477,1.,0.599241616420533));
#27654=CARTESIAN_POINT('Ctrl Pts',(-2.10397049886949,1.,0.60393203073603));
#27655=CARTESIAN_POINT('Ctrl Pts',(-2.1074919961518,1.,0.607711315454876));
#27656=CARTESIAN_POINT('Ctrl Pts',(-2.11012443807238,1.,0.610560911689899));
#27657=CARTESIAN_POINT('Ctrl Pts',(-2.11187554259986,1.,0.6124673655618));
#27658=CARTESIAN_POINT('Ctrl Pts',(-2.11275013067528,1.,0.61342227326009));
#27659=CARTESIAN_POINT('',(-1.7075470150345,0.,0.383122945602003));
#27660=CARTESIAN_POINT('Origin',(0.,0.,0.));
#27661=CARTESIAN_POINT('',(-1.74236521665491,1.,0.163289472382896));
#27662=CARTESIAN_POINT('Origin',(0.,1.,0.));
#27663=CARTESIAN_POINT('',(-1.74236521665491,0.,0.163289472382896));
#27664=CARTESIAN_POINT('Ctrl Pts',(-2.19890268624765,-1.,0.069476445021958));
#27665=CARTESIAN_POINT('Ctrl Pts',(-2.19890268624765,1.,0.069476445021958));
#27666=CARTESIAN_POINT('Ctrl Pts',(-2.19777582085423,-1.,0.0701143536325489));
#27667=CARTESIAN_POINT('Ctrl Pts',(-2.19777582085423,1.,0.0701143536325489));
#27668=CARTESIAN_POINT('Ctrl Pts',(-2.19552129484002,-1.,0.0713863779526153));
#27669=CARTESIAN_POINT('Ctrl Pts',(-2.19552129484002,1.,0.0713863779526153));
#27670=CARTESIAN_POINT('Ctrl Pts',(-2.19213712013662,-1.,0.0732830357306724));
#27671=CARTESIAN_POINT('Ctrl Pts',(-2.19213712013662,1.,0.0732830357306724));
#27672=CARTESIAN_POINT('Ctrl Pts',(-2.1876201139953,-1.,0.0757891465836146));
#27673=CARTESIAN_POINT('Ctrl Pts',(-2.1876201139953,1.,0.0757891465836146));
#27674=CARTESIAN_POINT('Ctrl Pts',(-2.18196589448887,-1.,0.0788837727685241));
#27675=CARTESIAN_POINT('Ctrl Pts',(-2.18196589448887,1.,0.0788837727685241));
#27676=CARTESIAN_POINT('Ctrl Pts',(-2.176303712113,-1.,0.0819402680872764));
#27677=CARTESIAN_POINT('Ctrl Pts',(-2.176303712113,1.,0.0819402680872764));
#27678=CARTESIAN_POINT('Ctrl Pts',(-2.17063357870952,-1.,0.0849584620835371));
#27679=CARTESIAN_POINT('Ctrl Pts',(-2.17063357870952,1.,0.0849584620835371));
#27680=CARTESIAN_POINT('Ctrl Pts',(-2.16495552645014,-1.,0.0879381291386921));
#27681=CARTESIAN_POINT('Ctrl Pts',(-2.16495552645014,1.,0.0879381291386921));
#27682=CARTESIAN_POINT('Ctrl Pts',(-2.15926961544516,-1.,0.0908789888107264));
#27683=CARTESIAN_POINT('Ctrl Pts',(-2.15926961544516,1.,0.0908789888107264));
#27684=CARTESIAN_POINT('Ctrl Pts',(-2.1535759397817,-1.,0.0937807218867642));
#27685=CARTESIAN_POINT('Ctrl Pts',(-2.1535759397817,1.,0.0937807218867642));
#27686=CARTESIAN_POINT('Ctrl Pts',(-2.14787463531795,-1.,0.0966429852305457));
#27687=CARTESIAN_POINT('Ctrl Pts',(-2.14787463531795,1.,0.0966429852305457));
#27688=CARTESIAN_POINT('Ctrl Pts',(-2.14216588396025,-1.,0.0994654261990914));
#27689=CARTESIAN_POINT('Ctrl Pts',(-2.14216588396025,1.,0.0994654261990914));
#27690=CARTESIAN_POINT('Ctrl Pts',(-2.13644992667165,-1.,0.1022477005561));
#27691=CARTESIAN_POINT('Ctrl Pts',(-2.13644992667165,1.,0.1022477005561));
#27692=CARTESIAN_POINT('Ctrl Pts',(-2.13072704887293,-1.,0.104989479152739));
#27693=CARTESIAN_POINT('Ctrl Pts',(-2.13072704887293,1.,0.104989479152739));
#27694=CARTESIAN_POINT('Ctrl Pts',(-2.12499752307,-1.,0.10769043523109));
#27695=CARTESIAN_POINT('Ctrl Pts',(-2.12499752307,1.,0.10769043523109));
#27696=CARTESIAN_POINT('Ctrl Pts',(-2.11926155590865,-1.,0.110350236135025));
#27697=CARTESIAN_POINT('Ctrl Pts',(-2.11926155590865,1.,0.110350236135025));
#27698=CARTESIAN_POINT('Ctrl Pts',(-2.11351924490306,-1.,0.112968534419737));
#27699=CARTESIAN_POINT('Ctrl Pts',(-2.11351924490306,1.,0.112968534419737));
#27700=CARTESIAN_POINT('Ctrl Pts',(-2.10777050261309,-1.,0.115544957687926));
#27701=CARTESIAN_POINT('Ctrl Pts',(-2.10777050261309,1.,0.115544957687926));
#27702=CARTESIAN_POINT('Ctrl Pts',(-2.102015121329,-1.,0.118079107988355));
#27703=CARTESIAN_POINT('Ctrl Pts',(-2.102015121329,1.,0.118079107988355));
#27704=CARTESIAN_POINT('Ctrl Pts',(-2.0962529286773,-1.,0.120570567965122));
#27705=CARTESIAN_POINT('Ctrl Pts',(-2.0962529286773,1.,0.120570567965122));
#27706=CARTESIAN_POINT('Ctrl Pts',(-2.09048392424825,-1.,0.123018905621083));
#27707=CARTESIAN_POINT('Ctrl Pts',(-2.09048392424825,1.,0.123018905621083));
#27708=CARTESIAN_POINT('Ctrl Pts',(-2.08470840653643,-1.,0.125423679412061));
#27709=CARTESIAN_POINT('Ctrl Pts',(-2.08470840653643,1.,0.125423679412061));
#27710=CARTESIAN_POINT('Ctrl Pts',(-2.07892715110987,-1.,0.12778444527612));
#27711=CARTESIAN_POINT('Ctrl Pts',(-2.07892715110987,1.,0.12778444527612));
#27712=CARTESIAN_POINT('Ctrl Pts',(-2.07314114713063,-1.,0.130100748328403));
#27713=CARTESIAN_POINT('Ctrl Pts',(-2.07314114713063,1.,0.130100748328403));
#27714=CARTESIAN_POINT('Ctrl Pts',(-2.06735123910326,-1.,0.13237211154771));
#27715=CARTESIAN_POINT('Ctrl Pts',(-2.06735123910326,1.,0.13237211154771));
#27716=CARTESIAN_POINT('Ctrl Pts',(-2.06155781517842,-1.,0.134598026192106));
#27717=CARTESIAN_POINT('Ctrl Pts',(-2.06155781517842,1.,0.134598026192106));
#27718=CARTESIAN_POINT('Ctrl Pts',(-2.05576044414264,-1.,0.136777941218043));
#27719=CARTESIAN_POINT('Ctrl Pts',(-2.05576044414264,1.,0.136777941218043));
#27720=CARTESIAN_POINT('Ctrl Pts',(-2.04995762001328,-1.,0.138911255368966));
#27721=CARTESIAN_POINT('Ctrl Pts',(-2.04995762001328,1.,0.138911255368966));
#27722=CARTESIAN_POINT('Ctrl Pts',(-2.04414757947916,-1.,0.140997332152546));
#27723=CARTESIAN_POINT('Ctrl Pts',(-2.04414757947916,1.,0.140997332152546));
#27724=CARTESIAN_POINT('Ctrl Pts',(-2.03832911025912,-1.,0.143035515058209));
#27725=CARTESIAN_POINT('Ctrl Pts',(-2.03832911025912,1.,0.143035515058209));
#27726=CARTESIAN_POINT('Ctrl Pts',(-2.03250223739942,-1.,0.145025140186057));
#27727=CARTESIAN_POINT('Ctrl Pts',(-2.03250223739942,1.,0.145025140186057));
#27728=CARTESIAN_POINT('Ctrl Pts',(-2.02666926182017,-1.,0.146965557332583));
#27729=CARTESIAN_POINT('Ctrl Pts',(-2.02666926182017,1.,0.146965557332583));
#27730=CARTESIAN_POINT('Ctrl Pts',(-2.02083464969894,-1.,0.148856124775337));
#27731=CARTESIAN_POINT('Ctrl Pts',(-2.02083464969894,1.,0.148856124775337));
#27732=CARTESIAN_POINT('Ctrl Pts',(-2.01500291940238,-1.,0.150696157673078));
#27733=CARTESIAN_POINT('Ctrl Pts',(-2.01500291940238,1.,0.150696157673078));
#27734=CARTESIAN_POINT('Ctrl Pts',(-2.00917680318424,-1.,0.15248488362145));
#27735=CARTESIAN_POINT('Ctrl Pts',(-2.00917680318424,1.,0.15248488362145));
#27736=CARTESIAN_POINT('Ctrl Pts',(-2.00335565310543,-1.,0.154221403049722));
#27737=CARTESIAN_POINT('Ctrl Pts',(-2.00335565310543,1.,0.154221403049722));
#27738=CARTESIAN_POINT('Ctrl Pts',(-1.99753284771497,-1.,0.155904629548783));
#27739=CARTESIAN_POINT('Ctrl Pts',(-1.99753284771497,1.,0.155904629548783));
#27740=CARTESIAN_POINT('Ctrl Pts',(-1.99169810931908,-1.,0.157533331459227));
#27741=CARTESIAN_POINT('Ctrl Pts',(-1.99169810931908,1.,0.157533331459227));
#27742=CARTESIAN_POINT('Ctrl Pts',(-1.98584238283292,-1.,0.159106226437299));
#27743=CARTESIAN_POINT('Ctrl Pts',(-1.98584238283292,1.,0.159106226437299));
#27744=CARTESIAN_POINT('Ctrl Pts',(-1.97996195437559,-1.,0.160622060784611));
#27745=CARTESIAN_POINT('Ctrl Pts',(-1.97996195437559,1.,0.160622060784611));
#27746=CARTESIAN_POINT('Ctrl Pts',(-1.97406280235188,-1.,0.162079693556288));
#27747=CARTESIAN_POINT('Ctrl Pts',(-1.97406280235188,1.,0.162079693556288));
#27748=CARTESIAN_POINT('Ctrl Pts',(-1.96816512677967,-1.,0.163478185457734));
#27749=CARTESIAN_POINT('Ctrl Pts',(-1.96816512677967,1.,0.163478185457734));
#27750=CARTESIAN_POINT('Ctrl Pts',(-1.96229379940136,-1.,0.164816568920269));
#27751=CARTESIAN_POINT('Ctrl Pts',(-1.96229379940136,1.,0.164816568920269));
#27752=CARTESIAN_POINT('Ctrl Pts',(-1.9564675971873,-1.,0.166093592002812));
#27753=CARTESIAN_POINT('Ctrl Pts',(-1.9564675971873,1.,0.166093592002812));
#27754=CARTESIAN_POINT('Ctrl Pts',(-1.95069027794294,-1.,0.167307501784475));
#27755=CARTESIAN_POINT('Ctrl Pts',(-1.95069027794294,1.,0.167307501784475));
#27756=CARTESIAN_POINT('Ctrl Pts',(-1.94493757756931,-1.,0.168455741607556));
#27757=CARTESIAN_POINT('Ctrl Pts',(-1.94493757756931,1.,0.168455741607556));
#27758=CARTESIAN_POINT('Ctrl Pts',(-1.93915639211581,-1.,0.169534904817491));
#27759=CARTESIAN_POINT('Ctrl Pts',(-1.93915639211581,1.,0.169534904817491));
#27760=CARTESIAN_POINT('Ctrl Pts',(-1.93329183155539,-1.,0.170541253116201));
#27761=CARTESIAN_POINT('Ctrl Pts',(-1.93329183155539,1.,0.170541253116201));
#27762=CARTESIAN_POINT('Ctrl Pts',(-1.92731093582036,-1.,0.171471191532988));
#27763=CARTESIAN_POINT('Ctrl Pts',(-1.92731093582036,1.,0.171471191532988));
#27764=CARTESIAN_POINT('Ctrl Pts',(-1.9212233439798,-1.,0.172321621259514));
#27765=CARTESIAN_POINT('Ctrl Pts',(-1.9212233439798,1.,0.172321621259514));
#27766=CARTESIAN_POINT('Ctrl Pts',(-1.91511429159527,-1.,0.173090695383496));
#27767=CARTESIAN_POINT('Ctrl Pts',(-1.91511429159527,1.,0.173090695383496));
#27768=CARTESIAN_POINT('Ctrl Pts',(-1.90911693975267,-1.,0.173776635257817));
#27769=CARTESIAN_POINT('Ctrl Pts',(-1.90911693975267,1.,0.173776635257817));
#27770=CARTESIAN_POINT('Ctrl Pts',(-1.90335253862834,-1.,0.174375518661085));
#27771=CARTESIAN_POINT('Ctrl Pts',(-1.90335253862834,1.,0.174375518661085));
#27772=CARTESIAN_POINT('Ctrl Pts',(-1.89788101117132,-1.,0.174879405091263));
#27773=CARTESIAN_POINT('Ctrl Pts',(-1.89788101117132,1.,0.174879405091263));
#27774=CARTESIAN_POINT('Ctrl Pts',(-1.892646301985,-1.,0.175274276190844));
#27775=CARTESIAN_POINT('Ctrl Pts',(-1.892646301985,1.,0.175274276190844));
#27776=CARTESIAN_POINT('Ctrl Pts',(-1.88742606273259,-1.,0.175538155840648));
#27777=CARTESIAN_POINT('Ctrl Pts',(-1.88742606273259,1.,0.175538155840648));
#27778=CARTESIAN_POINT('Ctrl Pts',(-1.88188663145367,-1.,0.175644148889698));
#27779=CARTESIAN_POINT('Ctrl Pts',(-1.88188663145367,1.,0.175644148889698));
#27780=CARTESIAN_POINT('Ctrl Pts',(-1.87563767773588,-1.,0.175563480746485));
#27781=CARTESIAN_POINT('Ctrl Pts',(-1.87563767773588,1.,0.175563480746485));
#27782=CARTESIAN_POINT('Ctrl Pts',(-1.86828349694799,-1.,0.175268337590758));
#27783=CARTESIAN_POINT('Ctrl Pts',(-1.86828349694799,1.,0.175268337590758));
#27784=CARTESIAN_POINT('Ctrl Pts',(-1.85948367088837,-1.,0.17473525927603));
#27785=CARTESIAN_POINT('Ctrl Pts',(-1.85948367088837,1.,0.17473525927603));
#27786=CARTESIAN_POINT('Ctrl Pts',(-1.8489811319852,-1.,0.173946627587731));
#27787=CARTESIAN_POINT('Ctrl Pts',(-1.8489811319852,1.,0.173946627587731));
#27788=CARTESIAN_POINT('Ctrl Pts',(-1.83658380527692,-1.,0.1728894428919));
#27789=CARTESIAN_POINT('Ctrl Pts',(-1.83658380527692,1.,0.1728894428919));
#27790=CARTESIAN_POINT('Ctrl Pts',(-1.82215766811545,-1.,0.171554770204119));
#27791=CARTESIAN_POINT('Ctrl Pts',(-1.82215766811545,1.,0.171554770204119));
#27792=CARTESIAN_POINT('Ctrl Pts',(-1.80561530629706,-1.,0.169936923904608));
#27793=CARTESIAN_POINT('Ctrl Pts',(-1.80561530629706,1.,0.169936923904608));
#27794=CARTESIAN_POINT('Ctrl Pts',(-1.7869064998507,-1.,0.168032772805197));
#27795=CARTESIAN_POINT('Ctrl Pts',(-1.7869064998507,1.,0.168032772805197));
#27796=CARTESIAN_POINT('Ctrl Pts',(-1.77018771684844,-1.,0.1662793551464));
#27797=CARTESIAN_POINT('Ctrl Pts',(-1.77018771684844,1.,0.1662793551464));
#27798=CARTESIAN_POINT('Ctrl Pts',(-1.75666056638427,-1.,0.164834765707158));
#27799=CARTESIAN_POINT('Ctrl Pts',(-1.75666056638427,1.,0.164834765707158));
#27800=CARTESIAN_POINT('Ctrl Pts',(-1.7472034950333,-1.,0.163814161002002));
#27801=CARTESIAN_POINT('Ctrl Pts',(-1.7472034950333,1.,0.163814161002002));
#27802=CARTESIAN_POINT('Ctrl Pts',(-1.74236521665491,-1.,0.163289472382896));
#27803=CARTESIAN_POINT('Ctrl Pts',(-1.74236521665491,1.,0.163289472382896));
#27804=CARTESIAN_POINT('',(-2.19890268624765,1.,0.069476445021958));
#27805=CARTESIAN_POINT('Ctrl Pts',(-2.19890268624765,1.,0.069476445021958));
#27806=CARTESIAN_POINT('Ctrl Pts',(-2.19777582085423,1.,0.0701143536325489));
#27807=CARTESIAN_POINT('Ctrl Pts',(-2.19552129484002,1.,0.0713863779526153));
#27808=CARTESIAN_POINT('Ctrl Pts',(-2.19213712013662,1.,0.0732830357306724));
#27809=CARTESIAN_POINT('Ctrl Pts',(-2.1876201139953,1.,0.0757891465836146));
#27810=CARTESIAN_POINT('Ctrl Pts',(-2.18196589448887,1.,0.0788837727685241));
#27811=CARTESIAN_POINT('Ctrl Pts',(-2.176303712113,1.,0.0819402680872764));
#27812=CARTESIAN_POINT('Ctrl Pts',(-2.17063357870952,1.,0.0849584620835371));
#27813=CARTESIAN_POINT('Ctrl Pts',(-2.16495552645014,1.,0.0879381291386921));
#27814=CARTESIAN_POINT('Ctrl Pts',(-2.15926961544516,1.,0.0908789888107264));
#27815=CARTESIAN_POINT('Ctrl Pts',(-2.1535759397817,1.,0.0937807218867642));
#27816=CARTESIAN_POINT('Ctrl Pts',(-2.14787463531795,1.,0.0966429852305457));
#27817=CARTESIAN_POINT('Ctrl Pts',(-2.14216588396025,1.,0.0994654261990914));
#27818=CARTESIAN_POINT('Ctrl Pts',(-2.13644992667165,1.,0.1022477005561));
#27819=CARTESIAN_POINT('Ctrl Pts',(-2.13072704887293,1.,0.104989479152739));
#27820=CARTESIAN_POINT('Ctrl Pts',(-2.12499752307,1.,0.10769043523109));
#27821=CARTESIAN_POINT('Ctrl Pts',(-2.11926155590865,1.,0.110350236135025));
#27822=CARTESIAN_POINT('Ctrl Pts',(-2.11351924490306,1.,0.112968534419737));
#27823=CARTESIAN_POINT('Ctrl Pts',(-2.10777050261309,1.,0.115544957687926));
#27824=CARTESIAN_POINT('Ctrl Pts',(-2.102015121329,1.,0.118079107988355));
#27825=CARTESIAN_POINT('Ctrl Pts',(-2.0962529286773,1.,0.120570567965122));
#27826=CARTESIAN_POINT('Ctrl Pts',(-2.09048392424825,1.,0.123018905621083));
#27827=CARTESIAN_POINT('Ctrl Pts',(-2.08470840653643,1.,0.125423679412061));
#27828=CARTESIAN_POINT('Ctrl Pts',(-2.07892715110987,1.,0.12778444527612));
#27829=CARTESIAN_POINT('Ctrl Pts',(-2.07314114713063,1.,0.130100748328403));
#27830=CARTESIAN_POINT('Ctrl Pts',(-2.06735123910326,1.,0.13237211154771));
#27831=CARTESIAN_POINT('Ctrl Pts',(-2.06155781517842,1.,0.134598026192106));
#27832=CARTESIAN_POINT('Ctrl Pts',(-2.05576044414264,1.,0.136777941218043));
#27833=CARTESIAN_POINT('Ctrl Pts',(-2.04995762001328,1.,0.138911255368966));
#27834=CARTESIAN_POINT('Ctrl Pts',(-2.04414757947916,1.,0.140997332152546));
#27835=CARTESIAN_POINT('Ctrl Pts',(-2.03832911025912,1.,0.143035515058209));
#27836=CARTESIAN_POINT('Ctrl Pts',(-2.03250223739942,1.,0.145025140186057));
#27837=CARTESIAN_POINT('Ctrl Pts',(-2.02666926182017,1.,0.146965557332583));
#27838=CARTESIAN_POINT('Ctrl Pts',(-2.02083464969894,1.,0.148856124775337));
#27839=CARTESIAN_POINT('Ctrl Pts',(-2.01500291940238,1.,0.150696157673078));
#27840=CARTESIAN_POINT('Ctrl Pts',(-2.00917680318424,1.,0.15248488362145));
#27841=CARTESIAN_POINT('Ctrl Pts',(-2.00335565310543,1.,0.154221403049722));
#27842=CARTESIAN_POINT('Ctrl Pts',(-1.99753284771497,1.,0.155904629548783));
#27843=CARTESIAN_POINT('Ctrl Pts',(-1.99169810931908,1.,0.157533331459227));
#27844=CARTESIAN_POINT('Ctrl Pts',(-1.98584238283292,1.,0.159106226437299));
#27845=CARTESIAN_POINT('Ctrl Pts',(-1.97996195437559,1.,0.160622060784611));
#27846=CARTESIAN_POINT('Ctrl Pts',(-1.97406280235188,1.,0.162079693556288));
#27847=CARTESIAN_POINT('Ctrl Pts',(-1.96816512677967,1.,0.163478185457734));
#27848=CARTESIAN_POINT('Ctrl Pts',(-1.96229379940136,1.,0.164816568920269));
#27849=CARTESIAN_POINT('Ctrl Pts',(-1.9564675971873,1.,0.166093592002812));
#27850=CARTESIAN_POINT('Ctrl Pts',(-1.95069027794294,1.,0.167307501784475));
#27851=CARTESIAN_POINT('Ctrl Pts',(-1.94493757756931,1.,0.168455741607556));
#27852=CARTESIAN_POINT('Ctrl Pts',(-1.93915639211581,1.,0.169534904817491));
#27853=CARTESIAN_POINT('Ctrl Pts',(-1.93329183155539,1.,0.170541253116201));
#27854=CARTESIAN_POINT('Ctrl Pts',(-1.92731093582036,1.,0.171471191532988));
#27855=CARTESIAN_POINT('Ctrl Pts',(-1.9212233439798,1.,0.172321621259514));
#27856=CARTESIAN_POINT('Ctrl Pts',(-1.91511429159527,1.,0.173090695383496));
#27857=CARTESIAN_POINT('Ctrl Pts',(-1.90911693975267,1.,0.173776635257817));
#27858=CARTESIAN_POINT('Ctrl Pts',(-1.90335253862834,1.,0.174375518661085));
#27859=CARTESIAN_POINT('Ctrl Pts',(-1.89788101117132,1.,0.174879405091263));
#27860=CARTESIAN_POINT('Ctrl Pts',(-1.892646301985,1.,0.175274276190844));
#27861=CARTESIAN_POINT('Ctrl Pts',(-1.88742606273259,1.,0.175538155840648));
#27862=CARTESIAN_POINT('Ctrl Pts',(-1.88188663145367,1.,0.175644148889698));
#27863=CARTESIAN_POINT('Ctrl Pts',(-1.87563767773588,1.,0.175563480746485));
#27864=CARTESIAN_POINT('Ctrl Pts',(-1.86828349694799,1.,0.175268337590758));
#27865=CARTESIAN_POINT('Ctrl Pts',(-1.85948367088837,1.,0.17473525927603));
#27866=CARTESIAN_POINT('Ctrl Pts',(-1.8489811319852,1.,0.173946627587731));
#27867=CARTESIAN_POINT('Ctrl Pts',(-1.83658380527692,1.,0.1728894428919));
#27868=CARTESIAN_POINT('Ctrl Pts',(-1.82215766811545,1.,0.171554770204119));
#27869=CARTESIAN_POINT('Ctrl Pts',(-1.80561530629706,1.,0.169936923904608));
#27870=CARTESIAN_POINT('Ctrl Pts',(-1.7869064998507,1.,0.168032772805197));
#27871=CARTESIAN_POINT('Ctrl Pts',(-1.77018771684844,1.,0.1662793551464));
#27872=CARTESIAN_POINT('Ctrl Pts',(-1.75666056638427,1.,0.164834765707158));
#27873=CARTESIAN_POINT('Ctrl Pts',(-1.7472034950333,1.,0.163814161002002));
#27874=CARTESIAN_POINT('Ctrl Pts',(-1.74236521665491,1.,0.163289472382896));
#27875=CARTESIAN_POINT('',(-2.19890268624765,0.,0.069476445021958));
#27876=CARTESIAN_POINT('Origin',(-2.19890268624765,0.,-0.0694764450219585));
#27877=CARTESIAN_POINT('',(-2.19890268624765,1.,-0.0694764450219585));
#27878=CARTESIAN_POINT('',(-2.19890268624765,1.,0.069476445021958));
#27879=CARTESIAN_POINT('',(-2.19890268624765,0.,-0.0694764450219585));
#27880=CARTESIAN_POINT('Ctrl Pts',(-1.74236521665491,-1.,-0.163289472382896));
#27881=CARTESIAN_POINT('Ctrl Pts',(-1.74236521665491,1.,-0.163289472382896));
#27882=CARTESIAN_POINT('Ctrl Pts',(-1.74720349503904,-1.,-0.163814161002474));
#27883=CARTESIAN_POINT('Ctrl Pts',(-1.74720349503904,1.,-0.163814161002474));
#27884=CARTESIAN_POINT('Ctrl Pts',(-1.75666056640041,-1.,-0.164834765708484));
#27885=CARTESIAN_POINT('Ctrl Pts',(-1.75666056640041,1.,-0.164834765708484));
#27886=CARTESIAN_POINT('Ctrl Pts',(-1.77018771687692,-1.,-0.166279355148738));
#27887=CARTESIAN_POINT('Ctrl Pts',(-1.77018771687692,1.,-0.166279355148738));
#27888=CARTESIAN_POINT('Ctrl Pts',(-1.78690649988931,-1.,-0.16803277280837));
#27889=CARTESIAN_POINT('Ctrl Pts',(-1.78690649988931,1.,-0.16803277280837));
#27890=CARTESIAN_POINT('Ctrl Pts',(-1.80561530633924,-1.,-0.169936923908078));
#27891=CARTESIAN_POINT('Ctrl Pts',(-1.80561530633924,1.,-0.169936923908078));
#27892=CARTESIAN_POINT('Ctrl Pts',(-1.82215766815414,-1.,-0.171554770207306));
#27893=CARTESIAN_POINT('Ctrl Pts',(-1.82215766815414,1.,-0.171554770207306));
#27894=CARTESIAN_POINT('Ctrl Pts',(-1.83658380530747,-1.,-0.17288944289442));
#27895=CARTESIAN_POINT('Ctrl Pts',(-1.83658380530747,1.,-0.17288944289442));
#27896=CARTESIAN_POINT('Ctrl Pts',(-1.84898113200543,-1.,-0.173946627589401));
#27897=CARTESIAN_POINT('Ctrl Pts',(-1.84898113200543,1.,-0.173946627589401));
#27898=CARTESIAN_POINT('Ctrl Pts',(-1.85948367089838,-1.,-0.174735259276856));
#27899=CARTESIAN_POINT('Ctrl Pts',(-1.85948367089838,1.,-0.174735259276856));
#27900=CARTESIAN_POINT('Ctrl Pts',(-1.86828349694972,-1.,-0.175268337590901));
#27901=CARTESIAN_POINT('Ctrl Pts',(-1.86828349694972,1.,-0.175268337590901));
#27902=CARTESIAN_POINT('Ctrl Pts',(-1.87563767773249,-1.,-0.175563480746205));
#27903=CARTESIAN_POINT('Ctrl Pts',(-1.87563767773249,1.,-0.175563480746205));
#27904=CARTESIAN_POINT('Ctrl Pts',(-1.88188663144846,-1.,-0.175644148889271));
#27905=CARTESIAN_POINT('Ctrl Pts',(-1.88188663144846,1.,-0.175644148889271));
#27906=CARTESIAN_POINT('Ctrl Pts',(-1.88742606272818,-1.,-0.175538155840286));
#27907=CARTESIAN_POINT('Ctrl Pts',(-1.88742606272818,1.,-0.175538155840286));
#27908=CARTESIAN_POINT('Ctrl Pts',(-1.89264630198279,-1.,-0.175274276190664));
#27909=CARTESIAN_POINT('Ctrl Pts',(-1.89264630198279,1.,-0.175274276190664));
#27910=CARTESIAN_POINT('Ctrl Pts',(-1.89788101117148,-1.,-0.174879405091277));
#27911=CARTESIAN_POINT('Ctrl Pts',(-1.89788101117148,1.,-0.174879405091277));
#27912=CARTESIAN_POINT('Ctrl Pts',(-1.90335253863003,-1.,-0.174375518661222));
#27913=CARTESIAN_POINT('Ctrl Pts',(-1.90335253863003,1.,-0.174375518661222));
#27914=CARTESIAN_POINT('Ctrl Pts',(-1.90911693975475,-1.,-0.173776635257984));
#27915=CARTESIAN_POINT('Ctrl Pts',(-1.90911693975475,1.,-0.173776635257984));
#27916=CARTESIAN_POINT('Ctrl Pts',(-1.91511429159681,-1.,-0.173090695383619));
#27917=CARTESIAN_POINT('Ctrl Pts',(-1.91511429159681,1.,-0.173090695383619));
#27918=CARTESIAN_POINT('Ctrl Pts',(-1.92122334398034,-1.,-0.172321621259557));
#27919=CARTESIAN_POINT('Ctrl Pts',(-1.92122334398034,1.,-0.172321621259557));
#27920=CARTESIAN_POINT('Ctrl Pts',(-1.92731093582,-1.,-0.17147119153296));
#27921=CARTESIAN_POINT('Ctrl Pts',(-1.92731093582,1.,-0.17147119153296));
#27922=CARTESIAN_POINT('Ctrl Pts',(-1.93329183155455,-1.,-0.170541253116136));
#27923=CARTESIAN_POINT('Ctrl Pts',(-1.93329183155455,1.,-0.170541253116136));
#27924=CARTESIAN_POINT('Ctrl Pts',(-1.93915639211497,-1.,-0.169534904817425));
#27925=CARTESIAN_POINT('Ctrl Pts',(-1.93915639211497,1.,-0.169534904817425));
#27926=CARTESIAN_POINT('Ctrl Pts',(-1.94493757756879,-1.,-0.168455741607516));
#27927=CARTESIAN_POINT('Ctrl Pts',(-1.94493757756879,1.,-0.168455741607516));
#27928=CARTESIAN_POINT('Ctrl Pts',(-1.95069027794286,-1.,-0.167307501784469));
#27929=CARTESIAN_POINT('Ctrl Pts',(-1.95069027794286,1.,-0.167307501784469));
#27930=CARTESIAN_POINT('Ctrl Pts',(-1.95646759718755,-1.,-0.166093592002833));
#27931=CARTESIAN_POINT('Ctrl Pts',(-1.95646759718755,1.,-0.166093592002833));
#27932=CARTESIAN_POINT('Ctrl Pts',(-1.96229379940174,-1.,-0.1648165689203));
#27933=CARTESIAN_POINT('Ctrl Pts',(-1.96229379940174,1.,-0.1648165689203));
#27934=CARTESIAN_POINT('Ctrl Pts',(-1.96816512678,-1.,-0.16347818545776));
#27935=CARTESIAN_POINT('Ctrl Pts',(-1.96816512678,1.,-0.16347818545776));
#27936=CARTESIAN_POINT('Ctrl Pts',(-1.97406280235204,-1.,-0.162079693556302));
#27937=CARTESIAN_POINT('Ctrl Pts',(-1.97406280235204,1.,-0.162079693556302));
#27938=CARTESIAN_POINT('Ctrl Pts',(-1.97996195437557,-1.,-0.16062206078461));
#27939=CARTESIAN_POINT('Ctrl Pts',(-1.97996195437557,1.,-0.16062206078461));
#27940=CARTESIAN_POINT('Ctrl Pts',(-1.98584238283279,-1.,-0.159106226437289));
#27941=CARTESIAN_POINT('Ctrl Pts',(-1.98584238283279,1.,-0.159106226437289));
#27942=CARTESIAN_POINT('Ctrl Pts',(-1.99169810931893,-1.,-0.157533331459215));
#27943=CARTESIAN_POINT('Ctrl Pts',(-1.99169810931893,1.,-0.157533331459215));
#27944=CARTESIAN_POINT('Ctrl Pts',(-1.99753284771487,-1.,-0.155904629548775));
#27945=CARTESIAN_POINT('Ctrl Pts',(-1.99753284771487,1.,-0.155904629548775));
#27946=CARTESIAN_POINT('Ctrl Pts',(-2.00335565310539,-1.,-0.154221403049719));
#27947=CARTESIAN_POINT('Ctrl Pts',(-2.00335565310539,1.,-0.154221403049719));
#27948=CARTESIAN_POINT('Ctrl Pts',(-2.00917680318426,-1.,-0.152484883621452));
#27949=CARTESIAN_POINT('Ctrl Pts',(-2.00917680318426,1.,-0.152484883621452));
#27950=CARTESIAN_POINT('Ctrl Pts',(-2.01500291940243,-1.,-0.150696157673084));
#27951=CARTESIAN_POINT('Ctrl Pts',(-2.01500291940243,1.,-0.150696157673084));
#27952=CARTESIAN_POINT('Ctrl Pts',(-2.02083464969897,-1.,-0.148856124775343));
#27953=CARTESIAN_POINT('Ctrl Pts',(-2.02083464969897,1.,-0.148856124775343));
#27954=CARTESIAN_POINT('Ctrl Pts',(-2.02666926182017,-1.,-0.146965557332586));
#27955=CARTESIAN_POINT('Ctrl Pts',(-2.02666926182017,1.,-0.146965557332586));
#27956=CARTESIAN_POINT('Ctrl Pts',(-2.03250223739941,-1.,-0.145025140186058));
#27957=CARTESIAN_POINT('Ctrl Pts',(-2.03250223739941,1.,-0.145025140186058));
#27958=CARTESIAN_POINT('Ctrl Pts',(-2.03832911025913,-1.,-0.143035515058208));
#27959=CARTESIAN_POINT('Ctrl Pts',(-2.03832911025913,1.,-0.143035515058208));
#27960=CARTESIAN_POINT('Ctrl Pts',(-2.04414757947919,-1.,-0.140997332152545));
#27961=CARTESIAN_POINT('Ctrl Pts',(-2.04414757947919,1.,-0.140997332152545));
#27962=CARTESIAN_POINT('Ctrl Pts',(-2.04995762001333,-1.,-0.138911255368966));
#27963=CARTESIAN_POINT('Ctrl Pts',(-2.04995762001333,1.,-0.138911255368966));
#27964=CARTESIAN_POINT('Ctrl Pts',(-2.0557604441427,-1.,-0.136777941218044));
#27965=CARTESIAN_POINT('Ctrl Pts',(-2.0557604441427,1.,-0.136777941218044));
#27966=CARTESIAN_POINT('Ctrl Pts',(-2.06155781517844,-1.,-0.134598026192107));
#27967=CARTESIAN_POINT('Ctrl Pts',(-2.06155781517844,1.,-0.134598026192107));
#27968=CARTESIAN_POINT('Ctrl Pts',(-2.06735123910319,-1.,-0.13237211154771));
#27969=CARTESIAN_POINT('Ctrl Pts',(-2.06735123910319,1.,-0.13237211154771));
#27970=CARTESIAN_POINT('Ctrl Pts',(-2.07314114713047,-1.,-0.130100748328401));
#27971=CARTESIAN_POINT('Ctrl Pts',(-2.07314114713047,1.,-0.130100748328401));
#27972=CARTESIAN_POINT('Ctrl Pts',(-2.07892715110967,-1.,-0.127784445276116));
#27973=CARTESIAN_POINT('Ctrl Pts',(-2.07892715110967,1.,-0.127784445276116));
#27974=CARTESIAN_POINT('Ctrl Pts',(-2.08470840653628,-1.,-0.125423679412058));
#27975=CARTESIAN_POINT('Ctrl Pts',(-2.08470840653628,1.,-0.125423679412058));
#27976=CARTESIAN_POINT('Ctrl Pts',(-2.09048392424826,-1.,-0.123018905621083));
#27977=CARTESIAN_POINT('Ctrl Pts',(-2.09048392424826,1.,-0.123018905621083));
#27978=CARTESIAN_POINT('Ctrl Pts',(-2.09625292867756,-1.,-0.120570567965129));
#27979=CARTESIAN_POINT('Ctrl Pts',(-2.09625292867756,1.,-0.120570567965129));
#27980=CARTESIAN_POINT('Ctrl Pts',(-2.10201512132945,-1.,-0.118079107988368));
#27981=CARTESIAN_POINT('Ctrl Pts',(-2.10201512132945,1.,-0.118079107988368));
#27982=CARTESIAN_POINT('Ctrl Pts',(-2.10777050261359,-1.,-0.11554495768794));
#27983=CARTESIAN_POINT('Ctrl Pts',(-2.10777050261359,1.,-0.11554495768794));
#27984=CARTESIAN_POINT('Ctrl Pts',(-2.11351924490335,-1.,-0.112968534419746));
#27985=CARTESIAN_POINT('Ctrl Pts',(-2.11351924490335,1.,-0.112968534419746));
#27986=CARTESIAN_POINT('Ctrl Pts',(-2.11926155590849,-1.,-0.11035023613502));
#27987=CARTESIAN_POINT('Ctrl Pts',(-2.11926155590849,1.,-0.11035023613502));
#27988=CARTESIAN_POINT('Ctrl Pts',(-2.12499752306927,-1.,-0.107690435231068));
#27989=CARTESIAN_POINT('Ctrl Pts',(-2.12499752306927,1.,-0.107690435231068));
#27990=CARTESIAN_POINT('Ctrl Pts',(-2.1307270488718,-1.,-0.104989479152703));
#27991=CARTESIAN_POINT('Ctrl Pts',(-2.1307270488718,1.,-0.104989479152703));
#27992=CARTESIAN_POINT('Ctrl Pts',(-2.13644992667052,-1.,-0.102247700556064));
#27993=CARTESIAN_POINT('Ctrl Pts',(-2.13644992667052,1.,-0.102247700556064));
#27994=CARTESIAN_POINT('Ctrl Pts',(-2.14216588395974,-1.,-0.0994654261990744));
#27995=CARTESIAN_POINT('Ctrl Pts',(-2.14216588395974,1.,-0.0994654261990744));
#27996=CARTESIAN_POINT('Ctrl Pts',(-2.14787463531864,-1.,-0.096642985230569));
#27997=CARTESIAN_POINT('Ctrl Pts',(-2.14787463531864,1.,-0.096642985230569));
#27998=CARTESIAN_POINT('Ctrl Pts',(-2.15357593978377,-1.,-0.0937807218868346));
#27999=CARTESIAN_POINT('Ctrl Pts',(-2.15357593978377,1.,-0.0937807218868346));
#28000=CARTESIAN_POINT('Ctrl Pts',(-2.15926961544808,-1.,-0.0908789888108267));
#28001=CARTESIAN_POINT('Ctrl Pts',(-2.15926961544808,1.,-0.0908789888108267));
#28002=CARTESIAN_POINT('Ctrl Pts',(-2.16495552645275,-1.,-0.0879381291387824));
#28003=CARTESIAN_POINT('Ctrl Pts',(-2.16495552645275,1.,-0.0879381291387824));
#28004=CARTESIAN_POINT('Ctrl Pts',(-2.17063357871031,-1.,-0.0849584620835644));
#28005=CARTESIAN_POINT('Ctrl Pts',(-2.17063357871031,1.,-0.0849584620835644));
#28006=CARTESIAN_POINT('Ctrl Pts',(-2.1763037121106,-1.,-0.0819402680871941));
#28007=CARTESIAN_POINT('Ctrl Pts',(-2.1763037121106,1.,-0.0819402680871941));
#28008=CARTESIAN_POINT('Ctrl Pts',(-2.18196589448304,-1.,-0.0788837727683229));
#28009=CARTESIAN_POINT('Ctrl Pts',(-2.18196589448304,1.,-0.0788837727683229));
#28010=CARTESIAN_POINT('Ctrl Pts',(-2.1876201139874,-1.,-0.0757891465833413));
#28011=CARTESIAN_POINT('Ctrl Pts',(-2.1876201139874,1.,-0.0757891465833413));
#28012=CARTESIAN_POINT('Ctrl Pts',(-2.19213712012956,-1.,-0.0732830357304277));
#28013=CARTESIAN_POINT('Ctrl Pts',(-2.19213712012956,1.,-0.0732830357304277));
#28014=CARTESIAN_POINT('Ctrl Pts',(-2.19552129483562,-1.,-0.0713863779524629));
#28015=CARTESIAN_POINT('Ctrl Pts',(-2.19552129483562,1.,-0.0713863779524629));
#28016=CARTESIAN_POINT('Ctrl Pts',(-2.19777582085261,-1.,-0.0701143536324927));
#28017=CARTESIAN_POINT('Ctrl Pts',(-2.19777582085261,1.,-0.0701143536324927));
#28018=CARTESIAN_POINT('Ctrl Pts',(-2.19890268624765,-1.,-0.0694764450219585));
#28019=CARTESIAN_POINT('Ctrl Pts',(-2.19890268624765,1.,-0.0694764450219585));
#28020=CARTESIAN_POINT('',(-1.74236521665491,1.,-0.163289472382896));
#28021=CARTESIAN_POINT('Ctrl Pts',(-1.74236521665491,1.,-0.163289472382896));
#28022=CARTESIAN_POINT('Ctrl Pts',(-1.74720349503904,1.,-0.163814161002474));
#28023=CARTESIAN_POINT('Ctrl Pts',(-1.75666056640041,1.,-0.164834765708484));
#28024=CARTESIAN_POINT('Ctrl Pts',(-1.77018771687692,1.,-0.166279355148738));
#28025=CARTESIAN_POINT('Ctrl Pts',(-1.78690649988931,1.,-0.16803277280837));
#28026=CARTESIAN_POINT('Ctrl Pts',(-1.80561530633924,1.,-0.169936923908078));
#28027=CARTESIAN_POINT('Ctrl Pts',(-1.82215766815414,1.,-0.171554770207306));
#28028=CARTESIAN_POINT('Ctrl Pts',(-1.83658380530747,1.,-0.17288944289442));
#28029=CARTESIAN_POINT('Ctrl Pts',(-1.84898113200543,1.,-0.173946627589401));
#28030=CARTESIAN_POINT('Ctrl Pts',(-1.85948367089838,1.,-0.174735259276856));
#28031=CARTESIAN_POINT('Ctrl Pts',(-1.86828349694972,1.,-0.175268337590901));
#28032=CARTESIAN_POINT('Ctrl Pts',(-1.87563767773249,1.,-0.175563480746205));
#28033=CARTESIAN_POINT('Ctrl Pts',(-1.88188663144846,1.,-0.175644148889271));
#28034=CARTESIAN_POINT('Ctrl Pts',(-1.88742606272818,1.,-0.175538155840286));
#28035=CARTESIAN_POINT('Ctrl Pts',(-1.89264630198279,1.,-0.175274276190664));
#28036=CARTESIAN_POINT('Ctrl Pts',(-1.89788101117148,1.,-0.174879405091277));
#28037=CARTESIAN_POINT('Ctrl Pts',(-1.90335253863003,1.,-0.174375518661222));
#28038=CARTESIAN_POINT('Ctrl Pts',(-1.90911693975475,1.,-0.173776635257984));
#28039=CARTESIAN_POINT('Ctrl Pts',(-1.91511429159681,1.,-0.173090695383619));
#28040=CARTESIAN_POINT('Ctrl Pts',(-1.92122334398034,1.,-0.172321621259557));
#28041=CARTESIAN_POINT('Ctrl Pts',(-1.92731093582,1.,-0.17147119153296));
#28042=CARTESIAN_POINT('Ctrl Pts',(-1.93329183155455,1.,-0.170541253116136));
#28043=CARTESIAN_POINT('Ctrl Pts',(-1.93915639211497,1.,-0.169534904817425));
#28044=CARTESIAN_POINT('Ctrl Pts',(-1.94493757756879,1.,-0.168455741607516));
#28045=CARTESIAN_POINT('Ctrl Pts',(-1.95069027794286,1.,-0.167307501784469));
#28046=CARTESIAN_POINT('Ctrl Pts',(-1.95646759718755,1.,-0.166093592002833));
#28047=CARTESIAN_POINT('Ctrl Pts',(-1.96229379940174,1.,-0.1648165689203));
#28048=CARTESIAN_POINT('Ctrl Pts',(-1.96816512678,1.,-0.16347818545776));
#28049=CARTESIAN_POINT('Ctrl Pts',(-1.97406280235204,1.,-0.162079693556302));
#28050=CARTESIAN_POINT('Ctrl Pts',(-1.97996195437557,1.,-0.16062206078461));
#28051=CARTESIAN_POINT('Ctrl Pts',(-1.98584238283279,1.,-0.159106226437289));
#28052=CARTESIAN_POINT('Ctrl Pts',(-1.99169810931893,1.,-0.157533331459215));
#28053=CARTESIAN_POINT('Ctrl Pts',(-1.99753284771487,1.,-0.155904629548775));
#28054=CARTESIAN_POINT('Ctrl Pts',(-2.00335565310539,1.,-0.154221403049719));
#28055=CARTESIAN_POINT('Ctrl Pts',(-2.00917680318426,1.,-0.152484883621452));
#28056=CARTESIAN_POINT('Ctrl Pts',(-2.01500291940243,1.,-0.150696157673084));
#28057=CARTESIAN_POINT('Ctrl Pts',(-2.02083464969897,1.,-0.148856124775343));
#28058=CARTESIAN_POINT('Ctrl Pts',(-2.02666926182017,1.,-0.146965557332586));
#28059=CARTESIAN_POINT('Ctrl Pts',(-2.03250223739941,1.,-0.145025140186058));
#28060=CARTESIAN_POINT('Ctrl Pts',(-2.03832911025913,1.,-0.143035515058208));
#28061=CARTESIAN_POINT('Ctrl Pts',(-2.04414757947919,1.,-0.140997332152545));
#28062=CARTESIAN_POINT('Ctrl Pts',(-2.04995762001333,1.,-0.138911255368966));
#28063=CARTESIAN_POINT('Ctrl Pts',(-2.0557604441427,1.,-0.136777941218044));
#28064=CARTESIAN_POINT('Ctrl Pts',(-2.06155781517844,1.,-0.134598026192107));
#28065=CARTESIAN_POINT('Ctrl Pts',(-2.06735123910319,1.,-0.13237211154771));
#28066=CARTESIAN_POINT('Ctrl Pts',(-2.07314114713047,1.,-0.130100748328401));
#28067=CARTESIAN_POINT('Ctrl Pts',(-2.07892715110967,1.,-0.127784445276116));
#28068=CARTESIAN_POINT('Ctrl Pts',(-2.08470840653628,1.,-0.125423679412058));
#28069=CARTESIAN_POINT('Ctrl Pts',(-2.09048392424826,1.,-0.123018905621083));
#28070=CARTESIAN_POINT('Ctrl Pts',(-2.09625292867756,1.,-0.120570567965129));
#28071=CARTESIAN_POINT('Ctrl Pts',(-2.10201512132945,1.,-0.118079107988368));
#28072=CARTESIAN_POINT('Ctrl Pts',(-2.10777050261359,1.,-0.11554495768794));
#28073=CARTESIAN_POINT('Ctrl Pts',(-2.11351924490335,1.,-0.112968534419746));
#28074=CARTESIAN_POINT('Ctrl Pts',(-2.11926155590849,1.,-0.11035023613502));
#28075=CARTESIAN_POINT('Ctrl Pts',(-2.12499752306927,1.,-0.107690435231068));
#28076=CARTESIAN_POINT('Ctrl Pts',(-2.1307270488718,1.,-0.104989479152703));
#28077=CARTESIAN_POINT('Ctrl Pts',(-2.13644992667052,1.,-0.102247700556064));
#28078=CARTESIAN_POINT('Ctrl Pts',(-2.14216588395974,1.,-0.0994654261990744));
#28079=CARTESIAN_POINT('Ctrl Pts',(-2.14787463531864,1.,-0.096642985230569));
#28080=CARTESIAN_POINT('Ctrl Pts',(-2.15357593978377,1.,-0.0937807218868346));
#28081=CARTESIAN_POINT('Ctrl Pts',(-2.15926961544808,1.,-0.0908789888108267));
#28082=CARTESIAN_POINT('Ctrl Pts',(-2.16495552645275,1.,-0.0879381291387824));
#28083=CARTESIAN_POINT('Ctrl Pts',(-2.17063357871031,1.,-0.0849584620835644));
#28084=CARTESIAN_POINT('Ctrl Pts',(-2.1763037121106,1.,-0.0819402680871941));
#28085=CARTESIAN_POINT('Ctrl Pts',(-2.18196589448304,1.,-0.0788837727683229));
#28086=CARTESIAN_POINT('Ctrl Pts',(-2.1876201139874,1.,-0.0757891465833413));
#28087=CARTESIAN_POINT('Ctrl Pts',(-2.19213712012956,1.,-0.0732830357304277));
#28088=CARTESIAN_POINT('Ctrl Pts',(-2.19552129483562,1.,-0.0713863779524629));
#28089=CARTESIAN_POINT('Ctrl Pts',(-2.19777582085261,1.,-0.0701143536324927));
#28090=CARTESIAN_POINT('Ctrl Pts',(-2.19890268624765,1.,-0.0694764450219585));
#28091=CARTESIAN_POINT('',(-1.74236521665491,0.,-0.163289472382896));
#28092=CARTESIAN_POINT('Origin',(0.,0.,0.));
#28093=CARTESIAN_POINT('',(-1.7075470150345,1.,-0.383122945602004));
#28094=CARTESIAN_POINT('Origin',(0.,1.,0.));
#28095=CARTESIAN_POINT('',(-1.7075470150345,0.,-0.383122945602004));
#28096=CARTESIAN_POINT('Ctrl Pts',(-2.11275013067528,-1.,-0.61342227326009));
#28097=CARTESIAN_POINT('Ctrl Pts',(-2.11275013067528,1.,-0.61342227326009));
#28098=CARTESIAN_POINT('Ctrl Pts',(-2.11187554260142,-1.,-0.61246736556225));
#28099=CARTESIAN_POINT('Ctrl Pts',(-2.11187554260142,1.,-0.61246736556225));
#28100=CARTESIAN_POINT('Ctrl Pts',(-2.11012443807661,-1.,-0.610560911691113));
#28101=CARTESIAN_POINT('Ctrl Pts',(-2.11012443807661,1.,-0.610560911691113));
#28102=CARTESIAN_POINT('Ctrl Pts',(-2.10749199615859,-1.,-0.607711315456826));
#28103=CARTESIAN_POINT('Ctrl Pts',(-2.10749199615859,1.,-0.607711315456826));
#28104=CARTESIAN_POINT('Ctrl Pts',(-2.10397049887709,-1.,-0.603932030738212));
#28105=CARTESIAN_POINT('Ctrl Pts',(-2.10397049887709,1.,-0.603932030738212));
#28106=CARTESIAN_POINT('Ctrl Pts',(-2.09954930865331,-1.,-0.599241616422144));
#28107=CARTESIAN_POINT('Ctrl Pts',(-2.09954930865331,1.,-0.599241616422144));
#28108=CARTESIAN_POINT('Ctrl Pts',(-2.09510876220501,-1.,-0.594585006052823));
#28109=CARTESIAN_POINT('Ctrl Pts',(-2.09510876220501,1.,-0.594585006052823));
#28110=CARTESIAN_POINT('Ctrl Pts',(-2.09064881812053,-1.,-0.589962365403189));
#28111=CARTESIAN_POINT('Ctrl Pts',(-2.09064881812053,1.,-0.589962365403189));
#28112=CARTESIAN_POINT('Ctrl Pts',(-2.086169437277,-1.,-0.585373918990895));
#28113=CARTESIAN_POINT('Ctrl Pts',(-2.086169437277,1.,-0.585373918990895));
#28114=CARTESIAN_POINT('Ctrl Pts',(-2.08167059018138,-1.,-0.580819952107257));
#28115=CARTESIAN_POINT('Ctrl Pts',(-2.08167059018138,1.,-0.580819952107257));
#28116=CARTESIAN_POINT('Ctrl Pts',(-2.07715226767361,-1.,-0.576300797416274));
#28117=CARTESIAN_POINT('Ctrl Pts',(-2.07715226767361,1.,-0.576300797416274));
#28118=CARTESIAN_POINT('Ctrl Pts',(-2.07261449292757,-1.,-0.571816823242411));
#28119=CARTESIAN_POINT('Ctrl Pts',(-2.07261449292757,1.,-0.571816823242411));
#28120=CARTESIAN_POINT('Ctrl Pts',(-2.06805732997383,-1.,-0.567368421181229));
#28121=CARTESIAN_POINT('Ctrl Pts',(-2.06805732997383,1.,-0.567368421181229));
#28122=CARTESIAN_POINT('Ctrl Pts',(-2.06348090160697,-1.,-0.562955993082574));
#28123=CARTESIAN_POINT('Ctrl Pts',(-2.06348090160697,1.,-0.562955993082574));
#28124=CARTESIAN_POINT('Ctrl Pts',(-2.05888537756571,-1.,-0.558579940185467));
#28125=CARTESIAN_POINT('Ctrl Pts',(-2.05888537756571,1.,-0.558579940185467));
#28126=CARTESIAN_POINT('Ctrl Pts',(-2.05427091604482,-1.,-0.554240657464109));
#28127=CARTESIAN_POINT('Ctrl Pts',(-2.05427091604482,1.,-0.554240657464109));
#28128=CARTESIAN_POINT('Ctrl Pts',(-2.04963761077974,-1.,-0.549938525150342));
#28129=CARTESIAN_POINT('Ctrl Pts',(-2.04963761077974,1.,-0.549938525150342));
#28130=CARTESIAN_POINT('Ctrl Pts',(-2.0449854471456,-1.,-0.545673903817348));
#28131=CARTESIAN_POINT('Ctrl Pts',(-2.0449854471456,1.,-0.545673903817348));
#28132=CARTESIAN_POINT('Ctrl Pts',(-2.0403142269048,-1.,-0.54144712061552));
#28133=CARTESIAN_POINT('Ctrl Pts',(-2.0403142269048,1.,-0.54144712061552));
#28134=CARTESIAN_POINT('Ctrl Pts',(-2.03562362953993,-1.,-0.537258489833134));
#28135=CARTESIAN_POINT('Ctrl Pts',(-2.03562362953993,1.,-0.537258489833134));
#28136=CARTESIAN_POINT('Ctrl Pts',(-2.03091336214401,-1.,-0.533108355132905));
#28137=CARTESIAN_POINT('Ctrl Pts',(-2.03091336214401,1.,-0.533108355132905));
#28138=CARTESIAN_POINT('Ctrl Pts',(-2.02618329083289,-1.,-0.52899712724191));
#28139=CARTESIAN_POINT('Ctrl Pts',(-2.02618329083289,1.,-0.52899712724191));
#28140=CARTESIAN_POINT('Ctrl Pts',(-2.02143356304712,-1.,-0.524925318333518));
#28141=CARTESIAN_POINT('Ctrl Pts',(-2.02143356304712,1.,-0.524925318333518));
#28142=CARTESIAN_POINT('Ctrl Pts',(-2.01666477917305,-1.,-0.520893590399428));
#28143=CARTESIAN_POINT('Ctrl Pts',(-2.01666477917305,1.,-0.520893590399428));
#28144=CARTESIAN_POINT('Ctrl Pts',(-2.01187773939257,-1.,-0.516902681728733));
#28145=CARTESIAN_POINT('Ctrl Pts',(-2.01187773939257,1.,-0.516902681728733));
#28146=CARTESIAN_POINT('Ctrl Pts',(-2.00707309946955,-1.,-0.512953306961813));
#28147=CARTESIAN_POINT('Ctrl Pts',(-2.00707309946955,1.,-0.512953306961813));
#28148=CARTESIAN_POINT('Ctrl Pts',(-2.00225107134733,-1.,-0.509046069886152));
#28149=CARTESIAN_POINT('Ctrl Pts',(-2.00225107134733,1.,-0.509046069886152));
#28150=CARTESIAN_POINT('Ctrl Pts',(-1.99741107463567,-1.,-0.505181361323011));
#28151=CARTESIAN_POINT('Ctrl Pts',(-1.99741107463567,1.,-0.505181361323011));
#28152=CARTESIAN_POINT('Ctrl Pts',(-1.9925514912615,-1.,-0.501359287727129));
#28153=CARTESIAN_POINT('Ctrl Pts',(-1.9925514912615,1.,-0.501359287727129));
#28154=CARTESIAN_POINT('Ctrl Pts',(-1.98767044752929,-1.,-0.497579909545564));
#28155=CARTESIAN_POINT('Ctrl Pts',(-1.98767044752929,1.,-0.497579909545564));
#28156=CARTESIAN_POINT('Ctrl Pts',(-1.9827665876182,-1.,-0.493843476541492));
#28157=CARTESIAN_POINT('Ctrl Pts',(-1.9827665876182,1.,-0.493843476541492));
#28158=CARTESIAN_POINT('Ctrl Pts',(-1.97783973019229,-1.,-0.490150627860955));
#28159=CARTESIAN_POINT('Ctrl Pts',(-1.97783973019229,1.,-0.490150627860955));
#28160=CARTESIAN_POINT('Ctrl Pts',(-1.97289186263272,-1.,-0.486502692907661));
#28161=CARTESIAN_POINT('Ctrl Pts',(-1.97289186263272,1.,-0.486502692907661));
#28162=CARTESIAN_POINT('Ctrl Pts',(-1.96792703422358,-1.,-0.482901662120686));
#28163=CARTESIAN_POINT('Ctrl Pts',(-1.96792703422358,1.,-0.482901662120686));
#28164=CARTESIAN_POINT('Ctrl Pts',(-1.96294933055938,-1.,-0.479349583074846));
#28165=CARTESIAN_POINT('Ctrl Pts',(-1.96294933055938,1.,-0.479349583074846));
#28166=CARTESIAN_POINT('Ctrl Pts',(-1.95796111148175,-1.,-0.475848034683171));
#28167=CARTESIAN_POINT('Ctrl Pts',(-1.95796111148175,1.,-0.475848034683171));
#28168=CARTESIAN_POINT('Ctrl Pts',(-1.95296148278136,-1.,-0.472397672264079));
#28169=CARTESIAN_POINT('Ctrl Pts',(-1.95296148278136,1.,-0.472397672264079));
#28170=CARTESIAN_POINT('Ctrl Pts',(-1.94794381136524,-1.,-0.468997482913158));
#28171=CARTESIAN_POINT('Ctrl Pts',(-1.94794381136524,1.,-0.468997482913158));
#28172=CARTESIAN_POINT('Ctrl Pts',(-1.94289794196205,-1.,-0.465645462026064));
#28173=CARTESIAN_POINT('Ctrl Pts',(-1.94289794196205,1.,-0.465645462026064));
#28174=CARTESIAN_POINT('Ctrl Pts',(-1.93781486640834,-1.,-0.462340031009087));
#28175=CARTESIAN_POINT('Ctrl Pts',(-1.93781486640834,1.,-0.462340031009087));
#28176=CARTESIAN_POINT('Ctrl Pts',(-1.93269066517936,-1.,-0.459081234547931));
#28177=CARTESIAN_POINT('Ctrl Pts',(-1.93269066517936,1.,-0.459081234547931));
#28178=CARTESIAN_POINT('Ctrl Pts',(-1.92753067150461,-1.,-0.455872005174335));
#28179=CARTESIAN_POINT('Ctrl Pts',(-1.92753067150461,1.,-0.455872005174335));
#28180=CARTESIAN_POINT('Ctrl Pts',(-1.9223538064847,-1.,-0.452719478359356));
#28181=CARTESIAN_POINT('Ctrl Pts',(-1.9223538064847,1.,-0.452719478359356));
#28182=CARTESIAN_POINT('Ctrl Pts',(-1.91718342555717,-1.,-0.449632260106572));
#28183=CARTESIAN_POINT('Ctrl Pts',(-1.91718342555717,1.,-0.449632260106572));
#28184=CARTESIAN_POINT('Ctrl Pts',(-1.91203699981095,-1.,-0.446617343485651));
#28185=CARTESIAN_POINT('Ctrl Pts',(-1.91203699981095,1.,-0.446617343485651));
#28186=CARTESIAN_POINT('Ctrl Pts',(-1.90691756144906,-1.,-0.44367755684917));
#28187=CARTESIAN_POINT('Ctrl Pts',(-1.90691756144906,1.,-0.44367755684917));
#28188=CARTESIAN_POINT('Ctrl Pts',(-1.90180124389137,-1.,-0.44080783370416));
#28189=CARTESIAN_POINT('Ctrl Pts',(-1.90180124389137,1.,-0.44080783370416));
#28190=CARTESIAN_POINT('Ctrl Pts',(-1.89663648956549,-1.,-0.437995003948443));
#28191=CARTESIAN_POINT('Ctrl Pts',(-1.89663648956549,1.,-0.437995003948443));
#28192=CARTESIAN_POINT('Ctrl Pts',(-1.89136993975585,-1.,-0.43522566096358));
#28193=CARTESIAN_POINT('Ctrl Pts',(-1.89136993975585,1.,-0.43522566096358));
#28194=CARTESIAN_POINT('Ctrl Pts',(-1.88596913666828,-1.,-0.432493038548833));
#28195=CARTESIAN_POINT('Ctrl Pts',(-1.88596913666828,1.,-0.432493038548833));
#28196=CARTESIAN_POINT('Ctrl Pts',(-1.88044229001778,-1.,-0.429803062482217));
#28197=CARTESIAN_POINT('Ctrl Pts',(-1.88044229001778,1.,-0.429803062482217));
#28198=CARTESIAN_POINT('Ctrl Pts',(-1.87486989291333,-1.,-0.427183828518743));
#28199=CARTESIAN_POINT('Ctrl Pts',(-1.87486989291333,1.,-0.427183828518743));
#28200=CARTESIAN_POINT('Ctrl Pts',(-1.8693780394412,-1.,-0.424678177290876));
#28201=CARTESIAN_POINT('Ctrl Pts',(-1.8693780394412,1.,-0.424678177290876));
#28202=CARTESIAN_POINT('Ctrl Pts',(-1.86408083333863,-1.,-0.422327307417884));
#28203=CARTESIAN_POINT('Ctrl Pts',(-1.86408083333863,1.,-0.422327307417884));
#28204=CARTESIAN_POINT('Ctrl Pts',(-1.8590328109667,-1.,-0.420157287975583));
#28205=CARTESIAN_POINT('Ctrl Pts',(-1.8590328109667,1.,-0.420157287975583));
#28206=CARTESIAN_POINT('Ctrl Pts',(-1.8541763285645,-1.,-0.418164129144045));
#28207=CARTESIAN_POINT('Ctrl Pts',(-1.8541763285645,1.,-0.418164129144045));
#28208=CARTESIAN_POINT('Ctrl Pts',(-1.84929312930314,-1.,-0.416300022039885));
#28209=CARTESIAN_POINT('Ctrl Pts',(-1.84929312930314,1.,-0.416300022039885));
#28210=CARTESIAN_POINT('Ctrl Pts',(-1.84405757074218,-1.,-0.414487438255542));
#28211=CARTESIAN_POINT('Ctrl Pts',(-1.84405757074218,1.,-0.414487438255542));
#28212=CARTESIAN_POINT('Ctrl Pts',(-1.8380895347617,-1.,-0.412633125322945));
#28213=CARTESIAN_POINT('Ctrl Pts',(-1.8380895347617,1.,-0.412633125322945));
#28214=CARTESIAN_POINT('Ctrl Pts',(-1.83100408895047,-1.,-0.410641256301276));
#28215=CARTESIAN_POINT('Ctrl Pts',(-1.83100408895047,1.,-0.410641256301276));
#28216=CARTESIAN_POINT('Ctrl Pts',(-1.82247022677562,-1.,-0.408428948106227));
#28217=CARTESIAN_POINT('Ctrl Pts',(-1.82247022677562,1.,-0.408428948106227));
#28218=CARTESIAN_POINT('Ctrl Pts',(-1.81223801812013,-1.,-0.405933518407175));
#28219=CARTESIAN_POINT('Ctrl Pts',(-1.81223801812013,1.,-0.405933518407175));
#28220=CARTESIAN_POINT('Ctrl Pts',(-1.80012077173238,-1.,-0.403107976163396));
#28221=CARTESIAN_POINT('Ctrl Pts',(-1.80012077173238,1.,-0.403107976163396));
#28222=CARTESIAN_POINT('Ctrl Pts',(-1.78598826343754,-1.,-0.399919403774155));
#28223=CARTESIAN_POINT('Ctrl Pts',(-1.78598826343754,1.,-0.399919403774155));
#28224=CARTESIAN_POINT('Ctrl Pts',(-1.76975560043442,-1.,-0.396346196110688));
#28225=CARTESIAN_POINT('Ctrl Pts',(-1.76975560043442,1.,-0.396346196110688));
#28226=CARTESIAN_POINT('Ctrl Pts',(-1.75137405310193,-1.,-0.392375812285395));
#28227=CARTESIAN_POINT('Ctrl Pts',(-1.75137405310193,1.,-0.392375812285395));
#28228=CARTESIAN_POINT('Ctrl Pts',(-1.73493170972829,-1.,-0.388877023502615));
#28229=CARTESIAN_POINT('Ctrl Pts',(-1.73493170972829,1.,-0.388877023502615));
#28230=CARTESIAN_POINT('Ctrl Pts',(-1.72162022244582,-1.,-0.386070790323281));
#28231=CARTESIAN_POINT('Ctrl Pts',(-1.72162022244582,1.,-0.386070790323281));
#28232=CARTESIAN_POINT('Ctrl Pts',(-1.71231062891398,-1.,-0.384119047314215));
#28233=CARTESIAN_POINT('Ctrl Pts',(-1.71231062891398,1.,-0.384119047314215));
#28234=CARTESIAN_POINT('Ctrl Pts',(-1.7075470150345,-1.,-0.383122945602004));
#28235=CARTESIAN_POINT('Ctrl Pts',(-1.7075470150345,1.,-0.383122945602004));
#28236=CARTESIAN_POINT('',(-2.11275013067528,1.,-0.61342227326009));
#28237=CARTESIAN_POINT('Ctrl Pts',(-2.11275013067528,1.,-0.61342227326009));
#28238=CARTESIAN_POINT('Ctrl Pts',(-2.11187554260142,1.,-0.61246736556225));
#28239=CARTESIAN_POINT('Ctrl Pts',(-2.11012443807661,1.,-0.610560911691113));
#28240=CARTESIAN_POINT('Ctrl Pts',(-2.10749199615859,1.,-0.607711315456826));
#28241=CARTESIAN_POINT('Ctrl Pts',(-2.10397049887709,1.,-0.603932030738212));
#28242=CARTESIAN_POINT('Ctrl Pts',(-2.09954930865331,1.,-0.599241616422144));
#28243=CARTESIAN_POINT('Ctrl Pts',(-2.09510876220501,1.,-0.594585006052823));
#28244=CARTESIAN_POINT('Ctrl Pts',(-2.09064881812053,1.,-0.589962365403189));
#28245=CARTESIAN_POINT('Ctrl Pts',(-2.086169437277,1.,-0.585373918990895));
#28246=CARTESIAN_POINT('Ctrl Pts',(-2.08167059018138,1.,-0.580819952107257));
#28247=CARTESIAN_POINT('Ctrl Pts',(-2.07715226767361,1.,-0.576300797416274));
#28248=CARTESIAN_POINT('Ctrl Pts',(-2.07261449292757,1.,-0.571816823242411));
#28249=CARTESIAN_POINT('Ctrl Pts',(-2.06805732997383,1.,-0.567368421181229));
#28250=CARTESIAN_POINT('Ctrl Pts',(-2.06348090160697,1.,-0.562955993082574));
#28251=CARTESIAN_POINT('Ctrl Pts',(-2.05888537756571,1.,-0.558579940185467));
#28252=CARTESIAN_POINT('Ctrl Pts',(-2.05427091604482,1.,-0.554240657464109));
#28253=CARTESIAN_POINT('Ctrl Pts',(-2.04963761077974,1.,-0.549938525150342));
#28254=CARTESIAN_POINT('Ctrl Pts',(-2.0449854471456,1.,-0.545673903817348));
#28255=CARTESIAN_POINT('Ctrl Pts',(-2.0403142269048,1.,-0.54144712061552));
#28256=CARTESIAN_POINT('Ctrl Pts',(-2.03562362953993,1.,-0.537258489833134));
#28257=CARTESIAN_POINT('Ctrl Pts',(-2.03091336214401,1.,-0.533108355132905));
#28258=CARTESIAN_POINT('Ctrl Pts',(-2.02618329083289,1.,-0.52899712724191));
#28259=CARTESIAN_POINT('Ctrl Pts',(-2.02143356304712,1.,-0.524925318333518));
#28260=CARTESIAN_POINT('Ctrl Pts',(-2.01666477917305,1.,-0.520893590399428));
#28261=CARTESIAN_POINT('Ctrl Pts',(-2.01187773939257,1.,-0.516902681728733));
#28262=CARTESIAN_POINT('Ctrl Pts',(-2.00707309946955,1.,-0.512953306961813));
#28263=CARTESIAN_POINT('Ctrl Pts',(-2.00225107134733,1.,-0.509046069886152));
#28264=CARTESIAN_POINT('Ctrl Pts',(-1.99741107463567,1.,-0.505181361323011));
#28265=CARTESIAN_POINT('Ctrl Pts',(-1.9925514912615,1.,-0.501359287727129));
#28266=CARTESIAN_POINT('Ctrl Pts',(-1.98767044752929,1.,-0.497579909545564));
#28267=CARTESIAN_POINT('Ctrl Pts',(-1.9827665876182,1.,-0.493843476541492));
#28268=CARTESIAN_POINT('Ctrl Pts',(-1.97783973019229,1.,-0.490150627860955));
#28269=CARTESIAN_POINT('Ctrl Pts',(-1.97289186263272,1.,-0.486502692907661));
#28270=CARTESIAN_POINT('Ctrl Pts',(-1.96792703422358,1.,-0.482901662120686));
#28271=CARTESIAN_POINT('Ctrl Pts',(-1.96294933055938,1.,-0.479349583074846));
#28272=CARTESIAN_POINT('Ctrl Pts',(-1.95796111148175,1.,-0.475848034683171));
#28273=CARTESIAN_POINT('Ctrl Pts',(-1.95296148278136,1.,-0.472397672264079));
#28274=CARTESIAN_POINT('Ctrl Pts',(-1.94794381136524,1.,-0.468997482913158));
#28275=CARTESIAN_POINT('Ctrl Pts',(-1.94289794196205,1.,-0.465645462026064));
#28276=CARTESIAN_POINT('Ctrl Pts',(-1.93781486640834,1.,-0.462340031009087));
#28277=CARTESIAN_POINT('Ctrl Pts',(-1.93269066517936,1.,-0.459081234547931));
#28278=CARTESIAN_POINT('Ctrl Pts',(-1.92753067150461,1.,-0.455872005174335));
#28279=CARTESIAN_POINT('Ctrl Pts',(-1.9223538064847,1.,-0.452719478359356));
#28280=CARTESIAN_POINT('Ctrl Pts',(-1.91718342555717,1.,-0.449632260106572));
#28281=CARTESIAN_POINT('Ctrl Pts',(-1.91203699981095,1.,-0.446617343485651));
#28282=CARTESIAN_POINT('Ctrl Pts',(-1.90691756144906,1.,-0.44367755684917));
#28283=CARTESIAN_POINT('Ctrl Pts',(-1.90180124389137,1.,-0.44080783370416));
#28284=CARTESIAN_POINT('Ctrl Pts',(-1.89663648956549,1.,-0.437995003948443));
#28285=CARTESIAN_POINT('Ctrl Pts',(-1.89136993975585,1.,-0.43522566096358));
#28286=CARTESIAN_POINT('Ctrl Pts',(-1.88596913666828,1.,-0.432493038548833));
#28287=CARTESIAN_POINT('Ctrl Pts',(-1.88044229001778,1.,-0.429803062482217));
#28288=CARTESIAN_POINT('Ctrl Pts',(-1.87486989291333,1.,-0.427183828518743));
#28289=CARTESIAN_POINT('Ctrl Pts',(-1.8693780394412,1.,-0.424678177290876));
#28290=CARTESIAN_POINT('Ctrl Pts',(-1.86408083333863,1.,-0.422327307417884));
#28291=CARTESIAN_POINT('Ctrl Pts',(-1.8590328109667,1.,-0.420157287975583));
#28292=CARTESIAN_POINT('Ctrl Pts',(-1.8541763285645,1.,-0.418164129144045));
#28293=CARTESIAN_POINT('Ctrl Pts',(-1.84929312930314,1.,-0.416300022039885));
#28294=CARTESIAN_POINT('Ctrl Pts',(-1.84405757074218,1.,-0.414487438255542));
#28295=CARTESIAN_POINT('Ctrl Pts',(-1.8380895347617,1.,-0.412633125322945));
#28296=CARTESIAN_POINT('Ctrl Pts',(-1.83100408895047,1.,-0.410641256301276));
#28297=CARTESIAN_POINT('Ctrl Pts',(-1.82247022677562,1.,-0.408428948106227));
#28298=CARTESIAN_POINT('Ctrl Pts',(-1.81223801812013,1.,-0.405933518407175));
#28299=CARTESIAN_POINT('Ctrl Pts',(-1.80012077173238,1.,-0.403107976163396));
#28300=CARTESIAN_POINT('Ctrl Pts',(-1.78598826343754,1.,-0.399919403774155));
#28301=CARTESIAN_POINT('Ctrl Pts',(-1.76975560043442,1.,-0.396346196110688));
#28302=CARTESIAN_POINT('Ctrl Pts',(-1.75137405310193,1.,-0.392375812285395));
#28303=CARTESIAN_POINT('Ctrl Pts',(-1.73493170972829,1.,-0.388877023502615));
#28304=CARTESIAN_POINT('Ctrl Pts',(-1.72162022244582,1.,-0.386070790323281));
#28305=CARTESIAN_POINT('Ctrl Pts',(-1.71231062891398,1.,-0.384119047314215));
#28306=CARTESIAN_POINT('Ctrl Pts',(-1.7075470150345,1.,-0.383122945602004));
#28307=CARTESIAN_POINT('',(-2.11275013067528,0.,-0.61342227326009));
#28308=CARTESIAN_POINT('Origin',(-2.0698113262342,0.,-0.745574324794401));
#28309=CARTESIAN_POINT('',(-2.0698113262342,1.,-0.745574324794401));
#28310=CARTESIAN_POINT('',(-2.11275013067528,1.,-0.61342227326009));
#28311=CARTESIAN_POINT('',(-2.0698113262342,0.,-0.745574324794401));
#28312=CARTESIAN_POINT('Ctrl Pts',(-1.60662857109684,-1.,-0.693717979106306));
#28313=CARTESIAN_POINT('Ctrl Pts',(-1.60662857109684,1.,-0.693717979106306));
#28314=CARTESIAN_POINT('Ctrl Pts',(-1.61106790958151,-1.,-0.695712097881194));
#28315=CARTESIAN_POINT('Ctrl Pts',(-1.61106790958151,1.,-0.695712097881194));
#28316=CARTESIAN_POINT('Ctrl Pts',(-1.61974673472612,-1.,-0.699605146405088));
#28317=CARTESIAN_POINT('Ctrl Pts',(-1.61974673472612,1.,-0.699605146405088));
#28318=CARTESIAN_POINT('Ctrl Pts',(-1.63216541664676,-1.,-0.705159151988319));
#28319=CARTESIAN_POINT('Ctrl Pts',(-1.63216541664676,1.,-0.705159151988319));
#28320=CARTESIAN_POINT('Ctrl Pts',(-1.64752408832016,-1.,-0.711993139355394));
#28321=CARTESIAN_POINT('Ctrl Pts',(-1.64752408832016,1.,-0.711993139355394));
#28322=CARTESIAN_POINT('Ctrl Pts',(-1.6647288055568,-1.,-0.719585433804282));
#28323=CARTESIAN_POINT('Ctrl Pts',(-1.6647288055568,1.,-0.719585433804282));
#28324=CARTESIAN_POINT('Ctrl Pts',(-1.67996158455503,-1.,-0.726235967997433));
#28325=CARTESIAN_POINT('Ctrl Pts',(-1.67996158455503,1.,-0.726235967997433));
#28326=CARTESIAN_POINT('Ctrl Pts',(-1.69326921975743,-1.,-0.731963238697195));
#28327=CARTESIAN_POINT('Ctrl Pts',(-1.69326921975743,1.,-0.731963238697195));
#28328=CARTESIAN_POINT('Ctrl Pts',(-1.70473309006121,-1.,-0.736799665724771));
#28329=CARTESIAN_POINT('Ctrl Pts',(-1.70473309006121,1.,-0.736799665724771));
#28330=CARTESIAN_POINT('Ctrl Pts',(-1.71447789751927,-1.,-0.740795162032087));
#28331=CARTESIAN_POINT('Ctrl Pts',(-1.71447789751927,1.,-0.740795162032087));
#28332=CARTESIAN_POINT('Ctrl Pts',(-1.7226822991693,-1.,-0.744021445433764));
#28333=CARTESIAN_POINT('Ctrl Pts',(-1.7226822991693,1.,-0.744021445433764));
#28334=CARTESIAN_POINT('Ctrl Pts',(-1.72958533647399,-1.,-0.746574710096436));
#28335=CARTESIAN_POINT('Ctrl Pts',(-1.72958533647399,1.,-0.746574710096436));
#28336=CARTESIAN_POINT('Ctrl Pts',(-1.73550351679848,-1.,-0.748582462954854));
#28337=CARTESIAN_POINT('Ctrl Pts',(-1.73550351679848,1.,-0.748582462954854));
#28338=CARTESIAN_POINT('Ctrl Pts',(-1.74080458266705,-1.,-0.75019343597954));
#28339=CARTESIAN_POINT('Ctrl Pts',(-1.74080458266705,1.,-0.75019343597954));
#28340=CARTESIAN_POINT('Ctrl Pts',(-1.74585086852298,-1.,-0.751555614163629));
#28341=CARTESIAN_POINT('Ctrl Pts',(-1.74585086852298,1.,-0.751555614163629));
#28342=CARTESIAN_POINT('Ctrl Pts',(-1.75095139468809,-1.,-0.752797683531377));
#28343=CARTESIAN_POINT('Ctrl Pts',(-1.75095139468809,1.,-0.752797683531377));
#28344=CARTESIAN_POINT('Ctrl Pts',(-1.75631083600175,-1.,-0.75400925402848));
#28345=CARTESIAN_POINT('Ctrl Pts',(-1.75631083600175,1.,-0.75400925402848));
#28346=CARTESIAN_POINT('Ctrl Pts',(-1.7619781724032,-1.,-0.755220979975262));
#28347=CARTESIAN_POINT('Ctrl Pts',(-1.7619781724032,1.,-0.755220979975262));
#28348=CARTESIAN_POINT('Ctrl Pts',(-1.76789396003141,-1.,-0.756421896028403));
#28349=CARTESIAN_POINT('Ctrl Pts',(-1.76789396003141,1.,-0.756421896028403));
#28350=CARTESIAN_POINT('Ctrl Pts',(-1.77394167108342,-1.,-0.757578264077238));
#28351=CARTESIAN_POINT('Ctrl Pts',(-1.77394167108342,1.,-0.757578264077238));
#28352=CARTESIAN_POINT('Ctrl Pts',(-1.77999411220912,-1.,-0.75865062667738));
#28353=CARTESIAN_POINT('Ctrl Pts',(-1.77999411220912,1.,-0.75865062667738));
#28354=CARTESIAN_POINT('Ctrl Pts',(-1.78596964884526,-1.,-0.759614401109868));
#28355=CARTESIAN_POINT('Ctrl Pts',(-1.78596964884526,1.,-0.759614401109868));
#28356=CARTESIAN_POINT('Ctrl Pts',(-1.79185815610802,-1.,-0.760469555880425));
#28357=CARTESIAN_POINT('Ctrl Pts',(-1.79185815610802,1.,-0.760469555880425));
#28358=CARTESIAN_POINT('Ctrl Pts',(-1.79768986997735,-1.,-0.761229695230359));
#28359=CARTESIAN_POINT('Ctrl Pts',(-1.79768986997735,1.,-0.761229695230359));
#28360=CARTESIAN_POINT('Ctrl Pts',(-1.80351583877334,-1.,-0.761915336443515));
#28361=CARTESIAN_POINT('Ctrl Pts',(-1.80351583877334,1.,-0.761915336443515));
#28362=CARTESIAN_POINT('Ctrl Pts',(-1.80938551463989,-1.,-0.762546129464036));
#28363=CARTESIAN_POINT('Ctrl Pts',(-1.80938551463989,1.,-0.762546129464036));
#28364=CARTESIAN_POINT('Ctrl Pts',(-1.81532118405566,-1.,-0.763132003836783));
#28365=CARTESIAN_POINT('Ctrl Pts',(-1.81532118405566,1.,-0.763132003836783));
#28366=CARTESIAN_POINT('Ctrl Pts',(-1.82131873145297,-1.,-0.763673465462854));
#28367=CARTESIAN_POINT('Ctrl Pts',(-1.82131873145297,1.,-0.763673465462854));
#28368=CARTESIAN_POINT('Ctrl Pts',(-1.8273599120008,-1.,-0.764165902606055));
#28369=CARTESIAN_POINT('Ctrl Pts',(-1.8273599120008,1.,-0.764165902606055));
#28370=CARTESIAN_POINT('Ctrl Pts',(-1.8334207722714,-1.,-0.764602549687845));
#28371=CARTESIAN_POINT('Ctrl Pts',(-1.8334207722714,1.,-0.764602549687845));
#28372=CARTESIAN_POINT('Ctrl Pts',(-1.83948181064823,-1.,-0.764978057881687));
#28373=CARTESIAN_POINT('Ctrl Pts',(-1.83948181064823,1.,-0.764978057881687));
#28374=CARTESIAN_POINT('Ctrl Pts',(-1.8455369887591,-1.,-0.765291664861971));
#28375=CARTESIAN_POINT('Ctrl Pts',(-1.8455369887591,1.,-0.765291664861971));
#28376=CARTESIAN_POINT('Ctrl Pts',(-1.85158945130054,-1.,-0.765545710619023));
#28377=CARTESIAN_POINT('Ctrl Pts',(-1.85158945130054,1.,-0.765545710619023));
#28378=CARTESIAN_POINT('Ctrl Pts',(-1.85764741390391,-1.,-0.765744212909305));
#28379=CARTESIAN_POINT('Ctrl Pts',(-1.85764741390391,1.,-0.765744212909305));
#28380=CARTESIAN_POINT('Ctrl Pts',(-1.86372027063314,-1.,-0.765891519092557));
#28381=CARTESIAN_POINT('Ctrl Pts',(-1.86372027063314,1.,-0.765891519092557));
#28382=CARTESIAN_POINT('Ctrl Pts',(-1.86981398314345,-1.,-0.765990708546111));
#28383=CARTESIAN_POINT('Ctrl Pts',(-1.86981398314345,1.,-0.765990708546111));
#28384=CARTESIAN_POINT('Ctrl Pts',(-1.87592888967886,-1.,-0.766042837036759));
#28385=CARTESIAN_POINT('Ctrl Pts',(-1.87592888967886,1.,-0.766042837036759));
#28386=CARTESIAN_POINT('Ctrl Pts',(-1.88206215302561,-1.,-0.766047794851868));
#28387=CARTESIAN_POINT('Ctrl Pts',(-1.88206215302561,1.,-0.766047794851868));
#28388=CARTESIAN_POINT('Ctrl Pts',(-1.88820926433409,-1.,-0.76600483706209));
#28389=CARTESIAN_POINT('Ctrl Pts',(-1.88820926433409,1.,-0.76600483706209));
#28390=CARTESIAN_POINT('Ctrl Pts',(-1.89436577771389,-1.,-0.765913193856979));
#28391=CARTESIAN_POINT('Ctrl Pts',(-1.89436577771389,1.,-0.765913193856979));
#28392=CARTESIAN_POINT('Ctrl Pts',(-1.90052930393599,-1.,-0.765772772593395));
#28393=CARTESIAN_POINT('Ctrl Pts',(-1.90052930393599,1.,-0.765772772593395));
#28394=CARTESIAN_POINT('Ctrl Pts',(-1.90669961402362,-1.,-0.765584196937936));
#28395=CARTESIAN_POINT('Ctrl Pts',(-1.90669961402362,1.,-0.765584196937936));
#28396=CARTESIAN_POINT('Ctrl Pts',(-1.91287765805174,-1.,-0.765348465884739));
#28397=CARTESIAN_POINT('Ctrl Pts',(-1.91287765805174,1.,-0.765348465884739));
#28398=CARTESIAN_POINT('Ctrl Pts',(-1.91906491634197,-1.,-0.765066729667095));
#28399=CARTESIAN_POINT('Ctrl Pts',(-1.91906491634197,1.,-0.765066729667095));
#28400=CARTESIAN_POINT('Ctrl Pts',(-1.92526263537041,-1.,-0.764740025488189));
#28401=CARTESIAN_POINT('Ctrl Pts',(-1.92526263537041,1.,-0.764740025488189));
#28402=CARTESIAN_POINT('Ctrl Pts',(-1.93147105496367,-1.,-0.764369010673889));
#28403=CARTESIAN_POINT('Ctrl Pts',(-1.93147105496367,1.,-0.764369010673889));
#28404=CARTESIAN_POINT('Ctrl Pts',(-1.93768964875867,-1.,-0.763954049121393));
#28405=CARTESIAN_POINT('Ctrl Pts',(-1.93768964875867,1.,-0.763954049121393));
#28406=CARTESIAN_POINT('Ctrl Pts',(-1.94391746617626,-1.,-0.76349533353858));
#28407=CARTESIAN_POINT('Ctrl Pts',(-1.94391746617626,1.,-0.76349533353858));
#28408=CARTESIAN_POINT('Ctrl Pts',(-1.95015342590025,-1.,-0.762992990878774));
#28409=CARTESIAN_POINT('Ctrl Pts',(-1.95015342590025,1.,-0.762992990878774));
#28410=CARTESIAN_POINT('Ctrl Pts',(-1.95639665309893,-1.,-0.762447203806263));
#28411=CARTESIAN_POINT('Ctrl Pts',(-1.95639665309893,1.,-0.762447203806263));
#28412=CARTESIAN_POINT('Ctrl Pts',(-1.96264672744229,-1.,-0.761858300014575));
#28413=CARTESIAN_POINT('Ctrl Pts',(-1.96264672744229,1.,-0.761858300014575));
#28414=CARTESIAN_POINT('Ctrl Pts',(-1.96890351582545,-1.,-0.761226690483986));
#28415=CARTESIAN_POINT('Ctrl Pts',(-1.96890351582545,1.,-0.761226690483986));
#28416=CARTESIAN_POINT('Ctrl Pts',(-1.97516705321521,-1.,-0.760552825409855));
#28417=CARTESIAN_POINT('Ctrl Pts',(-1.97516705321521,1.,-0.760552825409855));
#28418=CARTESIAN_POINT('Ctrl Pts',(-1.98143741418156,-1.,-0.759837147452135));
#28419=CARTESIAN_POINT('Ctrl Pts',(-1.98143741418156,1.,-0.759837147452135));
#28420=CARTESIAN_POINT('Ctrl Pts',(-1.98771456680806,-1.,-0.759080037802242));
#28421=CARTESIAN_POINT('Ctrl Pts',(-1.98771456680806,1.,-0.759080037802242));
#28422=CARTESIAN_POINT('Ctrl Pts',(-1.9939983109871,-1.,-0.758281796766377));
#28423=CARTESIAN_POINT('Ctrl Pts',(-1.9939983109871,1.,-0.758281796766377));
#28424=CARTESIAN_POINT('Ctrl Pts',(-2.00028834739072,-1.,-0.757442676862341));
#28425=CARTESIAN_POINT('Ctrl Pts',(-2.00028834739072,1.,-0.757442676862341));
#28426=CARTESIAN_POINT('Ctrl Pts',(-2.00658431587682,-1.,-0.756562904646496));
#28427=CARTESIAN_POINT('Ctrl Pts',(-2.00658431587682,1.,-0.756562904646496));
#28428=CARTESIAN_POINT('Ctrl Pts',(-2.01288584328149,-1.,-0.7556427049581));
#28429=CARTESIAN_POINT('Ctrl Pts',(-2.01288584328149,1.,-0.7556427049581));
#28430=CARTESIAN_POINT('Ctrl Pts',(-2.01919259406003,-1.,-0.75468233072352));
#28431=CARTESIAN_POINT('Ctrl Pts',(-2.01919259406003,1.,-0.75468233072352));
#28432=CARTESIAN_POINT('Ctrl Pts',(-2.02550428623587,-1.,-0.753682061113765));
#28433=CARTESIAN_POINT('Ctrl Pts',(-2.02550428623587,1.,-0.753682061113765));
#28434=CARTESIAN_POINT('Ctrl Pts',(-2.03182068456467,-1.,-0.752642180488104));
#28435=CARTESIAN_POINT('Ctrl Pts',(-2.03182068456467,1.,-0.752642180488104));
#28436=CARTESIAN_POINT('Ctrl Pts',(-2.03814160092173,-1.,-0.751562963361383));
#28437=CARTESIAN_POINT('Ctrl Pts',(-2.03814160092173,1.,-0.751562963361383));
#28438=CARTESIAN_POINT('Ctrl Pts',(-2.04446689147754,-1.,-0.750444657874758));
#28439=CARTESIAN_POINT('Ctrl Pts',(-2.04446689147754,1.,-0.750444657874758));
#28440=CARTESIAN_POINT('Ctrl Pts',(-2.05079645591606,-1.,-0.749287468663053));
#28441=CARTESIAN_POINT('Ctrl Pts',(-2.05079645591606,1.,-0.749287468663053));
#28442=CARTESIAN_POINT('Ctrl Pts',(-2.05713023030263,-1.,-0.748091554181101));
#28443=CARTESIAN_POINT('Ctrl Pts',(-2.05713023030263,1.,-0.748091554181101));
#28444=CARTESIAN_POINT('Ctrl Pts',(-2.06220058927162,-1.,-0.747103932785504));
#28445=CARTESIAN_POINT('Ctrl Pts',(-2.06220058927162,1.,-0.747103932785504));
#28446=CARTESIAN_POINT('Ctrl Pts',(-2.06600523016401,-1.,-0.746345871542695));
#28447=CARTESIAN_POINT('Ctrl Pts',(-2.06600523016401,1.,-0.746345871542695));
#28448=CARTESIAN_POINT('Ctrl Pts',(-2.06854248895575,-1.,-0.74583279137781));
#28449=CARTESIAN_POINT('Ctrl Pts',(-2.06854248895575,1.,-0.74583279137781));
#28450=CARTESIAN_POINT('Ctrl Pts',(-2.0698113262342,-1.,-0.745574324794401));
#28451=CARTESIAN_POINT('Ctrl Pts',(-2.0698113262342,1.,-0.745574324794401));
#28452=CARTESIAN_POINT('',(-1.60662857109684,1.,-0.693717979106306));
#28453=CARTESIAN_POINT('Ctrl Pts',(-1.60662857109684,1.,-0.693717979106306));
#28454=CARTESIAN_POINT('Ctrl Pts',(-1.61106790958151,1.,-0.695712097881194));
#28455=CARTESIAN_POINT('Ctrl Pts',(-1.61974673472612,1.,-0.699605146405088));
#28456=CARTESIAN_POINT('Ctrl Pts',(-1.63216541664676,1.,-0.705159151988319));
#28457=CARTESIAN_POINT('Ctrl Pts',(-1.64752408832016,1.,-0.711993139355394));
#28458=CARTESIAN_POINT('Ctrl Pts',(-1.6647288055568,1.,-0.719585433804282));
#28459=CARTESIAN_POINT('Ctrl Pts',(-1.67996158455503,1.,-0.726235967997433));
#28460=CARTESIAN_POINT('Ctrl Pts',(-1.69326921975743,1.,-0.731963238697195));
#28461=CARTESIAN_POINT('Ctrl Pts',(-1.70473309006121,1.,-0.736799665724771));
#28462=CARTESIAN_POINT('Ctrl Pts',(-1.71447789751927,1.,-0.740795162032087));
#28463=CARTESIAN_POINT('Ctrl Pts',(-1.7226822991693,1.,-0.744021445433764));
#28464=CARTESIAN_POINT('Ctrl Pts',(-1.72958533647399,1.,-0.746574710096436));
#28465=CARTESIAN_POINT('Ctrl Pts',(-1.73550351679848,1.,-0.748582462954854));
#28466=CARTESIAN_POINT('Ctrl Pts',(-1.74080458266705,1.,-0.75019343597954));
#28467=CARTESIAN_POINT('Ctrl Pts',(-1.74585086852298,1.,-0.751555614163629));
#28468=CARTESIAN_POINT('Ctrl Pts',(-1.75095139468809,1.,-0.752797683531377));
#28469=CARTESIAN_POINT('Ctrl Pts',(-1.75631083600175,1.,-0.75400925402848));
#28470=CARTESIAN_POINT('Ctrl Pts',(-1.7619781724032,1.,-0.755220979975262));
#28471=CARTESIAN_POINT('Ctrl Pts',(-1.76789396003141,1.,-0.756421896028403));
#28472=CARTESIAN_POINT('Ctrl Pts',(-1.77394167108342,1.,-0.757578264077238));
#28473=CARTESIAN_POINT('Ctrl Pts',(-1.77999411220912,1.,-0.75865062667738));
#28474=CARTESIAN_POINT('Ctrl Pts',(-1.78596964884526,1.,-0.759614401109868));
#28475=CARTESIAN_POINT('Ctrl Pts',(-1.79185815610802,1.,-0.760469555880425));
#28476=CARTESIAN_POINT('Ctrl Pts',(-1.79768986997735,1.,-0.761229695230359));
#28477=CARTESIAN_POINT('Ctrl Pts',(-1.80351583877334,1.,-0.761915336443515));
#28478=CARTESIAN_POINT('Ctrl Pts',(-1.80938551463989,1.,-0.762546129464036));
#28479=CARTESIAN_POINT('Ctrl Pts',(-1.81532118405566,1.,-0.763132003836783));
#28480=CARTESIAN_POINT('Ctrl Pts',(-1.82131873145297,1.,-0.763673465462854));
#28481=CARTESIAN_POINT('Ctrl Pts',(-1.8273599120008,1.,-0.764165902606055));
#28482=CARTESIAN_POINT('Ctrl Pts',(-1.8334207722714,1.,-0.764602549687845));
#28483=CARTESIAN_POINT('Ctrl Pts',(-1.83948181064823,1.,-0.764978057881687));
#28484=CARTESIAN_POINT('Ctrl Pts',(-1.8455369887591,1.,-0.765291664861971));
#28485=CARTESIAN_POINT('Ctrl Pts',(-1.85158945130054,1.,-0.765545710619023));
#28486=CARTESIAN_POINT('Ctrl Pts',(-1.85764741390391,1.,-0.765744212909305));
#28487=CARTESIAN_POINT('Ctrl Pts',(-1.86372027063314,1.,-0.765891519092557));
#28488=CARTESIAN_POINT('Ctrl Pts',(-1.86981398314345,1.,-0.765990708546111));
#28489=CARTESIAN_POINT('Ctrl Pts',(-1.87592888967886,1.,-0.766042837036759));
#28490=CARTESIAN_POINT('Ctrl Pts',(-1.88206215302561,1.,-0.766047794851868));
#28491=CARTESIAN_POINT('Ctrl Pts',(-1.88820926433409,1.,-0.76600483706209));
#28492=CARTESIAN_POINT('Ctrl Pts',(-1.89436577771389,1.,-0.765913193856979));
#28493=CARTESIAN_POINT('Ctrl Pts',(-1.90052930393599,1.,-0.765772772593395));
#28494=CARTESIAN_POINT('Ctrl Pts',(-1.90669961402362,1.,-0.765584196937936));
#28495=CARTESIAN_POINT('Ctrl Pts',(-1.91287765805174,1.,-0.765348465884739));
#28496=CARTESIAN_POINT('Ctrl Pts',(-1.91906491634197,1.,-0.765066729667095));
#28497=CARTESIAN_POINT('Ctrl Pts',(-1.92526263537041,1.,-0.764740025488189));
#28498=CARTESIAN_POINT('Ctrl Pts',(-1.93147105496367,1.,-0.764369010673889));
#28499=CARTESIAN_POINT('Ctrl Pts',(-1.93768964875867,1.,-0.763954049121393));
#28500=CARTESIAN_POINT('Ctrl Pts',(-1.94391746617626,1.,-0.76349533353858));
#28501=CARTESIAN_POINT('Ctrl Pts',(-1.95015342590025,1.,-0.762992990878774));
#28502=CARTESIAN_POINT('Ctrl Pts',(-1.95639665309893,1.,-0.762447203806263));
#28503=CARTESIAN_POINT('Ctrl Pts',(-1.96264672744229,1.,-0.761858300014575));
#28504=CARTESIAN_POINT('Ctrl Pts',(-1.96890351582545,1.,-0.761226690483986));
#28505=CARTESIAN_POINT('Ctrl Pts',(-1.97516705321521,1.,-0.760552825409855));
#28506=CARTESIAN_POINT('Ctrl Pts',(-1.98143741418156,1.,-0.759837147452135));
#28507=CARTESIAN_POINT('Ctrl Pts',(-1.98771456680806,1.,-0.759080037802242));
#28508=CARTESIAN_POINT('Ctrl Pts',(-1.9939983109871,1.,-0.758281796766377));
#28509=CARTESIAN_POINT('Ctrl Pts',(-2.00028834739072,1.,-0.757442676862341));
#28510=CARTESIAN_POINT('Ctrl Pts',(-2.00658431587682,1.,-0.756562904646496));
#28511=CARTESIAN_POINT('Ctrl Pts',(-2.01288584328149,1.,-0.7556427049581));
#28512=CARTESIAN_POINT('Ctrl Pts',(-2.01919259406003,1.,-0.75468233072352));
#28513=CARTESIAN_POINT('Ctrl Pts',(-2.02550428623587,1.,-0.753682061113765));
#28514=CARTESIAN_POINT('Ctrl Pts',(-2.03182068456467,1.,-0.752642180488104));
#28515=CARTESIAN_POINT('Ctrl Pts',(-2.03814160092173,1.,-0.751562963361383));
#28516=CARTESIAN_POINT('Ctrl Pts',(-2.04446689147754,1.,-0.750444657874758));
#28517=CARTESIAN_POINT('Ctrl Pts',(-2.05079645591606,1.,-0.749287468663053));
#28518=CARTESIAN_POINT('Ctrl Pts',(-2.05713023030263,1.,-0.748091554181101));
#28519=CARTESIAN_POINT('Ctrl Pts',(-2.06220058927162,1.,-0.747103932785504));
#28520=CARTESIAN_POINT('Ctrl Pts',(-2.06600523016401,1.,-0.746345871542695));
#28521=CARTESIAN_POINT('Ctrl Pts',(-2.06854248895575,1.,-0.74583279137781));
#28522=CARTESIAN_POINT('Ctrl Pts',(-2.0698113262342,1.,-0.745574324794401));
#28523=CARTESIAN_POINT('',(-1.60662857109684,0.,-0.693717979106306));
#28524=CARTESIAN_POINT('Origin',(0.,0.,0.));
#28525=CARTESIAN_POINT('',(-1.5055822144029,1.,-0.892032620296855));
#28526=CARTESIAN_POINT('Origin',(0.,1.,0.));
#28527=CARTESIAN_POINT('',(-1.5055822144029,0.,-0.892032620296855));
#28528=CARTESIAN_POINT('Ctrl Pts',(-1.81978687191668,-1.,-1.23627494547115));
#28529=CARTESIAN_POINT('Ctrl Pts',(-1.81978687191668,1.,-1.23627494547115));
#28530=CARTESIAN_POINT('Ctrl Pts',(-1.81925017193666,-1.,-1.23509651170476));
#28531=CARTESIAN_POINT('Ctrl Pts',(-1.81925017193666,1.,-1.23509651170476));
#28532=CARTESIAN_POINT('Ctrl Pts',(-1.81817389921279,-1.,-1.2327422452705));
#28533=CARTESIAN_POINT('Ctrl Pts',(-1.81817389921279,1.,-1.2327422452705));
#28534=CARTESIAN_POINT('Ctrl Pts',(-1.8165508718364,-1.,-1.2292186489137));
#28535=CARTESIAN_POINT('Ctrl Pts',(-1.8165508718364,1.,-1.2292186489137));
#28536=CARTESIAN_POINT('Ctrl Pts',(-1.81436959210434,-1.,-1.2245361330495));
#28537=CARTESIAN_POINT('Ctrl Pts',(-1.81436959210434,1.,-1.2245361330495));
#28538=CARTESIAN_POINT('Ctrl Pts',(-1.81161420806656,-1.,-1.21870906103557));
#28539=CARTESIAN_POINT('Ctrl Pts',(-1.81161420806656,1.,-1.21870906103557));
#28540=CARTESIAN_POINT('Ctrl Pts',(-1.80882996917129,-1.,-1.21290815708314));
#28541=CARTESIAN_POINT('Ctrl Pts',(-1.80882996917129,1.,-1.21290815708314));
#28542=CARTESIAN_POINT('Ctrl Pts',(-1.80601678480707,-1.,-1.20713356605475));
#28543=CARTESIAN_POINT('Ctrl Pts',(-1.80601678480707,1.,-1.20713356605475));
#28544=CARTESIAN_POINT('Ctrl Pts',(-1.80317454838603,-1.,-1.20138548938974));
#28545=CARTESIAN_POINT('Ctrl Pts',(-1.80317454838603,1.,-1.20138548938974));
#28546=CARTESIAN_POINT('Ctrl Pts',(-1.80030314369879,-1.,-1.19566418930242));
#28547=CARTESIAN_POINT('Ctrl Pts',(-1.80030314369879,1.,-1.19566418930242));
#28548=CARTESIAN_POINT('Ctrl Pts',(-1.79740245923478,-1.,-1.18996997934445));
#28549=CARTESIAN_POINT('Ctrl Pts',(-1.79740245923478,1.,-1.18996997934445));
#28550=CARTESIAN_POINT('Ctrl Pts',(-1.79447240321515,-1.,-1.18430321697432));
#28551=CARTESIAN_POINT('Ctrl Pts',(-1.79447240321515,1.,-1.18430321697432));
#28552=CARTESIAN_POINT('Ctrl Pts',(-1.79151291552689,-1.,-1.17866429440809));
#28553=CARTESIAN_POINT('Ctrl Pts',(-1.79151291552689,1.,-1.17866429440809));
#28554=CARTESIAN_POINT('Ctrl Pts',(-1.78852398877616,-1.,-1.17305363177328));
#28555=CARTESIAN_POINT('Ctrl Pts',(-1.78852398877616,1.,-1.17305363177328));
#28556=CARTESIAN_POINT('Ctrl Pts',(-1.78550566040443,-1.,-1.16747166312303));
#28557=CARTESIAN_POINT('Ctrl Pts',(-1.78550566040443,1.,-1.16747166312303));
#28558=CARTESIAN_POINT('Ctrl Pts',(-1.78245795881009,-1.,-1.16191881298499));
#28559=CARTESIAN_POINT('Ctrl Pts',(-1.78245795881009,1.,-1.16191881298499));
#28560=CARTESIAN_POINT('Ctrl Pts',(-1.77938085564275,-1.,-1.15639547194698));
#28561=CARTESIAN_POINT('Ctrl Pts',(-1.77938085564275,1.,-1.15639547194698));
#28562=CARTESIAN_POINT('Ctrl Pts',(-1.7762742255701,-1.,-1.15090197841515));
#28563=CARTESIAN_POINT('Ctrl Pts',(-1.7762742255701,1.,-1.15090197841515));
#28564=CARTESIAN_POINT('Ctrl Pts',(-1.77313777896194,-1.,-1.1454385822692));
#28565=CARTESIAN_POINT('Ctrl Pts',(-1.77313777896194,1.,-1.1454385822692));
#28566=CARTESIAN_POINT('Ctrl Pts',(-1.76997111386769,-1.,-1.14000548336975));
#28567=CARTESIAN_POINT('Ctrl Pts',(-1.76997111386769,1.,-1.14000548336975));
#28568=CARTESIAN_POINT('Ctrl Pts',(-1.76677384551862,-1.,-1.1346029180462));
#28569=CARTESIAN_POINT('Ctrl Pts',(-1.76677384551862,1.,-1.1346029180462));
#28570=CARTESIAN_POINT('Ctrl Pts',(-1.7635457196617,-1.,-1.12923123555075));
#28571=CARTESIAN_POINT('Ctrl Pts',(-1.7635457196617,1.,-1.12923123555075));
#28572=CARTESIAN_POINT('Ctrl Pts',(-1.76028671825096,-1.,-1.12389096855086));
#28573=CARTESIAN_POINT('Ctrl Pts',(-1.76028671825096,1.,-1.12389096855086));
#28574=CARTESIAN_POINT('Ctrl Pts',(-1.75699720772105,-1.,-1.11858293216763));
#28575=CARTESIAN_POINT('Ctrl Pts',(-1.75699720772105,1.,-1.11858293216763));
#28576=CARTESIAN_POINT('Ctrl Pts',(-1.7536777209463,-1.,-1.11330807582551));
#28577=CARTESIAN_POINT('Ctrl Pts',(-1.7536777209463,1.,-1.11330807582551));
#28578=CARTESIAN_POINT('Ctrl Pts',(-1.7503286607592,-1.,-1.10806728183007));
#28579=CARTESIAN_POINT('Ctrl Pts',(-1.7503286607592,1.,-1.10806728183007));
#28580=CARTESIAN_POINT('Ctrl Pts',(-1.74695004214923,-1.,-1.10286118991143));
#28581=CARTESIAN_POINT('Ctrl Pts',(-1.74695004214923,1.,-1.10286118991143));
#28582=CARTESIAN_POINT('Ctrl Pts',(-1.74354119236208,-1.,-1.09768999241225));
#28583=CARTESIAN_POINT('Ctrl Pts',(-1.74354119236208,1.,-1.09768999241225));
#28584=CARTESIAN_POINT('Ctrl Pts',(-1.74010053962247,-1.,-1.09255329056493));
#28585=CARTESIAN_POINT('Ctrl Pts',(-1.74010053962247,1.,-1.09255329056493));
#28586=CARTESIAN_POINT('Ctrl Pts',(-1.73662628326091,-1.,-1.08745056285427));
#28587=CARTESIAN_POINT('Ctrl Pts',(-1.73662628326091,1.,-1.08745056285427));
#28588=CARTESIAN_POINT('Ctrl Pts',(-1.73311705663407,-1.,-1.08238162784749));
#28589=CARTESIAN_POINT('Ctrl Pts',(-1.73311705663407,1.,-1.08238162784749));
#28590=CARTESIAN_POINT('Ctrl Pts',(-1.72957248977424,-1.,-1.0773470373727));
#28591=CARTESIAN_POINT('Ctrl Pts',(-1.72957248977424,1.,-1.0773470373727));
#28592=CARTESIAN_POINT('Ctrl Pts',(-1.72599406198488,-1.,-1.07234866990252));
#28593=CARTESIAN_POINT('Ctrl Pts',(-1.72599406198488,1.,-1.07234866990252));
#28594=CARTESIAN_POINT('Ctrl Pts',(-1.72238500928453,-1.,-1.06738966975462));
#28595=CARTESIAN_POINT('Ctrl Pts',(-1.72238500928453,1.,-1.06738966975462));
#28596=CARTESIAN_POINT('Ctrl Pts',(-1.71874858456904,-1.,-1.06247324680647));
#28597=CARTESIAN_POINT('Ctrl Pts',(-1.71874858456904,1.,-1.06247324680647));
#28598=CARTESIAN_POINT('Ctrl Pts',(-1.7150865442702,-1.,-1.05760163192479));
#28599=CARTESIAN_POINT('Ctrl Pts',(-1.7150865442702,1.,-1.05760163192479));
#28600=CARTESIAN_POINT('Ctrl Pts',(-1.71139783543989,-1.,-1.05277517202855));
#28601=CARTESIAN_POINT('Ctrl Pts',(-1.71139783543989,1.,-1.05277517202855));
#28602=CARTESIAN_POINT('Ctrl Pts',(-1.70767646263649,-1.,-1.04799085404995));
#28603=CARTESIAN_POINT('Ctrl Pts',(-1.70767646263649,1.,-1.04799085404995));
#28604=CARTESIAN_POINT('Ctrl Pts',(-1.70391338707982,-1.,-1.04324363334554));
#28605=CARTESIAN_POINT('Ctrl Pts',(-1.70391338707982,1.,-1.04324363334554));
#28606=CARTESIAN_POINT('Ctrl Pts',(-1.70010052930962,-1.,-1.03852922490789));
#28607=CARTESIAN_POINT('Ctrl Pts',(-1.70010052930962,1.,-1.03852922490789));
#28608=CARTESIAN_POINT('Ctrl Pts',(-1.69623414782771,-1.,-1.03384646003588));
#28609=CARTESIAN_POINT('Ctrl Pts',(-1.69623414782771,1.,-1.03384646003588));
#28610=CARTESIAN_POINT('Ctrl Pts',(-1.69231840863458,-1.,-1.02919977579147));
#28611=CARTESIAN_POINT('Ctrl Pts',(-1.69231840863458,1.,-1.02919977579147));
#28612=CARTESIAN_POINT('Ctrl Pts',(-1.68836910178447,-1.,-1.02460180535255));
#28613=CARTESIAN_POINT('Ctrl Pts',(-1.68836910178447,1.,-1.02460180535255));
#28614=CARTESIAN_POINT('Ctrl Pts',(-1.68440578021706,-1.,-1.02006795074201));
#28615=CARTESIAN_POINT('Ctrl Pts',(-1.68440578021706,1.,-1.02006795074201));
#28616=CARTESIAN_POINT('Ctrl Pts',(-1.68044289894798,-1.,-1.01561026162773));
#28617=CARTESIAN_POINT('Ctrl Pts',(-1.68044289894798,1.,-1.01561026162773));
#28618=CARTESIAN_POINT('Ctrl Pts',(-1.67648246776464,-1.,-1.01123236493511));
#28619=CARTESIAN_POINT('Ctrl Pts',(-1.67648246776464,1.,-1.01123236493511));
#28620=CARTESIAN_POINT('Ctrl Pts',(-1.67250335383293,-1.,-1.00692206696414));
#28621=CARTESIAN_POINT('Ctrl Pts',(-1.67250335383293,1.,-1.00692206696414));
#28622=CARTESIAN_POINT('Ctrl Pts',(-1.66846059277303,-1.,-1.00265091003727));
#28623=CARTESIAN_POINT('Ctrl Pts',(-1.66846059277303,1.,-1.00265091003727));
#28624=CARTESIAN_POINT('Ctrl Pts',(-1.66430758030376,-1.,-0.998389654952758));
#28625=CARTESIAN_POINT('Ctrl Pts',(-1.66430758030376,1.,-0.998389654952758));
#28626=CARTESIAN_POINT('Ctrl Pts',(-1.66001553809947,-1.,-0.994121836661306));
#28627=CARTESIAN_POINT('Ctrl Pts',(-1.66001553809947,1.,-0.994121836661306));
#28628=CARTESIAN_POINT('Ctrl Pts',(-1.65559044289699,-1.,-0.989855627854165));
#28629=CARTESIAN_POINT('Ctrl Pts',(-1.65559044289699,1.,-0.989855627854165));
#28630=CARTESIAN_POINT('Ctrl Pts',(-1.65110016612638,-1.,-0.985642622920821));
#28631=CARTESIAN_POINT('Ctrl Pts',(-1.65110016612638,1.,-0.985642622920821));
#28632=CARTESIAN_POINT('Ctrl Pts',(-1.64665139190656,-1.,-0.981562530939489));
#28633=CARTESIAN_POINT('Ctrl Pts',(-1.64665139190656,1.,-0.981562530939489));
#28634=CARTESIAN_POINT('Ctrl Pts',(-1.64233990826687,-1.,-0.977689794119416));
#28635=CARTESIAN_POINT('Ctrl Pts',(-1.64233990826687,1.,-0.977689794119416));
#28636=CARTESIAN_POINT('Ctrl Pts',(-1.63820952658144,-1.,-0.974066058287418));
#28637=CARTESIAN_POINT('Ctrl Pts',(-1.63820952658144,1.,-0.974066058287418));
#28638=CARTESIAN_POINT('Ctrl Pts',(-1.63420665729798,-1.,-0.970669715997509));
#28639=CARTESIAN_POINT('Ctrl Pts',(-1.63420665729798,1.,-0.970669715997509));
#28640=CARTESIAN_POINT('Ctrl Pts',(-1.63013849959461,-1.,-0.967387853230345));
#28641=CARTESIAN_POINT('Ctrl Pts',(-1.63013849959461,1.,-0.967387853230345));
#28642=CARTESIAN_POINT('Ctrl Pts',(-1.62571930670187,-1.,-0.964046107040536));
#28643=CARTESIAN_POINT('Ctrl Pts',(-1.62571930670187,1.,-0.964046107040536));
#28644=CARTESIAN_POINT('Ctrl Pts',(-1.62061638140221,-1.,-0.960438326101729));
#28645=CARTESIAN_POINT('Ctrl Pts',(-1.62061638140221,1.,-0.960438326101729));
#28646=CARTESIAN_POINT('Ctrl Pts',(-1.61449324337085,-1.,-0.956354422920671));
#28647=CARTESIAN_POINT('Ctrl Pts',(-1.61449324337085,1.,-0.956354422920671));
#28648=CARTESIAN_POINT('Ctrl Pts',(-1.60706069896936,-1.,-0.951613284356035));
#28649=CARTESIAN_POINT('Ctrl Pts',(-1.60706069896936,1.,-0.951613284356035));
#28650=CARTESIAN_POINT('Ctrl Pts',(-1.59810042043673,-1.,-0.946078063315257));
#28651=CARTESIAN_POINT('Ctrl Pts',(-1.59810042043673,1.,-0.946078063315257));
#28652=CARTESIAN_POINT('Ctrl Pts',(-1.58744937487176,-1.,-0.939646377893399));
#28653=CARTESIAN_POINT('Ctrl Pts',(-1.58744937487176,1.,-0.939646377893399));
#28654=CARTESIAN_POINT('Ctrl Pts',(-1.57499388382243,-1.,-0.932246680108685));
#28655=CARTESIAN_POINT('Ctrl Pts',(-1.57499388382243,1.,-0.932246680108685));
#28656=CARTESIAN_POINT('Ctrl Pts',(-1.56065988578893,-1.,-0.923832188944341));
#28657=CARTESIAN_POINT('Ctrl Pts',(-1.56065988578893,1.,-0.923832188944341));
#28658=CARTESIAN_POINT('Ctrl Pts',(-1.54440491149498,-1.,-0.914375919026456));
#28659=CARTESIAN_POINT('Ctrl Pts',(-1.54440491149498,1.,-0.914375919026456));
#28660=CARTESIAN_POINT('Ctrl Pts',(-1.52984849887993,-1.,-0.905967409625651));
#28661=CARTESIAN_POINT('Ctrl Pts',(-1.52984849887993,1.,-0.905967409625651));
#28662=CARTESIAN_POINT('Ctrl Pts',(-1.51805569590094,-1.,-0.899185047483511));
#28663=CARTESIAN_POINT('Ctrl Pts',(-1.51805569590094,1.,-0.899185047483511));
#28664=CARTESIAN_POINT('Ctrl Pts',(-1.50980486806688,-1.,-0.894452006964543));
#28665=CARTESIAN_POINT('Ctrl Pts',(-1.50980486806688,1.,-0.894452006964543));
#28666=CARTESIAN_POINT('Ctrl Pts',(-1.5055822144029,-1.,-0.892032620296855));
#28667=CARTESIAN_POINT('Ctrl Pts',(-1.5055822144029,1.,-0.892032620296855));
#28668=CARTESIAN_POINT('',(-1.81978687191668,1.,-1.23627494547115));
#28669=CARTESIAN_POINT('Ctrl Pts',(-1.81978687191668,1.,-1.23627494547115));
#28670=CARTESIAN_POINT('Ctrl Pts',(-1.81925017193666,1.,-1.23509651170476));
#28671=CARTESIAN_POINT('Ctrl Pts',(-1.81817389921279,1.,-1.2327422452705));
#28672=CARTESIAN_POINT('Ctrl Pts',(-1.8165508718364,1.,-1.2292186489137));
#28673=CARTESIAN_POINT('Ctrl Pts',(-1.81436959210434,1.,-1.2245361330495));
#28674=CARTESIAN_POINT('Ctrl Pts',(-1.81161420806656,1.,-1.21870906103557));
#28675=CARTESIAN_POINT('Ctrl Pts',(-1.80882996917129,1.,-1.21290815708314));
#28676=CARTESIAN_POINT('Ctrl Pts',(-1.80601678480707,1.,-1.20713356605475));
#28677=CARTESIAN_POINT('Ctrl Pts',(-1.80317454838603,1.,-1.20138548938974));
#28678=CARTESIAN_POINT('Ctrl Pts',(-1.80030314369879,1.,-1.19566418930242));
#28679=CARTESIAN_POINT('Ctrl Pts',(-1.79740245923478,1.,-1.18996997934445));
#28680=CARTESIAN_POINT('Ctrl Pts',(-1.79447240321515,1.,-1.18430321697432));
#28681=CARTESIAN_POINT('Ctrl Pts',(-1.79151291552689,1.,-1.17866429440809));
#28682=CARTESIAN_POINT('Ctrl Pts',(-1.78852398877616,1.,-1.17305363177328));
#28683=CARTESIAN_POINT('Ctrl Pts',(-1.78550566040443,1.,-1.16747166312303));
#28684=CARTESIAN_POINT('Ctrl Pts',(-1.78245795881009,1.,-1.16191881298499));
#28685=CARTESIAN_POINT('Ctrl Pts',(-1.77938085564275,1.,-1.15639547194698));
#28686=CARTESIAN_POINT('Ctrl Pts',(-1.7762742255701,1.,-1.15090197841515));
#28687=CARTESIAN_POINT('Ctrl Pts',(-1.77313777896194,1.,-1.1454385822692));
#28688=CARTESIAN_POINT('Ctrl Pts',(-1.76997111386769,1.,-1.14000548336975));
#28689=CARTESIAN_POINT('Ctrl Pts',(-1.76677384551862,1.,-1.1346029180462));
#28690=CARTESIAN_POINT('Ctrl Pts',(-1.7635457196617,1.,-1.12923123555075));
#28691=CARTESIAN_POINT('Ctrl Pts',(-1.76028671825096,1.,-1.12389096855086));
#28692=CARTESIAN_POINT('Ctrl Pts',(-1.75699720772105,1.,-1.11858293216763));
#28693=CARTESIAN_POINT('Ctrl Pts',(-1.7536777209463,1.,-1.11330807582551));
#28694=CARTESIAN_POINT('Ctrl Pts',(-1.7503286607592,1.,-1.10806728183007));
#28695=CARTESIAN_POINT('Ctrl Pts',(-1.74695004214923,1.,-1.10286118991143));
#28696=CARTESIAN_POINT('Ctrl Pts',(-1.74354119236208,1.,-1.09768999241225));
#28697=CARTESIAN_POINT('Ctrl Pts',(-1.74010053962247,1.,-1.09255329056493));
#28698=CARTESIAN_POINT('Ctrl Pts',(-1.73662628326091,1.,-1.08745056285427));
#28699=CARTESIAN_POINT('Ctrl Pts',(-1.73311705663407,1.,-1.08238162784749));
#28700=CARTESIAN_POINT('Ctrl Pts',(-1.72957248977424,1.,-1.0773470373727));
#28701=CARTESIAN_POINT('Ctrl Pts',(-1.72599406198488,1.,-1.07234866990252));
#28702=CARTESIAN_POINT('Ctrl Pts',(-1.72238500928453,1.,-1.06738966975462));
#28703=CARTESIAN_POINT('Ctrl Pts',(-1.71874858456904,1.,-1.06247324680647));
#28704=CARTESIAN_POINT('Ctrl Pts',(-1.7150865442702,1.,-1.05760163192479));
#28705=CARTESIAN_POINT('Ctrl Pts',(-1.71139783543989,1.,-1.05277517202855));
#28706=CARTESIAN_POINT('Ctrl Pts',(-1.70767646263649,1.,-1.04799085404995));
#28707=CARTESIAN_POINT('Ctrl Pts',(-1.70391338707982,1.,-1.04324363334554));
#28708=CARTESIAN_POINT('Ctrl Pts',(-1.70010052930962,1.,-1.03852922490789));
#28709=CARTESIAN_POINT('Ctrl Pts',(-1.69623414782771,1.,-1.03384646003588));
#28710=CARTESIAN_POINT('Ctrl Pts',(-1.69231840863458,1.,-1.02919977579147));
#28711=CARTESIAN_POINT('Ctrl Pts',(-1.68836910178447,1.,-1.02460180535255));
#28712=CARTESIAN_POINT('Ctrl Pts',(-1.68440578021706,1.,-1.02006795074201));
#28713=CARTESIAN_POINT('Ctrl Pts',(-1.68044289894798,1.,-1.01561026162773));
#28714=CARTESIAN_POINT('Ctrl Pts',(-1.67648246776464,1.,-1.01123236493511));
#28715=CARTESIAN_POINT('Ctrl Pts',(-1.67250335383293,1.,-1.00692206696414));
#28716=CARTESIAN_POINT('Ctrl Pts',(-1.66846059277303,1.,-1.00265091003727));
#28717=CARTESIAN_POINT('Ctrl Pts',(-1.66430758030376,1.,-0.998389654952758));
#28718=CARTESIAN_POINT('Ctrl Pts',(-1.66001553809947,1.,-0.994121836661306));
#28719=CARTESIAN_POINT('Ctrl Pts',(-1.65559044289699,1.,-0.989855627854165));
#28720=CARTESIAN_POINT('Ctrl Pts',(-1.65110016612638,1.,-0.985642622920821));
#28721=CARTESIAN_POINT('Ctrl Pts',(-1.64665139190656,1.,-0.981562530939489));
#28722=CARTESIAN_POINT('Ctrl Pts',(-1.64233990826687,1.,-0.977689794119416));
#28723=CARTESIAN_POINT('Ctrl Pts',(-1.63820952658144,1.,-0.974066058287418));
#28724=CARTESIAN_POINT('Ctrl Pts',(-1.63420665729798,1.,-0.970669715997509));
#28725=CARTESIAN_POINT('Ctrl Pts',(-1.63013849959461,1.,-0.967387853230345));
#28726=CARTESIAN_POINT('Ctrl Pts',(-1.62571930670187,1.,-0.964046107040536));
#28727=CARTESIAN_POINT('Ctrl Pts',(-1.62061638140221,1.,-0.960438326101729));
#28728=CARTESIAN_POINT('Ctrl Pts',(-1.61449324337085,1.,-0.956354422920671));
#28729=CARTESIAN_POINT('Ctrl Pts',(-1.60706069896936,1.,-0.951613284356035));
#28730=CARTESIAN_POINT('Ctrl Pts',(-1.59810042043673,1.,-0.946078063315257));
#28731=CARTESIAN_POINT('Ctrl Pts',(-1.58744937487176,1.,-0.939646377893399));
#28732=CARTESIAN_POINT('Ctrl Pts',(-1.57499388382243,1.,-0.932246680108685));
#28733=CARTESIAN_POINT('Ctrl Pts',(-1.56065988578893,1.,-0.923832188944341));
#28734=CARTESIAN_POINT('Ctrl Pts',(-1.54440491149498,1.,-0.914375919026456));
#28735=CARTESIAN_POINT('Ctrl Pts',(-1.52984849887993,1.,-0.905967409625651));
#28736=CARTESIAN_POINT('Ctrl Pts',(-1.51805569590094,1.,-0.899185047483511));
#28737=CARTESIAN_POINT('Ctrl Pts',(-1.50980486806688,1.,-0.894452006964543));
#28738=CARTESIAN_POINT('Ctrl Pts',(-1.5055822144029,1.,-0.892032620296855));
#28739=CARTESIAN_POINT('',(-1.81978687191668,0.,-1.23627494547115));
#28740=CARTESIAN_POINT('Origin',(-1.73811241238545,0.,-1.34869019493419));
#28741=CARTESIAN_POINT('',(-1.73811241238545,1.,-1.34869019493419));
#28742=CARTESIAN_POINT('',(-1.81978687191668,1.,-1.23627494547115));
#28743=CARTESIAN_POINT('',(-1.73811241238545,0.,-1.34869019493419));
#28744=CARTESIAN_POINT('Ctrl Pts',(-1.31362392696032,-1.,-1.15624053661742));
#28745=CARTESIAN_POINT('Ctrl Pts',(-1.31362392696032,1.,-1.15624053661742));
#28746=CARTESIAN_POINT('Ctrl Pts',(-1.31722977216397,-1.,-1.15950888730809));
#28747=CARTESIAN_POINT('Ctrl Pts',(-1.31722977216397,1.,-1.15950888730809));
#28748=CARTESIAN_POINT('Ctrl Pts',(-1.32428080721772,-1.,-1.16589330093588));
#28749=CARTESIAN_POINT('Ctrl Pts',(-1.32428080721772,1.,-1.16589330093588));
#28750=CARTESIAN_POINT('Ctrl Pts',(-1.33437539347008,-1.,-1.17501305789857));
#28751=CARTESIAN_POINT('Ctrl Pts',(-1.33437539347008,1.,-1.17501305789857));
#28752=CARTESIAN_POINT('Ctrl Pts',(-1.34687054001093,-1.,-1.18625865667441));
#28753=CARTESIAN_POINT('Ctrl Pts',(-1.34687054001093,1.,-1.18625865667441));
#28754=CARTESIAN_POINT('Ctrl Pts',(-1.36088705043885,-1.,-1.1987959077932));
#28755=CARTESIAN_POINT('Ctrl Pts',(-1.36088705043885,1.,-1.1987959077932));
#28756=CARTESIAN_POINT('Ctrl Pts',(-1.37331915607905,-1.,-1.20982812925645));
#28757=CARTESIAN_POINT('Ctrl Pts',(-1.37331915607905,1.,-1.20982812925645));
#28758=CARTESIAN_POINT('Ctrl Pts',(-1.38420564527715,-1.,-1.21938737280852));
#28759=CARTESIAN_POINT('Ctrl Pts',(-1.38420564527715,1.,-1.21938737280852));
#28760=CARTESIAN_POINT('Ctrl Pts',(-1.39361389568796,-1.,-1.22752961899387));
#28761=CARTESIAN_POINT('Ctrl Pts',(-1.39361389568796,1.,-1.22752961899387));
#28762=CARTESIAN_POINT('Ctrl Pts',(-1.40164708206106,-1.,-1.23434087290423));
#28763=CARTESIAN_POINT('Ctrl Pts',(-1.40164708206106,1.,-1.23434087290423));
#28764=CARTESIAN_POINT('Ctrl Pts',(-1.40845295531283,-1.,-1.23994455029534));
#28765=CARTESIAN_POINT('Ctrl Pts',(-1.40845295531283,1.,-1.23994455029534));
#28766=CARTESIAN_POINT('Ctrl Pts',(-1.41422913175179,-1.,-1.24450600513056));
#28767=CARTESIAN_POINT('Ctrl Pts',(-1.41422913175179,1.,-1.24450600513056));
#28768=CARTESIAN_POINT('Ctrl Pts',(-1.41923722596025,-1.,-1.24824430986571));
#28769=CARTESIAN_POINT('Ctrl Pts',(-1.41923722596025,1.,-1.24824430986571));
#28770=CARTESIAN_POINT('Ctrl Pts',(-1.42378102115575,-1.,-1.2514145557001));
#28771=CARTESIAN_POINT('Ctrl Pts',(-1.42378102115575,1.,-1.2514145557001));
#28772=CARTESIAN_POINT('Ctrl Pts',(-1.42815938799387,-1.,-1.25426945222639));
#28773=CARTESIAN_POINT('Ctrl Pts',(-1.42815938799387,1.,-1.25426945222639));
#28774=CARTESIAN_POINT('Ctrl Pts',(-1.43262645609691,-1.,-1.25702687965755));
#28775=CARTESIAN_POINT('Ctrl Pts',(-1.43262645609691,1.,-1.25702687965755));
#28776=CARTESIAN_POINT('Ctrl Pts',(-1.43734919180848,-1.,-1.25983531012005));
#28777=CARTESIAN_POINT('Ctrl Pts',(-1.43734919180848,1.,-1.25983531012005));
#28778=CARTESIAN_POINT('Ctrl Pts',(-1.44236470511303,-1.,-1.26273903323859));
#28779=CARTESIAN_POINT('Ctrl Pts',(-1.44236470511303,1.,-1.26273903323859));
#28780=CARTESIAN_POINT('Ctrl Pts',(-1.44761985001662,-1.,-1.26570925118868));
#28781=CARTESIAN_POINT('Ctrl Pts',(-1.44761985001662,1.,-1.26570925118868));
#28782=CARTESIAN_POINT('Ctrl Pts',(-1.45301422764247,-1.,-1.2686778680489));
#28783=CARTESIAN_POINT('Ctrl Pts',(-1.45301422764247,1.,-1.2686778680489));
#28784=CARTESIAN_POINT('Ctrl Pts',(-1.45843906294697,-1.,-1.27156805265289));
#28785=CARTESIAN_POINT('Ctrl Pts',(-1.45843906294697,1.,-1.27156805265289));
#28786=CARTESIAN_POINT('Ctrl Pts',(-1.46382431332476,-1.,-1.27433119897822));
#28787=CARTESIAN_POINT('Ctrl Pts',(-1.46382431332476,1.,-1.27433119897822));
#28788=CARTESIAN_POINT('Ctrl Pts',(-1.46916035917133,-1.,-1.27696414831089));
#28789=CARTESIAN_POINT('Ctrl Pts',(-1.46916035917133,1.,-1.27696414831089));
#28790=CARTESIAN_POINT('Ctrl Pts',(-1.4744717526707,-1.,-1.2794891824849));
#28791=CARTESIAN_POINT('Ctrl Pts',(-1.4744717526707,1.,-1.2794891824849));
#28792=CARTESIAN_POINT('Ctrl Pts',(-1.47980070347095,-1.,-1.28194158939517));
#28793=CARTESIAN_POINT('Ctrl Pts',(-1.47980070347095,1.,-1.28194158939517));
#28794=CARTESIAN_POINT('Ctrl Pts',(-1.4851881711891,-1.,-1.28435533880201));
#28795=CARTESIAN_POINT('Ctrl Pts',(-1.4851881711891,1.,-1.28435533880201));
#28796=CARTESIAN_POINT('Ctrl Pts',(-1.4906522831278,-1.,-1.2867467611644));
#28797=CARTESIAN_POINT('Ctrl Pts',(-1.4906522831278,1.,-1.2867467611644));
#28798=CARTESIAN_POINT('Ctrl Pts',(-1.49618896881754,-1.,-1.28911506584254));
#28799=CARTESIAN_POINT('Ctrl Pts',(-1.49618896881754,1.,-1.28911506584254));
#28800=CARTESIAN_POINT('Ctrl Pts',(-1.50178230149776,-1.,-1.29145022885181));
#28801=CARTESIAN_POINT('Ctrl Pts',(-1.50178230149776,1.,-1.29145022885181));
#28802=CARTESIAN_POINT('Ctrl Pts',(-1.50741159078365,-1.,-1.29373841372842));
#28803=CARTESIAN_POINT('Ctrl Pts',(-1.50741159078365,1.,-1.29373841372842));
#28804=CARTESIAN_POINT('Ctrl Pts',(-1.51305994241402,-1.,-1.29596850710509));
#28805=CARTESIAN_POINT('Ctrl Pts',(-1.51305994241402,1.,-1.29596850710509));
#28806=CARTESIAN_POINT('Ctrl Pts',(-1.51872184912724,-1.,-1.29813791800747));
#28807=CARTESIAN_POINT('Ctrl Pts',(-1.51872184912724,1.,-1.29813791800747));
#28808=CARTESIAN_POINT('Ctrl Pts',(-1.52439957861062,-1.,-1.30024984366328));
#28809=CARTESIAN_POINT('Ctrl Pts',(-1.52439957861062,1.,-1.30024984366328));
#28810=CARTESIAN_POINT('Ctrl Pts',(-1.53009970283891,-1.,-1.30231064395568));
#28811=CARTESIAN_POINT('Ctrl Pts',(-1.53009970283891,1.,-1.30231064395568));
#28812=CARTESIAN_POINT('Ctrl Pts',(-1.53582981268977,-1.,-1.30432735639489));
#28813=CARTESIAN_POINT('Ctrl Pts',(-1.53582981268977,1.,-1.30432735639489));
#28814=CARTESIAN_POINT('Ctrl Pts',(-1.54159462645432,-1.,-1.30630475189556));
#28815=CARTESIAN_POINT('Ctrl Pts',(-1.54159462645432,1.,-1.30630475189556));
#28816=CARTESIAN_POINT('Ctrl Pts',(-1.54739413957185,-1.,-1.30824393907473));
#28817=CARTESIAN_POINT('Ctrl Pts',(-1.54739413957185,1.,-1.30824393907473));
#28818=CARTESIAN_POINT('Ctrl Pts',(-1.55322568759481,-1.,-1.31014393684222));
#28819=CARTESIAN_POINT('Ctrl Pts',(-1.55322568759481,1.,-1.31014393684222));
#28820=CARTESIAN_POINT('Ctrl Pts',(-1.55908521254821,-1.,-1.31200264341696));
#28821=CARTESIAN_POINT('Ctrl Pts',(-1.55908521254821,1.,-1.31200264341696));
#28822=CARTESIAN_POINT('Ctrl Pts',(-1.56496872402353,-1.,-1.31381795281002));
#28823=CARTESIAN_POINT('Ctrl Pts',(-1.56496872402353,1.,-1.31381795281002));
#28824=CARTESIAN_POINT('Ctrl Pts',(-1.57087397835723,-1.,-1.31558903860016));
#28825=CARTESIAN_POINT('Ctrl Pts',(-1.57087397835723,1.,-1.31558903860016));
#28826=CARTESIAN_POINT('Ctrl Pts',(-1.5768005650559,-1.,-1.31731642317187));
#28827=CARTESIAN_POINT('Ctrl Pts',(-1.5768005650559,1.,-1.31731642317187));
#28828=CARTESIAN_POINT('Ctrl Pts',(-1.58274907898834,-1.,-1.31900135021432));
#28829=CARTESIAN_POINT('Ctrl Pts',(-1.58274907898834,1.,-1.31900135021432));
#28830=CARTESIAN_POINT('Ctrl Pts',(-1.58872057258245,-1.,-1.32064537110892));
#28831=CARTESIAN_POINT('Ctrl Pts',(-1.58872057258245,1.,-1.32064537110892));
#28832=CARTESIAN_POINT('Ctrl Pts',(-1.59471591079403,-1.,-1.32224985747682));
#28833=CARTESIAN_POINT('Ctrl Pts',(-1.59471591079403,1.,-1.32224985747682));
#28834=CARTESIAN_POINT('Ctrl Pts',(-1.60073511858687,-1.,-1.32381550858256));
#28835=CARTESIAN_POINT('Ctrl Pts',(-1.60073511858687,1.,-1.32381550858256));
#28836=CARTESIAN_POINT('Ctrl Pts',(-1.60677758290954,-1.,-1.32534250785782));
#28837=CARTESIAN_POINT('Ctrl Pts',(-1.60677758290954,1.,-1.32534250785782));
#28838=CARTESIAN_POINT('Ctrl Pts',(-1.6128423401575,-1.,-1.32683074483356));
#28839=CARTESIAN_POINT('Ctrl Pts',(-1.6128423401575,1.,-1.32683074483356));
#28840=CARTESIAN_POINT('Ctrl Pts',(-1.61892832270724,-1.,-1.32828000610449));
#28841=CARTESIAN_POINT('Ctrl Pts',(-1.61892832270724,1.,-1.32828000610449));
#28842=CARTESIAN_POINT('Ctrl Pts',(-1.62503464209797,-1.,-1.3296901950568));
#28843=CARTESIAN_POINT('Ctrl Pts',(-1.62503464209797,1.,-1.3296901950568));
#28844=CARTESIAN_POINT('Ctrl Pts',(-1.63116079730923,-1.,-1.33106149345645));
#28845=CARTESIAN_POINT('Ctrl Pts',(-1.63116079730923,1.,-1.33106149345645));
#28846=CARTESIAN_POINT('Ctrl Pts',(-1.63730653475089,-1.,-1.33239425103724));
#28847=CARTESIAN_POINT('Ctrl Pts',(-1.63730653475089,1.,-1.33239425103724));
#28848=CARTESIAN_POINT('Ctrl Pts',(-1.6434717485603,-1.,-1.33368890676572));
#28849=CARTESIAN_POINT('Ctrl Pts',(-1.6434717485603,1.,-1.33368890676572));
#28850=CARTESIAN_POINT('Ctrl Pts',(-1.6496563728683,-1.,-1.33494590467993));
#28851=CARTESIAN_POINT('Ctrl Pts',(-1.6496563728683,1.,-1.33494590467993));
#28852=CARTESIAN_POINT('Ctrl Pts',(-1.65586025952593,-1.,-1.33616559745172));
#28853=CARTESIAN_POINT('Ctrl Pts',(-1.65586025952593,1.,-1.33616559745172));
#28854=CARTESIAN_POINT('Ctrl Pts',(-1.66208312541983,-1.,-1.33734820885262));
#28855=CARTESIAN_POINT('Ctrl Pts',(-1.66208312541983,1.,-1.33734820885262));
#28856=CARTESIAN_POINT('Ctrl Pts',(-1.66832460783989,-1.,-1.33849388654388));
#28857=CARTESIAN_POINT('Ctrl Pts',(-1.66832460783989,1.,-1.33849388654388));
#28858=CARTESIAN_POINT('Ctrl Pts',(-1.67458429426086,-1.,-1.3396027347034));
#28859=CARTESIAN_POINT('Ctrl Pts',(-1.67458429426086,1.,-1.3396027347034));
#28860=CARTESIAN_POINT('Ctrl Pts',(-1.68086176030362,-1.,-1.34067485185203));
#28861=CARTESIAN_POINT('Ctrl Pts',(-1.68086176030362,1.,-1.34067485185203));
#28862=CARTESIAN_POINT('Ctrl Pts',(-1.68715660868764,-1.,-1.341710374848));
#28863=CARTESIAN_POINT('Ctrl Pts',(-1.68715660868764,1.,-1.341710374848));
#28864=CARTESIAN_POINT('Ctrl Pts',(-1.6934684849687,-1.,-1.34270948206319));
#28865=CARTESIAN_POINT('Ctrl Pts',(-1.6934684849687,1.,-1.34270948206319));
#28866=CARTESIAN_POINT('Ctrl Pts',(-1.69979707754427,-1.,-1.34367237124483));
#28867=CARTESIAN_POINT('Ctrl Pts',(-1.69979707754427,1.,-1.34367237124483));
#28868=CARTESIAN_POINT('Ctrl Pts',(-1.70614212266738,-1.,-1.34459924533831));
#28869=CARTESIAN_POINT('Ctrl Pts',(-1.70614212266738,1.,-1.34459924533831));
#28870=CARTESIAN_POINT('Ctrl Pts',(-1.71250340686822,-1.,-1.34549029589416));
#28871=CARTESIAN_POINT('Ctrl Pts',(-1.71250340686822,1.,-1.34549029589416));
#28872=CARTESIAN_POINT('Ctrl Pts',(-1.7188807715049,-1.,-1.34634568653227));
#28873=CARTESIAN_POINT('Ctrl Pts',(-1.7188807715049,1.,-1.34634568653227));
#28874=CARTESIAN_POINT('Ctrl Pts',(-1.72527410680674,-1.,-1.34716554819527));
#28875=CARTESIAN_POINT('Ctrl Pts',(-1.72527410680674,1.,-1.34716554819527));
#28876=CARTESIAN_POINT('Ctrl Pts',(-1.7304014965394,-1.,-1.34779309152035));
#28877=CARTESIAN_POINT('Ctrl Pts',(-1.7304014965394,1.,-1.34779309152035));
#28878=CARTESIAN_POINT('Ctrl Pts',(-1.73425417885907,-1.,-1.34824783112887));
#28879=CARTESIAN_POINT('Ctrl Pts',(-1.73425417885907,1.,-1.34824783112887));
#28880=CARTESIAN_POINT('Ctrl Pts',(-1.73682580585691,-1.,-1.34854391898045));
#28881=CARTESIAN_POINT('Ctrl Pts',(-1.73682580585691,1.,-1.34854391898045));
#28882=CARTESIAN_POINT('Ctrl Pts',(-1.73811241238545,-1.,-1.34869019493419));
#28883=CARTESIAN_POINT('Ctrl Pts',(-1.73811241238545,1.,-1.34869019493419));
#28884=CARTESIAN_POINT('',(-1.31362392696032,1.,-1.15624053661742));
#28885=CARTESIAN_POINT('Ctrl Pts',(-1.31362392696032,1.,-1.15624053661742));
#28886=CARTESIAN_POINT('Ctrl Pts',(-1.31722977216397,1.,-1.15950888730809));
#28887=CARTESIAN_POINT('Ctrl Pts',(-1.32428080721772,1.,-1.16589330093588));
#28888=CARTESIAN_POINT('Ctrl Pts',(-1.33437539347008,1.,-1.17501305789857));
#28889=CARTESIAN_POINT('Ctrl Pts',(-1.34687054001093,1.,-1.18625865667441));
#28890=CARTESIAN_POINT('Ctrl Pts',(-1.36088705043885,1.,-1.1987959077932));
#28891=CARTESIAN_POINT('Ctrl Pts',(-1.37331915607905,1.,-1.20982812925645));
#28892=CARTESIAN_POINT('Ctrl Pts',(-1.38420564527715,1.,-1.21938737280852));
#28893=CARTESIAN_POINT('Ctrl Pts',(-1.39361389568796,1.,-1.22752961899387));
#28894=CARTESIAN_POINT('Ctrl Pts',(-1.40164708206106,1.,-1.23434087290423));
#28895=CARTESIAN_POINT('Ctrl Pts',(-1.40845295531283,1.,-1.23994455029534));
#28896=CARTESIAN_POINT('Ctrl Pts',(-1.41422913175179,1.,-1.24450600513056));
#28897=CARTESIAN_POINT('Ctrl Pts',(-1.41923722596025,1.,-1.24824430986571));
#28898=CARTESIAN_POINT('Ctrl Pts',(-1.42378102115575,1.,-1.2514145557001));
#28899=CARTESIAN_POINT('Ctrl Pts',(-1.42815938799387,1.,-1.25426945222639));
#28900=CARTESIAN_POINT('Ctrl Pts',(-1.43262645609691,1.,-1.25702687965755));
#28901=CARTESIAN_POINT('Ctrl Pts',(-1.43734919180848,1.,-1.25983531012005));
#28902=CARTESIAN_POINT('Ctrl Pts',(-1.44236470511303,1.,-1.26273903323859));
#28903=CARTESIAN_POINT('Ctrl Pts',(-1.44761985001662,1.,-1.26570925118868));
#28904=CARTESIAN_POINT('Ctrl Pts',(-1.45301422764247,1.,-1.2686778680489));
#28905=CARTESIAN_POINT('Ctrl Pts',(-1.45843906294697,1.,-1.27156805265289));
#28906=CARTESIAN_POINT('Ctrl Pts',(-1.46382431332476,1.,-1.27433119897822));
#28907=CARTESIAN_POINT('Ctrl Pts',(-1.46916035917133,1.,-1.27696414831089));
#28908=CARTESIAN_POINT('Ctrl Pts',(-1.4744717526707,1.,-1.2794891824849));
#28909=CARTESIAN_POINT('Ctrl Pts',(-1.47980070347095,1.,-1.28194158939517));
#28910=CARTESIAN_POINT('Ctrl Pts',(-1.4851881711891,1.,-1.28435533880201));
#28911=CARTESIAN_POINT('Ctrl Pts',(-1.4906522831278,1.,-1.2867467611644));
#28912=CARTESIAN_POINT('Ctrl Pts',(-1.49618896881754,1.,-1.28911506584254));
#28913=CARTESIAN_POINT('Ctrl Pts',(-1.50178230149776,1.,-1.29145022885181));
#28914=CARTESIAN_POINT('Ctrl Pts',(-1.50741159078365,1.,-1.29373841372842));
#28915=CARTESIAN_POINT('Ctrl Pts',(-1.51305994241402,1.,-1.29596850710509));
#28916=CARTESIAN_POINT('Ctrl Pts',(-1.51872184912724,1.,-1.29813791800747));
#28917=CARTESIAN_POINT('Ctrl Pts',(-1.52439957861062,1.,-1.30024984366328));
#28918=CARTESIAN_POINT('Ctrl Pts',(-1.53009970283891,1.,-1.30231064395568));
#28919=CARTESIAN_POINT('Ctrl Pts',(-1.53582981268977,1.,-1.30432735639489));
#28920=CARTESIAN_POINT('Ctrl Pts',(-1.54159462645432,1.,-1.30630475189556));
#28921=CARTESIAN_POINT('Ctrl Pts',(-1.54739413957185,1.,-1.30824393907473));
#28922=CARTESIAN_POINT('Ctrl Pts',(-1.55322568759481,1.,-1.31014393684222));
#28923=CARTESIAN_POINT('Ctrl Pts',(-1.55908521254821,1.,-1.31200264341696));
#28924=CARTESIAN_POINT('Ctrl Pts',(-1.56496872402353,1.,-1.31381795281002));
#28925=CARTESIAN_POINT('Ctrl Pts',(-1.57087397835723,1.,-1.31558903860016));
#28926=CARTESIAN_POINT('Ctrl Pts',(-1.5768005650559,1.,-1.31731642317187));
#28927=CARTESIAN_POINT('Ctrl Pts',(-1.58274907898834,1.,-1.31900135021432));
#28928=CARTESIAN_POINT('Ctrl Pts',(-1.58872057258245,1.,-1.32064537110892));
#28929=CARTESIAN_POINT('Ctrl Pts',(-1.59471591079403,1.,-1.32224985747682));
#28930=CARTESIAN_POINT('Ctrl Pts',(-1.60073511858687,1.,-1.32381550858256));
#28931=CARTESIAN_POINT('Ctrl Pts',(-1.60677758290954,1.,-1.32534250785782));
#28932=CARTESIAN_POINT('Ctrl Pts',(-1.6128423401575,1.,-1.32683074483356));
#28933=CARTESIAN_POINT('Ctrl Pts',(-1.61892832270724,1.,-1.32828000610449));
#28934=CARTESIAN_POINT('Ctrl Pts',(-1.62503464209797,1.,-1.3296901950568));
#28935=CARTESIAN_POINT('Ctrl Pts',(-1.63116079730923,1.,-1.33106149345645));
#28936=CARTESIAN_POINT('Ctrl Pts',(-1.63730653475089,1.,-1.33239425103724));
#28937=CARTESIAN_POINT('Ctrl Pts',(-1.6434717485603,1.,-1.33368890676572));
#28938=CARTESIAN_POINT('Ctrl Pts',(-1.6496563728683,1.,-1.33494590467993));
#28939=CARTESIAN_POINT('Ctrl Pts',(-1.65586025952593,1.,-1.33616559745172));
#28940=CARTESIAN_POINT('Ctrl Pts',(-1.66208312541983,1.,-1.33734820885262));
#28941=CARTESIAN_POINT('Ctrl Pts',(-1.66832460783989,1.,-1.33849388654388));
#28942=CARTESIAN_POINT('Ctrl Pts',(-1.67458429426086,1.,-1.3396027347034));
#28943=CARTESIAN_POINT('Ctrl Pts',(-1.68086176030362,1.,-1.34067485185203));
#28944=CARTESIAN_POINT('Ctrl Pts',(-1.68715660868764,1.,-1.341710374848));
#28945=CARTESIAN_POINT('Ctrl Pts',(-1.6934684849687,1.,-1.34270948206319));
#28946=CARTESIAN_POINT('Ctrl Pts',(-1.69979707754427,1.,-1.34367237124483));
#28947=CARTESIAN_POINT('Ctrl Pts',(-1.70614212266738,1.,-1.34459924533831));
#28948=CARTESIAN_POINT('Ctrl Pts',(-1.71250340686822,1.,-1.34549029589416));
#28949=CARTESIAN_POINT('Ctrl Pts',(-1.7188807715049,1.,-1.34634568653227));
#28950=CARTESIAN_POINT('Ctrl Pts',(-1.72527410680674,1.,-1.34716554819527));
#28951=CARTESIAN_POINT('Ctrl Pts',(-1.7304014965394,1.,-1.34779309152035));
#28952=CARTESIAN_POINT('Ctrl Pts',(-1.73425417885907,1.,-1.34824783112887));
#28953=CARTESIAN_POINT('Ctrl Pts',(-1.73682580585691,1.,-1.34854391898045));
#28954=CARTESIAN_POINT('Ctrl Pts',(-1.73811241238545,1.,-1.34869019493419));
#28955=CARTESIAN_POINT('',(-1.31362392696032,0.,-1.15624053661742));
#28956=CARTESIAN_POINT('Origin',(0.,0.,0.));
#28957=CARTESIAN_POINT('',(-1.15624053661742,1.,-1.31362392696033));
#28958=CARTESIAN_POINT('Origin',(0.,1.,0.));
#28959=CARTESIAN_POINT('',(-1.15624053661742,0.,-1.31362392696033));
#28960=CARTESIAN_POINT('Ctrl Pts',(-1.34869019493419,-1.,-1.73811241238545));
#28961=CARTESIAN_POINT('Ctrl Pts',(-1.34869019493419,1.,-1.73811241238545));
#28962=CARTESIAN_POINT('Ctrl Pts',(-1.34854391898145,-1.,-1.73682580585819));
#28963=CARTESIAN_POINT('Ctrl Pts',(-1.34854391898145,1.,-1.73682580585819));
#28964=CARTESIAN_POINT('Ctrl Pts',(-1.34824783113158,-1.,-1.73425417886255));
#28965=CARTESIAN_POINT('Ctrl Pts',(-1.34824783113158,1.,-1.73425417886255));
#28966=CARTESIAN_POINT('Ctrl Pts',(-1.3477930915247,-1.,-1.73040149654497));
#28967=CARTESIAN_POINT('Ctrl Pts',(-1.3477930915247,1.,-1.73040149654497));
#28968=CARTESIAN_POINT('Ctrl Pts',(-1.34716554820013,-1.,-1.72527410681298));
#28969=CARTESIAN_POINT('Ctrl Pts',(-1.34716554820013,1.,-1.72527410681298));
#28970=CARTESIAN_POINT('Ctrl Pts',(-1.34634568653586,-1.,-1.7188807715095));
#28971=CARTESIAN_POINT('Ctrl Pts',(-1.34634568653586,1.,-1.7188807715095));
#28972=CARTESIAN_POINT('Ctrl Pts',(-1.34549029589563,-1.,-1.71250340687011));
#28973=CARTESIAN_POINT('Ctrl Pts',(-1.34549029589563,1.,-1.71250340687011));
#28974=CARTESIAN_POINT('Ctrl Pts',(-1.34459924533783,-1.,-1.70614212266676));
#28975=CARTESIAN_POINT('Ctrl Pts',(-1.34459924533783,1.,-1.70614212266676));
#28976=CARTESIAN_POINT('Ctrl Pts',(-1.34367237124322,-1.,-1.69979707754221));
#28977=CARTESIAN_POINT('Ctrl Pts',(-1.34367237124322,1.,-1.69979707754221));
#28978=CARTESIAN_POINT('Ctrl Pts',(-1.34270948206139,-1.,-1.6934684849664));
#28979=CARTESIAN_POINT('Ctrl Pts',(-1.34270948206139,1.,-1.6934684849664));
#28980=CARTESIAN_POINT('Ctrl Pts',(-1.34171037484673,-1.,-1.68715660868602));
#28981=CARTESIAN_POINT('Ctrl Pts',(-1.34171037484673,1.,-1.68715660868602));
#28982=CARTESIAN_POINT('Ctrl Pts',(-1.3406748518516,-1.,-1.68086176030308));
#28983=CARTESIAN_POINT('Ctrl Pts',(-1.3406748518516,1.,-1.68086176030308));
#28984=CARTESIAN_POINT('Ctrl Pts',(-1.33960273470372,-1.,-1.67458429426126));
#28985=CARTESIAN_POINT('Ctrl Pts',(-1.33960273470372,1.,-1.67458429426126));
#28986=CARTESIAN_POINT('Ctrl Pts',(-1.33849388654458,-1.,-1.66832460784078));
#28987=CARTESIAN_POINT('Ctrl Pts',(-1.33849388654458,1.,-1.66832460784078));
#28988=CARTESIAN_POINT('Ctrl Pts',(-1.33734820885331,-1.,-1.66208312542073));
#28989=CARTESIAN_POINT('Ctrl Pts',(-1.33734820885331,1.,-1.66208312542073));
#28990=CARTESIAN_POINT('Ctrl Pts',(-1.33616559745217,-1.,-1.65586025952651));
#28991=CARTESIAN_POINT('Ctrl Pts',(-1.33616559745217,1.,-1.65586025952651));
#28992=CARTESIAN_POINT('Ctrl Pts',(-1.33494590468003,-1.,-1.64965637286843));
#28993=CARTESIAN_POINT('Ctrl Pts',(-1.33494590468003,1.,-1.64965637286843));
#28994=CARTESIAN_POINT('Ctrl Pts',(-1.33368890676554,-1.,-1.64347174856007));
#28995=CARTESIAN_POINT('Ctrl Pts',(-1.33368890676554,1.,-1.64347174856007));
#28996=CARTESIAN_POINT('Ctrl Pts',(-1.33239425103694,-1.,-1.6373065347505));
#28997=CARTESIAN_POINT('Ctrl Pts',(-1.33239425103694,1.,-1.6373065347505));
#28998=CARTESIAN_POINT('Ctrl Pts',(-1.33106149345618,-1.,-1.63116079730887));
#28999=CARTESIAN_POINT('Ctrl Pts',(-1.33106149345618,1.,-1.63116079730887));
#29000=CARTESIAN_POINT('Ctrl Pts',(-1.32969019505665,-1.,-1.62503464209777));
#29001=CARTESIAN_POINT('Ctrl Pts',(-1.32969019505665,1.,-1.62503464209777));
#29002=CARTESIAN_POINT('Ctrl Pts',(-1.32828000610448,-1.,-1.61892832270723));
#29003=CARTESIAN_POINT('Ctrl Pts',(-1.32828000610448,1.,-1.61892832270723));
#29004=CARTESIAN_POINT('Ctrl Pts',(-1.32683074483365,-1.,-1.61284234015762));
#29005=CARTESIAN_POINT('Ctrl Pts',(-1.32683074483365,1.,-1.61284234015762));
#29006=CARTESIAN_POINT('Ctrl Pts',(-1.32534250785794,-1.,-1.6067775829097));
#29007=CARTESIAN_POINT('Ctrl Pts',(-1.32534250785794,1.,-1.6067775829097));
#29008=CARTESIAN_POINT('Ctrl Pts',(-1.32381550858266,-1.,-1.600735118587));
#29009=CARTESIAN_POINT('Ctrl Pts',(-1.32381550858266,1.,-1.600735118587));
#29010=CARTESIAN_POINT('Ctrl Pts',(-1.32224985747686,-1.,-1.59471591079408));
#29011=CARTESIAN_POINT('Ctrl Pts',(-1.32224985747686,1.,-1.59471591079408));
#29012=CARTESIAN_POINT('Ctrl Pts',(-1.32064537110891,-1.,-1.58872057258244));
#29013=CARTESIAN_POINT('Ctrl Pts',(-1.32064537110891,1.,-1.58872057258244));
#29014=CARTESIAN_POINT('Ctrl Pts',(-1.31900135021428,-1.,-1.58274907898829));
#29015=CARTESIAN_POINT('Ctrl Pts',(-1.31900135021428,1.,-1.58274907898829));
#29016=CARTESIAN_POINT('Ctrl Pts',(-1.31731642317183,-1.,-1.57680056505585));
#29017=CARTESIAN_POINT('Ctrl Pts',(-1.31731642317183,1.,-1.57680056505585));
#29018=CARTESIAN_POINT('Ctrl Pts',(-1.31558903860015,-1.,-1.57087397835721));
#29019=CARTESIAN_POINT('Ctrl Pts',(-1.31558903860015,1.,-1.57087397835721));
#29020=CARTESIAN_POINT('Ctrl Pts',(-1.31381795281002,-1.,-1.56496872402352));
#29021=CARTESIAN_POINT('Ctrl Pts',(-1.31381795281002,1.,-1.56496872402352));
#29022=CARTESIAN_POINT('Ctrl Pts',(-1.31200264341696,-1.,-1.55908521254822));
#29023=CARTESIAN_POINT('Ctrl Pts',(-1.31200264341696,1.,-1.55908521254822));
#29024=CARTESIAN_POINT('Ctrl Pts',(-1.31014393684221,-1.,-1.55322568759481));
#29025=CARTESIAN_POINT('Ctrl Pts',(-1.31014393684221,1.,-1.55322568759481));
#29026=CARTESIAN_POINT('Ctrl Pts',(-1.30824393907471,-1.,-1.54739413957183));
#29027=CARTESIAN_POINT('Ctrl Pts',(-1.30824393907471,1.,-1.54739413957183));
#29028=CARTESIAN_POINT('Ctrl Pts',(-1.30630475189553,-1.,-1.54159462645428));
#29029=CARTESIAN_POINT('Ctrl Pts',(-1.30630475189553,1.,-1.54159462645428));
#29030=CARTESIAN_POINT('Ctrl Pts',(-1.30432735639487,-1.,-1.53582981268976));
#29031=CARTESIAN_POINT('Ctrl Pts',(-1.30432735639487,1.,-1.53582981268976));
#29032=CARTESIAN_POINT('Ctrl Pts',(-1.3023106439557,-1.,-1.53009970283893));
#29033=CARTESIAN_POINT('Ctrl Pts',(-1.3023106439557,1.,-1.53009970283893));
#29034=CARTESIAN_POINT('Ctrl Pts',(-1.30024984366334,-1.,-1.5243995786107));
#29035=CARTESIAN_POINT('Ctrl Pts',(-1.30024984366334,1.,-1.5243995786107));
#29036=CARTESIAN_POINT('Ctrl Pts',(-1.29813791800757,-1.,-1.51872184912735));
#29037=CARTESIAN_POINT('Ctrl Pts',(-1.29813791800757,1.,-1.51872184912735));
#29038=CARTESIAN_POINT('Ctrl Pts',(-1.29596850710518,-1.,-1.51305994241412));
#29039=CARTESIAN_POINT('Ctrl Pts',(-1.29596850710518,1.,-1.51305994241412));
#29040=CARTESIAN_POINT('Ctrl Pts',(-1.29373841372843,-1.,-1.50741159078367));
#29041=CARTESIAN_POINT('Ctrl Pts',(-1.29373841372843,1.,-1.50741159078367));
#29042=CARTESIAN_POINT('Ctrl Pts',(-1.29145022885171,-1.,-1.50178230149764));
#29043=CARTESIAN_POINT('Ctrl Pts',(-1.29145022885171,1.,-1.50178230149764));
#29044=CARTESIAN_POINT('Ctrl Pts',(-1.28911506584232,-1.,-1.49618896881729));
#29045=CARTESIAN_POINT('Ctrl Pts',(-1.28911506584232,1.,-1.49618896881729));
#29046=CARTESIAN_POINT('Ctrl Pts',(-1.28674676116415,-1.,-1.4906522831275));
#29047=CARTESIAN_POINT('Ctrl Pts',(-1.28674676116415,1.,-1.4906522831275));
#29048=CARTESIAN_POINT('Ctrl Pts',(-1.28435533880184,-1.,-1.48518817118891));
#29049=CARTESIAN_POINT('Ctrl Pts',(-1.28435533880184,1.,-1.48518817118891));
#29050=CARTESIAN_POINT('Ctrl Pts',(-1.28194158939522,-1.,-1.47980070347102));
#29051=CARTESIAN_POINT('Ctrl Pts',(-1.28194158939522,1.,-1.47980070347102));
#29052=CARTESIAN_POINT('Ctrl Pts',(-1.27948918248524,-1.,-1.4744717526711));
#29053=CARTESIAN_POINT('Ctrl Pts',(-1.27948918248524,1.,-1.4744717526711));
#29054=CARTESIAN_POINT('Ctrl Pts',(-1.27696414831144,-1.,-1.46916035917197));
#29055=CARTESIAN_POINT('Ctrl Pts',(-1.27696414831144,1.,-1.46916035917197));
#29056=CARTESIAN_POINT('Ctrl Pts',(-1.27433119897877,-1.,-1.4638243133254));
#29057=CARTESIAN_POINT('Ctrl Pts',(-1.27433119897877,1.,-1.4638243133254));
#29058=CARTESIAN_POINT('Ctrl Pts',(-1.27156805265312,-1.,-1.45843906294725));
#29059=CARTESIAN_POINT('Ctrl Pts',(-1.27156805265312,1.,-1.45843906294725));
#29060=CARTESIAN_POINT('Ctrl Pts',(-1.26867786804854,-1.,-1.45301422764205));
#29061=CARTESIAN_POINT('Ctrl Pts',(-1.26867786804854,1.,-1.45301422764205));
#29062=CARTESIAN_POINT('Ctrl Pts',(-1.26570925118767,-1.,-1.44761985001544));
#29063=CARTESIAN_POINT('Ctrl Pts',(-1.26570925118767,1.,-1.44761985001544));
#29064=CARTESIAN_POINT('Ctrl Pts',(-1.26273903323723,-1.,-1.44236470511145));
#29065=CARTESIAN_POINT('Ctrl Pts',(-1.26273903323723,1.,-1.44236470511145));
#29066=CARTESIAN_POINT('Ctrl Pts',(-1.25983531011894,-1.,-1.43734919180719));
#29067=CARTESIAN_POINT('Ctrl Pts',(-1.25983531011894,1.,-1.43734919180719));
#29068=CARTESIAN_POINT('Ctrl Pts',(-1.25702687965744,-1.,-1.43262645609679));
#29069=CARTESIAN_POINT('Ctrl Pts',(-1.25702687965744,1.,-1.43262645609679));
#29070=CARTESIAN_POINT('Ctrl Pts',(-1.25426945222783,-1.,-1.42815938799555));
#29071=CARTESIAN_POINT('Ctrl Pts',(-1.25426945222783,1.,-1.42815938799555));
#29072=CARTESIAN_POINT('Ctrl Pts',(-1.25141455570299,-1.,-1.42378102115911));
#29073=CARTESIAN_POINT('Ctrl Pts',(-1.25141455570299,1.,-1.42378102115911));
#29074=CARTESIAN_POINT('Ctrl Pts',(-1.24824430986911,-1.,-1.41923722596421));
#29075=CARTESIAN_POINT('Ctrl Pts',(-1.24824430986911,1.,-1.41923722596421));
#29076=CARTESIAN_POINT('Ctrl Pts',(-1.24450600513278,-1.,-1.41422913175437));
#29077=CARTESIAN_POINT('Ctrl Pts',(-1.24450600513278,1.,-1.41422913175437));
#29078=CARTESIAN_POINT('Ctrl Pts',(-1.23994455029421,-1.,-1.40845295531151));
#29079=CARTESIAN_POINT('Ctrl Pts',(-1.23994455029421,1.,-1.40845295531151));
#29080=CARTESIAN_POINT('Ctrl Pts',(-1.23434087289768,-1.,-1.40164708205345));
#29081=CARTESIAN_POINT('Ctrl Pts',(-1.23434087289768,1.,-1.40164708205345));
#29082=CARTESIAN_POINT('Ctrl Pts',(-1.22752961898063,-1.,-1.39361389567257));
#29083=CARTESIAN_POINT('Ctrl Pts',(-1.22752961898063,1.,-1.39361389567257));
#29084=CARTESIAN_POINT('Ctrl Pts',(-1.21938737278853,-1.,-1.38420564525391));
#29085=CARTESIAN_POINT('Ctrl Pts',(-1.21938737278853,1.,-1.38420564525391));
#29086=CARTESIAN_POINT('Ctrl Pts',(-1.20982812923113,-1.,-1.37331915604962));
#29087=CARTESIAN_POINT('Ctrl Pts',(-1.20982812923113,1.,-1.37331915604962));
#29088=CARTESIAN_POINT('Ctrl Pts',(-1.1987959077656,-1.,-1.36088705040677));
#29089=CARTESIAN_POINT('Ctrl Pts',(-1.1987959077656,1.,-1.36088705040677));
#29090=CARTESIAN_POINT('Ctrl Pts',(-1.18625865664915,-1.,-1.34687053998157));
#29091=CARTESIAN_POINT('Ctrl Pts',(-1.18625865664915,1.,-1.34687053998157));
#29092=CARTESIAN_POINT('Ctrl Pts',(-1.17501305787994,-1.,-1.33437539344842));
#29093=CARTESIAN_POINT('Ctrl Pts',(-1.17501305787994,1.,-1.33437539344842));
#29094=CARTESIAN_POINT('Ctrl Pts',(-1.16589330092532,-1.,-1.32428080720544));
#29095=CARTESIAN_POINT('Ctrl Pts',(-1.16589330092532,1.,-1.32428080720544));
#29096=CARTESIAN_POINT('Ctrl Pts',(-1.15950888730433,-1.,-1.3172297721596));
#29097=CARTESIAN_POINT('Ctrl Pts',(-1.15950888730433,1.,-1.3172297721596));
#29098=CARTESIAN_POINT('Ctrl Pts',(-1.15624053661742,-1.,-1.31362392696033));
#29099=CARTESIAN_POINT('Ctrl Pts',(-1.15624053661742,1.,-1.31362392696033));
#29100=CARTESIAN_POINT('',(-1.34869019493419,1.,-1.73811241238545));
#29101=CARTESIAN_POINT('Ctrl Pts',(-1.34869019493419,1.,-1.73811241238545));
#29102=CARTESIAN_POINT('Ctrl Pts',(-1.34854391898145,1.,-1.73682580585819));
#29103=CARTESIAN_POINT('Ctrl Pts',(-1.34824783113158,1.,-1.73425417886255));
#29104=CARTESIAN_POINT('Ctrl Pts',(-1.3477930915247,1.,-1.73040149654497));
#29105=CARTESIAN_POINT('Ctrl Pts',(-1.34716554820013,1.,-1.72527410681298));
#29106=CARTESIAN_POINT('Ctrl Pts',(-1.34634568653586,1.,-1.7188807715095));
#29107=CARTESIAN_POINT('Ctrl Pts',(-1.34549029589563,1.,-1.71250340687011));
#29108=CARTESIAN_POINT('Ctrl Pts',(-1.34459924533783,1.,-1.70614212266676));
#29109=CARTESIAN_POINT('Ctrl Pts',(-1.34367237124322,1.,-1.69979707754221));
#29110=CARTESIAN_POINT('Ctrl Pts',(-1.34270948206139,1.,-1.6934684849664));
#29111=CARTESIAN_POINT('Ctrl Pts',(-1.34171037484673,1.,-1.68715660868602));
#29112=CARTESIAN_POINT('Ctrl Pts',(-1.3406748518516,1.,-1.68086176030308));
#29113=CARTESIAN_POINT('Ctrl Pts',(-1.33960273470372,1.,-1.67458429426126));
#29114=CARTESIAN_POINT('Ctrl Pts',(-1.33849388654458,1.,-1.66832460784078));
#29115=CARTESIAN_POINT('Ctrl Pts',(-1.33734820885331,1.,-1.66208312542073));
#29116=CARTESIAN_POINT('Ctrl Pts',(-1.33616559745217,1.,-1.65586025952651));
#29117=CARTESIAN_POINT('Ctrl Pts',(-1.33494590468003,1.,-1.64965637286843));
#29118=CARTESIAN_POINT('Ctrl Pts',(-1.33368890676554,1.,-1.64347174856007));
#29119=CARTESIAN_POINT('Ctrl Pts',(-1.33239425103694,1.,-1.6373065347505));
#29120=CARTESIAN_POINT('Ctrl Pts',(-1.33106149345618,1.,-1.63116079730887));
#29121=CARTESIAN_POINT('Ctrl Pts',(-1.32969019505665,1.,-1.62503464209777));
#29122=CARTESIAN_POINT('Ctrl Pts',(-1.32828000610448,1.,-1.61892832270723));
#29123=CARTESIAN_POINT('Ctrl Pts',(-1.32683074483365,1.,-1.61284234015762));
#29124=CARTESIAN_POINT('Ctrl Pts',(-1.32534250785794,1.,-1.6067775829097));
#29125=CARTESIAN_POINT('Ctrl Pts',(-1.32381550858266,1.,-1.600735118587));
#29126=CARTESIAN_POINT('Ctrl Pts',(-1.32224985747686,1.,-1.59471591079408));
#29127=CARTESIAN_POINT('Ctrl Pts',(-1.32064537110891,1.,-1.58872057258244));
#29128=CARTESIAN_POINT('Ctrl Pts',(-1.31900135021428,1.,-1.58274907898829));
#29129=CARTESIAN_POINT('Ctrl Pts',(-1.31731642317183,1.,-1.57680056505585));
#29130=CARTESIAN_POINT('Ctrl Pts',(-1.31558903860015,1.,-1.57087397835721));
#29131=CARTESIAN_POINT('Ctrl Pts',(-1.31381795281002,1.,-1.56496872402352));
#29132=CARTESIAN_POINT('Ctrl Pts',(-1.31200264341696,1.,-1.55908521254822));
#29133=CARTESIAN_POINT('Ctrl Pts',(-1.31014393684221,1.,-1.55322568759481));
#29134=CARTESIAN_POINT('Ctrl Pts',(-1.30824393907471,1.,-1.54739413957183));
#29135=CARTESIAN_POINT('Ctrl Pts',(-1.30630475189553,1.,-1.54159462645428));
#29136=CARTESIAN_POINT('Ctrl Pts',(-1.30432735639487,1.,-1.53582981268976));
#29137=CARTESIAN_POINT('Ctrl Pts',(-1.3023106439557,1.,-1.53009970283893));
#29138=CARTESIAN_POINT('Ctrl Pts',(-1.30024984366334,1.,-1.5243995786107));
#29139=CARTESIAN_POINT('Ctrl Pts',(-1.29813791800757,1.,-1.51872184912735));
#29140=CARTESIAN_POINT('Ctrl Pts',(-1.29596850710518,1.,-1.51305994241412));
#29141=CARTESIAN_POINT('Ctrl Pts',(-1.29373841372843,1.,-1.50741159078367));
#29142=CARTESIAN_POINT('Ctrl Pts',(-1.29145022885171,1.,-1.50178230149764));
#29143=CARTESIAN_POINT('Ctrl Pts',(-1.28911506584232,1.,-1.49618896881729));
#29144=CARTESIAN_POINT('Ctrl Pts',(-1.28674676116415,1.,-1.4906522831275));
#29145=CARTESIAN_POINT('Ctrl Pts',(-1.28435533880184,1.,-1.48518817118891));
#29146=CARTESIAN_POINT('Ctrl Pts',(-1.28194158939522,1.,-1.47980070347102));
#29147=CARTESIAN_POINT('Ctrl Pts',(-1.27948918248524,1.,-1.4744717526711));
#29148=CARTESIAN_POINT('Ctrl Pts',(-1.27696414831144,1.,-1.46916035917197));
#29149=CARTESIAN_POINT('Ctrl Pts',(-1.27433119897877,1.,-1.4638243133254));
#29150=CARTESIAN_POINT('Ctrl Pts',(-1.27156805265312,1.,-1.45843906294725));
#29151=CARTESIAN_POINT('Ctrl Pts',(-1.26867786804854,1.,-1.45301422764205));
#29152=CARTESIAN_POINT('Ctrl Pts',(-1.26570925118767,1.,-1.44761985001544));
#29153=CARTESIAN_POINT('Ctrl Pts',(-1.26273903323723,1.,-1.44236470511145));
#29154=CARTESIAN_POINT('Ctrl Pts',(-1.25983531011894,1.,-1.43734919180719));
#29155=CARTESIAN_POINT('Ctrl Pts',(-1.25702687965744,1.,-1.43262645609679));
#29156=CARTESIAN_POINT('Ctrl Pts',(-1.25426945222783,1.,-1.42815938799555));
#29157=CARTESIAN_POINT('Ctrl Pts',(-1.25141455570299,1.,-1.42378102115911));
#29158=CARTESIAN_POINT('Ctrl Pts',(-1.24824430986911,1.,-1.41923722596421));
#29159=CARTESIAN_POINT('Ctrl Pts',(-1.24450600513278,1.,-1.41422913175437));
#29160=CARTESIAN_POINT('Ctrl Pts',(-1.23994455029421,1.,-1.40845295531151));
#29161=CARTESIAN_POINT('Ctrl Pts',(-1.23434087289768,1.,-1.40164708205345));
#29162=CARTESIAN_POINT('Ctrl Pts',(-1.22752961898063,1.,-1.39361389567257));
#29163=CARTESIAN_POINT('Ctrl Pts',(-1.21938737278853,1.,-1.38420564525391));
#29164=CARTESIAN_POINT('Ctrl Pts',(-1.20982812923113,1.,-1.37331915604962));
#29165=CARTESIAN_POINT('Ctrl Pts',(-1.1987959077656,1.,-1.36088705040677));
#29166=CARTESIAN_POINT('Ctrl Pts',(-1.18625865664915,1.,-1.34687053998157));
#29167=CARTESIAN_POINT('Ctrl Pts',(-1.17501305787994,1.,-1.33437539344842));
#29168=CARTESIAN_POINT('Ctrl Pts',(-1.16589330092532,1.,-1.32428080720544));
#29169=CARTESIAN_POINT('Ctrl Pts',(-1.15950888730433,1.,-1.3172297721596));
#29170=CARTESIAN_POINT('Ctrl Pts',(-1.15624053661742,1.,-1.31362392696033));
#29171=CARTESIAN_POINT('',(-1.34869019493419,0.,-1.73811241238545));
#29172=CARTESIAN_POINT('Origin',(-1.23627494547115,0.,-1.81978687191668));
#29173=CARTESIAN_POINT('',(-1.23627494547115,1.,-1.81978687191668));
#29174=CARTESIAN_POINT('',(-1.34869019493419,1.,-1.73811241238545));
#29175=CARTESIAN_POINT('',(-1.23627494547115,0.,-1.81978687191668));
#29176=CARTESIAN_POINT('Ctrl Pts',(-0.892032620296855,-1.,-1.5055822144029));
#29177=CARTESIAN_POINT('Ctrl Pts',(-0.892032620296855,1.,-1.5055822144029));
#29178=CARTESIAN_POINT('Ctrl Pts',(-0.894452006967538,-1.,-1.50980486807181));
#29179=CARTESIAN_POINT('Ctrl Pts',(-0.894452006967538,1.,-1.50980486807181));
#29180=CARTESIAN_POINT('Ctrl Pts',(-0.89918504749193,-1.,-1.51805569591479));
#29181=CARTESIAN_POINT('Ctrl Pts',(-0.89918504749193,1.,-1.51805569591479));
#29182=CARTESIAN_POINT('Ctrl Pts',(-0.905967409640499,-1.,-1.52984849890434));
#29183=CARTESIAN_POINT('Ctrl Pts',(-0.905967409640499,1.,-1.52984849890434));
#29184=CARTESIAN_POINT('Ctrl Pts',(-0.91437591904658,-1.,-1.54440491152808));
#29185=CARTESIAN_POINT('Ctrl Pts',(-0.91437591904658,1.,-1.54440491152808));
#29186=CARTESIAN_POINT('Ctrl Pts',(-0.923832188966322,-1.,-1.56065988582509));
#29187=CARTESIAN_POINT('Ctrl Pts',(-0.923832188966322,1.,-1.56065988582509));
#29188=CARTESIAN_POINT('Ctrl Pts',(-0.932246680128849,-1.,-1.57499388385561));
#29189=CARTESIAN_POINT('Ctrl Pts',(-0.932246680128849,1.,-1.57499388385561));
#29190=CARTESIAN_POINT('Ctrl Pts',(-0.939646377909319,-1.,-1.58744937489796));
#29191=CARTESIAN_POINT('Ctrl Pts',(-0.939646377909319,1.,-1.58744937489796));
#29192=CARTESIAN_POINT('Ctrl Pts',(-0.946078063325796,-1.,-1.59810042045408));
#29193=CARTESIAN_POINT('Ctrl Pts',(-0.946078063325796,1.,-1.59810042045408));
#29194=CARTESIAN_POINT('Ctrl Pts',(-0.951613284361248,-1.,-1.60706069897794));
#29195=CARTESIAN_POINT('Ctrl Pts',(-0.951613284361248,1.,-1.60706069897794));
#29196=CARTESIAN_POINT('Ctrl Pts',(-0.956354422921573,-1.,-1.61449324337233));
#29197=CARTESIAN_POINT('Ctrl Pts',(-0.956354422921573,1.,-1.61449324337233));
#29198=CARTESIAN_POINT('Ctrl Pts',(-0.960438326099958,-1.,-1.62061638139929));
#29199=CARTESIAN_POINT('Ctrl Pts',(-0.960438326099958,1.,-1.62061638139929));
#29200=CARTESIAN_POINT('Ctrl Pts',(-0.964046107037821,-1.,-1.6257193066974));
#29201=CARTESIAN_POINT('Ctrl Pts',(-0.964046107037821,1.,-1.6257193066974));
#29202=CARTESIAN_POINT('Ctrl Pts',(-0.967387853228041,-1.,-1.63013849959083));
#29203=CARTESIAN_POINT('Ctrl Pts',(-0.967387853228041,1.,-1.63013849959083));
#29204=CARTESIAN_POINT('Ctrl Pts',(-0.970669715996356,-1.,-1.63420665729609));
#29205=CARTESIAN_POINT('Ctrl Pts',(-0.970669715996356,1.,-1.63420665729609));
#29206=CARTESIAN_POINT('Ctrl Pts',(-0.974066058287501,-1.,-1.63820952658157));
#29207=CARTESIAN_POINT('Ctrl Pts',(-0.974066058287501,1.,-1.63820952658157));
#29208=CARTESIAN_POINT('Ctrl Pts',(-0.977689794120297,-1.,-1.64233990826831));
#29209=CARTESIAN_POINT('Ctrl Pts',(-0.977689794120297,1.,-1.64233990826831));
#29210=CARTESIAN_POINT('Ctrl Pts',(-0.981562530940574,-1.,-1.64665139190834));
#29211=CARTESIAN_POINT('Ctrl Pts',(-0.981562530940574,1.,-1.64665139190834));
#29212=CARTESIAN_POINT('Ctrl Pts',(-0.985642622921626,-1.,-1.6511001661277));
#29213=CARTESIAN_POINT('Ctrl Pts',(-0.985642622921626,1.,-1.6511001661277));
#29214=CARTESIAN_POINT('Ctrl Pts',(-0.98985562785445,-1.,-1.65559044289746));
#29215=CARTESIAN_POINT('Ctrl Pts',(-0.98985562785445,1.,-1.65559044289746));
#29216=CARTESIAN_POINT('Ctrl Pts',(-0.994121836661116,-1.,-1.66001553809916));
#29217=CARTESIAN_POINT('Ctrl Pts',(-0.994121836661116,1.,-1.66001553809916));
#29218=CARTESIAN_POINT('Ctrl Pts',(-0.998389654952317,-1.,-1.66430758030304));
#29219=CARTESIAN_POINT('Ctrl Pts',(-0.998389654952317,1.,-1.66430758030304));
#29220=CARTESIAN_POINT('Ctrl Pts',(-1.00265091003682,-1.,-1.66846059277231));
#29221=CARTESIAN_POINT('Ctrl Pts',(-1.00265091003682,1.,-1.66846059277231));
#29222=CARTESIAN_POINT('Ctrl Pts',(-1.00692206696387,-1.,-1.67250335383248));
#29223=CARTESIAN_POINT('Ctrl Pts',(-1.00692206696387,1.,-1.67250335383248));
#29224=CARTESIAN_POINT('Ctrl Pts',(-1.01123236493507,-1.,-1.67648246776457));
#29225=CARTESIAN_POINT('Ctrl Pts',(-1.01123236493507,1.,-1.67648246776457));
#29226=CARTESIAN_POINT('Ctrl Pts',(-1.01561026162787,-1.,-1.6804428989482));
#29227=CARTESIAN_POINT('Ctrl Pts',(-1.01561026162787,1.,-1.6804428989482));
#29228=CARTESIAN_POINT('Ctrl Pts',(-1.02006795074222,-1.,-1.68440578021739));
#29229=CARTESIAN_POINT('Ctrl Pts',(-1.02006795074222,1.,-1.68440578021739));
#29230=CARTESIAN_POINT('Ctrl Pts',(-1.02460180535272,-1.,-1.68836910178475));
#29231=CARTESIAN_POINT('Ctrl Pts',(-1.02460180535272,1.,-1.68836910178475));
#29232=CARTESIAN_POINT('Ctrl Pts',(-1.02919977579155,-1.,-1.69231840863471));
#29233=CARTESIAN_POINT('Ctrl Pts',(-1.02919977579155,1.,-1.69231840863471));
#29234=CARTESIAN_POINT('Ctrl Pts',(-1.03384646003587,-1.,-1.69623414782769));
#29235=CARTESIAN_POINT('Ctrl Pts',(-1.03384646003587,1.,-1.69623414782769));
#29236=CARTESIAN_POINT('Ctrl Pts',(-1.03852922490782,-1.,-1.70010052930951));
#29237=CARTESIAN_POINT('Ctrl Pts',(-1.03852922490782,1.,-1.70010052930951));
#29238=CARTESIAN_POINT('Ctrl Pts',(-1.04324363334546,-1.,-1.70391338707969));
#29239=CARTESIAN_POINT('Ctrl Pts',(-1.04324363334546,1.,-1.70391338707969));
#29240=CARTESIAN_POINT('Ctrl Pts',(-1.0479908540499,-1.,-1.70767646263641));
#29241=CARTESIAN_POINT('Ctrl Pts',(-1.0479908540499,1.,-1.70767646263641));
#29242=CARTESIAN_POINT('Ctrl Pts',(-1.05277517202854,-1.,-1.71139783543986));
#29243=CARTESIAN_POINT('Ctrl Pts',(-1.05277517202854,1.,-1.71139783543986));
#29244=CARTESIAN_POINT('Ctrl Pts',(-1.05760163192481,-1.,-1.71508654427022));
#29245=CARTESIAN_POINT('Ctrl Pts',(-1.05760163192481,1.,-1.71508654427022));
#29246=CARTESIAN_POINT('Ctrl Pts',(-1.0624732468065,-1.,-1.71874858456908));
#29247=CARTESIAN_POINT('Ctrl Pts',(-1.0624732468065,1.,-1.71874858456908));
#29248=CARTESIAN_POINT('Ctrl Pts',(-1.06738966975463,-1.,-1.72238500928456));
#29249=CARTESIAN_POINT('Ctrl Pts',(-1.06738966975463,1.,-1.72238500928456));
#29250=CARTESIAN_POINT('Ctrl Pts',(-1.07234866990252,-1.,-1.72599406198489));
#29251=CARTESIAN_POINT('Ctrl Pts',(-1.07234866990252,1.,-1.72599406198489));
#29252=CARTESIAN_POINT('Ctrl Pts',(-1.0773470373727,-1.,-1.72957248977424));
#29253=CARTESIAN_POINT('Ctrl Pts',(-1.0773470373727,1.,-1.72957248977424));
#29254=CARTESIAN_POINT('Ctrl Pts',(-1.08238162784749,-1.,-1.73311705663407));
#29255=CARTESIAN_POINT('Ctrl Pts',(-1.08238162784749,1.,-1.73311705663407));
#29256=CARTESIAN_POINT('Ctrl Pts',(-1.08745056285429,-1.,-1.73662628326093));
#29257=CARTESIAN_POINT('Ctrl Pts',(-1.08745056285429,1.,-1.73662628326093));
#29258=CARTESIAN_POINT('Ctrl Pts',(-1.09255329056496,-1.,-1.74010053962252));
#29259=CARTESIAN_POINT('Ctrl Pts',(-1.09255329056496,1.,-1.74010053962252));
#29260=CARTESIAN_POINT('Ctrl Pts',(-1.09768999241229,-1.,-1.74354119236212));
#29261=CARTESIAN_POINT('Ctrl Pts',(-1.09768999241229,1.,-1.74354119236212));
#29262=CARTESIAN_POINT('Ctrl Pts',(-1.10286118991144,-1.,-1.74695004214924));
#29263=CARTESIAN_POINT('Ctrl Pts',(-1.10286118991144,1.,-1.74695004214924));
#29264=CARTESIAN_POINT('Ctrl Pts',(-1.10806728183003,-1.,-1.75032866075914));
#29265=CARTESIAN_POINT('Ctrl Pts',(-1.10806728183003,1.,-1.75032866075914));
#29266=CARTESIAN_POINT('Ctrl Pts',(-1.11330807582542,-1.,-1.75367772094617));
#29267=CARTESIAN_POINT('Ctrl Pts',(-1.11330807582542,1.,-1.75367772094617));
#29268=CARTESIAN_POINT('Ctrl Pts',(-1.11858293216752,-1.,-1.75699720772089));
#29269=CARTESIAN_POINT('Ctrl Pts',(-1.11858293216752,1.,-1.75699720772089));
#29270=CARTESIAN_POINT('Ctrl Pts',(-1.12389096855078,-1.,-1.76028671825084));
#29271=CARTESIAN_POINT('Ctrl Pts',(-1.12389096855078,1.,-1.76028671825084));
#29272=CARTESIAN_POINT('Ctrl Pts',(-1.12923123555076,-1.,-1.76354571966171));
#29273=CARTESIAN_POINT('Ctrl Pts',(-1.12923123555076,1.,-1.76354571966171));
#29274=CARTESIAN_POINT('Ctrl Pts',(-1.13460291804635,-1.,-1.76677384551883));
#29275=CARTESIAN_POINT('Ctrl Pts',(-1.13460291804635,1.,-1.76677384551883));
#29276=CARTESIAN_POINT('Ctrl Pts',(-1.14000548337,-1.,-1.76997111386806));
#29277=CARTESIAN_POINT('Ctrl Pts',(-1.14000548337,1.,-1.76997111386806));
#29278=CARTESIAN_POINT('Ctrl Pts',(-1.14543858226948,-1.,-1.77313777896234));
#29279=CARTESIAN_POINT('Ctrl Pts',(-1.14543858226948,1.,-1.77313777896234));
#29280=CARTESIAN_POINT('Ctrl Pts',(-1.15090197841531,-1.,-1.77627422557034));
#29281=CARTESIAN_POINT('Ctrl Pts',(-1.15090197841531,1.,-1.77627422557034));
#29282=CARTESIAN_POINT('Ctrl Pts',(-1.15639547194689,-1.,-1.77938085564261));
#29283=CARTESIAN_POINT('Ctrl Pts',(-1.15639547194689,1.,-1.77938085564261));
#29284=CARTESIAN_POINT('Ctrl Pts',(-1.16191881298458,-1.,-1.78245795880949));
#29285=CARTESIAN_POINT('Ctrl Pts',(-1.16191881298458,1.,-1.78245795880949));
#29286=CARTESIAN_POINT('Ctrl Pts',(-1.16747166312239,-1.,-1.78550566040349));
#29287=CARTESIAN_POINT('Ctrl Pts',(-1.16747166312239,1.,-1.78550566040349));
#29288=CARTESIAN_POINT('Ctrl Pts',(-1.17305363177265,-1.,-1.78852398877523));
#29289=CARTESIAN_POINT('Ctrl Pts',(-1.17305363177265,1.,-1.78852398877523));
#29290=CARTESIAN_POINT('Ctrl Pts',(-1.17866429440781,-1.,-1.79151291552646));
#29291=CARTESIAN_POINT('Ctrl Pts',(-1.17866429440781,1.,-1.79151291552646));
#29292=CARTESIAN_POINT('Ctrl Pts',(-1.18430321697471,-1.,-1.79447240321572));
#29293=CARTESIAN_POINT('Ctrl Pts',(-1.18430321697471,1.,-1.79447240321572));
#29294=CARTESIAN_POINT('Ctrl Pts',(-1.1899699793456,-1.,-1.79740245923649));
#29295=CARTESIAN_POINT('Ctrl Pts',(-1.1899699793456,1.,-1.79740245923649));
#29296=CARTESIAN_POINT('Ctrl Pts',(-1.19566418930405,-1.,-1.80030314370121));
#29297=CARTESIAN_POINT('Ctrl Pts',(-1.19566418930405,1.,-1.80030314370121));
#29298=CARTESIAN_POINT('Ctrl Pts',(-1.2013854893912,-1.,-1.8031745483882));
#29299=CARTESIAN_POINT('Ctrl Pts',(-1.2013854893912,1.,-1.8031745483882));
#29300=CARTESIAN_POINT('Ctrl Pts',(-1.20713356605519,-1.,-1.80601678480772));
#29301=CARTESIAN_POINT('Ctrl Pts',(-1.20713356605519,1.,-1.80601678480772));
#29302=CARTESIAN_POINT('Ctrl Pts',(-1.2129081570818,-1.,-1.80882996916931));
#29303=CARTESIAN_POINT('Ctrl Pts',(-1.2129081570818,1.,-1.80882996916931));
#29304=CARTESIAN_POINT('Ctrl Pts',(-1.2187090610323,-1.,-1.81161420806172));
#29305=CARTESIAN_POINT('Ctrl Pts',(-1.2187090610323,1.,-1.81161420806172));
#29306=CARTESIAN_POINT('Ctrl Pts',(-1.22453613304507,-1.,-1.81436959209778));
#29307=CARTESIAN_POINT('Ctrl Pts',(-1.22453613304507,1.,-1.81436959209778));
#29308=CARTESIAN_POINT('Ctrl Pts',(-1.22921864890975,-1.,-1.81655087183054));
#29309=CARTESIAN_POINT('Ctrl Pts',(-1.22921864890975,1.,-1.81655087183054));
#29310=CARTESIAN_POINT('Ctrl Pts',(-1.23274224526804,-1.,-1.81817389920914));
#29311=CARTESIAN_POINT('Ctrl Pts',(-1.23274224526804,1.,-1.81817389920914));
#29312=CARTESIAN_POINT('Ctrl Pts',(-1.23509651170384,-1.,-1.81925017193531));
#29313=CARTESIAN_POINT('Ctrl Pts',(-1.23509651170384,1.,-1.81925017193531));
#29314=CARTESIAN_POINT('Ctrl Pts',(-1.23627494547115,-1.,-1.81978687191668));
#29315=CARTESIAN_POINT('Ctrl Pts',(-1.23627494547115,1.,-1.81978687191668));
#29316=CARTESIAN_POINT('',(-0.892032620296855,1.,-1.5055822144029));
#29317=CARTESIAN_POINT('Ctrl Pts',(-0.892032620296855,1.,-1.5055822144029));
#29318=CARTESIAN_POINT('Ctrl Pts',(-0.894452006967538,1.,-1.50980486807181));
#29319=CARTESIAN_POINT('Ctrl Pts',(-0.89918504749193,1.,-1.51805569591479));
#29320=CARTESIAN_POINT('Ctrl Pts',(-0.905967409640499,1.,-1.52984849890434));
#29321=CARTESIAN_POINT('Ctrl Pts',(-0.91437591904658,1.,-1.54440491152808));
#29322=CARTESIAN_POINT('Ctrl Pts',(-0.923832188966322,1.,-1.56065988582509));
#29323=CARTESIAN_POINT('Ctrl Pts',(-0.932246680128849,1.,-1.57499388385561));
#29324=CARTESIAN_POINT('Ctrl Pts',(-0.939646377909319,1.,-1.58744937489796));
#29325=CARTESIAN_POINT('Ctrl Pts',(-0.946078063325796,1.,-1.59810042045408));
#29326=CARTESIAN_POINT('Ctrl Pts',(-0.951613284361248,1.,-1.60706069897794));
#29327=CARTESIAN_POINT('Ctrl Pts',(-0.956354422921573,1.,-1.61449324337233));
#29328=CARTESIAN_POINT('Ctrl Pts',(-0.960438326099958,1.,-1.62061638139929));
#29329=CARTESIAN_POINT('Ctrl Pts',(-0.964046107037821,1.,-1.6257193066974));
#29330=CARTESIAN_POINT('Ctrl Pts',(-0.967387853228041,1.,-1.63013849959083));
#29331=CARTESIAN_POINT('Ctrl Pts',(-0.970669715996356,1.,-1.63420665729609));
#29332=CARTESIAN_POINT('Ctrl Pts',(-0.974066058287501,1.,-1.63820952658157));
#29333=CARTESIAN_POINT('Ctrl Pts',(-0.977689794120297,1.,-1.64233990826831));
#29334=CARTESIAN_POINT('Ctrl Pts',(-0.981562530940574,1.,-1.64665139190834));
#29335=CARTESIAN_POINT('Ctrl Pts',(-0.985642622921626,1.,-1.6511001661277));
#29336=CARTESIAN_POINT('Ctrl Pts',(-0.98985562785445,1.,-1.65559044289746));
#29337=CARTESIAN_POINT('Ctrl Pts',(-0.994121836661116,1.,-1.66001553809916));
#29338=CARTESIAN_POINT('Ctrl Pts',(-0.998389654952317,1.,-1.66430758030304));
#29339=CARTESIAN_POINT('Ctrl Pts',(-1.00265091003682,1.,-1.66846059277231));
#29340=CARTESIAN_POINT('Ctrl Pts',(-1.00692206696387,1.,-1.67250335383248));
#29341=CARTESIAN_POINT('Ctrl Pts',(-1.01123236493507,1.,-1.67648246776457));
#29342=CARTESIAN_POINT('Ctrl Pts',(-1.01561026162787,1.,-1.6804428989482));
#29343=CARTESIAN_POINT('Ctrl Pts',(-1.02006795074222,1.,-1.68440578021739));
#29344=CARTESIAN_POINT('Ctrl Pts',(-1.02460180535272,1.,-1.68836910178475));
#29345=CARTESIAN_POINT('Ctrl Pts',(-1.02919977579155,1.,-1.69231840863471));
#29346=CARTESIAN_POINT('Ctrl Pts',(-1.03384646003587,1.,-1.69623414782769));
#29347=CARTESIAN_POINT('Ctrl Pts',(-1.03852922490782,1.,-1.70010052930951));
#29348=CARTESIAN_POINT('Ctrl Pts',(-1.04324363334546,1.,-1.70391338707969));
#29349=CARTESIAN_POINT('Ctrl Pts',(-1.0479908540499,1.,-1.70767646263641));
#29350=CARTESIAN_POINT('Ctrl Pts',(-1.05277517202854,1.,-1.71139783543986));
#29351=CARTESIAN_POINT('Ctrl Pts',(-1.05760163192481,1.,-1.71508654427022));
#29352=CARTESIAN_POINT('Ctrl Pts',(-1.0624732468065,1.,-1.71874858456908));
#29353=CARTESIAN_POINT('Ctrl Pts',(-1.06738966975463,1.,-1.72238500928456));
#29354=CARTESIAN_POINT('Ctrl Pts',(-1.07234866990252,1.,-1.72599406198489));
#29355=CARTESIAN_POINT('Ctrl Pts',(-1.0773470373727,1.,-1.72957248977424));
#29356=CARTESIAN_POINT('Ctrl Pts',(-1.08238162784749,1.,-1.73311705663407));
#29357=CARTESIAN_POINT('Ctrl Pts',(-1.08745056285429,1.,-1.73662628326093));
#29358=CARTESIAN_POINT('Ctrl Pts',(-1.09255329056496,1.,-1.74010053962252));
#29359=CARTESIAN_POINT('Ctrl Pts',(-1.09768999241229,1.,-1.74354119236212));
#29360=CARTESIAN_POINT('Ctrl Pts',(-1.10286118991144,1.,-1.74695004214924));
#29361=CARTESIAN_POINT('Ctrl Pts',(-1.10806728183003,1.,-1.75032866075914));
#29362=CARTESIAN_POINT('Ctrl Pts',(-1.11330807582542,1.,-1.75367772094617));
#29363=CARTESIAN_POINT('Ctrl Pts',(-1.11858293216752,1.,-1.75699720772089));
#29364=CARTESIAN_POINT('Ctrl Pts',(-1.12389096855078,1.,-1.76028671825084));
#29365=CARTESIAN_POINT('Ctrl Pts',(-1.12923123555076,1.,-1.76354571966171));
#29366=CARTESIAN_POINT('Ctrl Pts',(-1.13460291804635,1.,-1.76677384551883));
#29367=CARTESIAN_POINT('Ctrl Pts',(-1.14000548337,1.,-1.76997111386806));
#29368=CARTESIAN_POINT('Ctrl Pts',(-1.14543858226948,1.,-1.77313777896234));
#29369=CARTESIAN_POINT('Ctrl Pts',(-1.15090197841531,1.,-1.77627422557034));
#29370=CARTESIAN_POINT('Ctrl Pts',(-1.15639547194689,1.,-1.77938085564261));
#29371=CARTESIAN_POINT('Ctrl Pts',(-1.16191881298458,1.,-1.78245795880949));
#29372=CARTESIAN_POINT('Ctrl Pts',(-1.16747166312239,1.,-1.78550566040349));
#29373=CARTESIAN_POINT('Ctrl Pts',(-1.17305363177265,1.,-1.78852398877523));
#29374=CARTESIAN_POINT('Ctrl Pts',(-1.17866429440781,1.,-1.79151291552646));
#29375=CARTESIAN_POINT('Ctrl Pts',(-1.18430321697471,1.,-1.79447240321572));
#29376=CARTESIAN_POINT('Ctrl Pts',(-1.1899699793456,1.,-1.79740245923649));
#29377=CARTESIAN_POINT('Ctrl Pts',(-1.19566418930405,1.,-1.80030314370121));
#29378=CARTESIAN_POINT('Ctrl Pts',(-1.2013854893912,1.,-1.8031745483882));
#29379=CARTESIAN_POINT('Ctrl Pts',(-1.20713356605519,1.,-1.80601678480772));
#29380=CARTESIAN_POINT('Ctrl Pts',(-1.2129081570818,1.,-1.80882996916931));
#29381=CARTESIAN_POINT('Ctrl Pts',(-1.2187090610323,1.,-1.81161420806172));
#29382=CARTESIAN_POINT('Ctrl Pts',(-1.22453613304507,1.,-1.81436959209778));
#29383=CARTESIAN_POINT('Ctrl Pts',(-1.22921864890975,1.,-1.81655087183054));
#29384=CARTESIAN_POINT('Ctrl Pts',(-1.23274224526804,1.,-1.81817389920914));
#29385=CARTESIAN_POINT('Ctrl Pts',(-1.23509651170384,1.,-1.81925017193531));
#29386=CARTESIAN_POINT('Ctrl Pts',(-1.23627494547115,1.,-1.81978687191668));
#29387=CARTESIAN_POINT('',(-0.892032620296856,0.,-1.5055822144029));
#29388=CARTESIAN_POINT('Origin',(0.,0.,0.));
#29389=CARTESIAN_POINT('',(-0.693717979106305,1.,-1.60662857109684));
#29390=CARTESIAN_POINT('Origin',(0.,1.,0.));
#29391=CARTESIAN_POINT('',(-0.693717979106306,0.,-1.60662857109684));
#29392=CARTESIAN_POINT('Ctrl Pts',(-0.745574324794401,-1.,-2.0698113262342));
#29393=CARTESIAN_POINT('Ctrl Pts',(-0.745574324794401,1.,-2.0698113262342));
#29394=CARTESIAN_POINT('Ctrl Pts',(-0.745832791378367,-1.,-2.06854248895728));
#29395=CARTESIAN_POINT('Ctrl Pts',(-0.745832791378367,1.,-2.06854248895728));
#29396=CARTESIAN_POINT('Ctrl Pts',(-0.7463458715442,-1.,-2.06600523016815));
#29397=CARTESIAN_POINT('Ctrl Pts',(-0.7463458715442,1.,-2.06600523016815));
#29398=CARTESIAN_POINT('Ctrl Pts',(-0.747103932787919,-1.,-2.06220058927826));
#29399=CARTESIAN_POINT('Ctrl Pts',(-0.747103932787919,1.,-2.06220058927826));
#29400=CARTESIAN_POINT('Ctrl Pts',(-0.748091554183802,-1.,-2.05713023031006));
#29401=CARTESIAN_POINT('Ctrl Pts',(-0.748091554183802,1.,-2.05713023031006));
#29402=CARTESIAN_POINT('Ctrl Pts',(-0.749287468665046,-1.,-2.05079645592154));
#29403=CARTESIAN_POINT('Ctrl Pts',(-0.749287468665046,1.,-2.05079645592154));
#29404=CARTESIAN_POINT('Ctrl Pts',(-0.750444657875576,-1.,-2.04446689147979));
#29405=CARTESIAN_POINT('Ctrl Pts',(-0.750444657875576,1.,-2.04446689147979));
#29406=CARTESIAN_POINT('Ctrl Pts',(-0.751562963361115,-1.,-2.03814160092099));
#29407=CARTESIAN_POINT('Ctrl Pts',(-0.751562963361115,1.,-2.03814160092099));
#29408=CARTESIAN_POINT('Ctrl Pts',(-0.752642180487211,-1.,-2.03182068456221));
#29409=CARTESIAN_POINT('Ctrl Pts',(-0.752642180487211,1.,-2.03182068456221));
#29410=CARTESIAN_POINT('Ctrl Pts',(-0.753682061112768,-1.,-2.02550428623313));
#29411=CARTESIAN_POINT('Ctrl Pts',(-0.753682061112768,1.,-2.02550428623313));
#29412=CARTESIAN_POINT('Ctrl Pts',(-0.754682330722816,-1.,-2.01919259405809));
#29413=CARTESIAN_POINT('Ctrl Pts',(-0.754682330722816,1.,-2.01919259405809));
#29414=CARTESIAN_POINT('Ctrl Pts',(-0.755642704957865,-1.,-2.01288584328084));
#29415=CARTESIAN_POINT('Ctrl Pts',(-0.755642704957865,1.,-2.01288584328084));
#29416=CARTESIAN_POINT('Ctrl Pts',(-0.75656290464667,-1.,-2.0065843158773));
#29417=CARTESIAN_POINT('Ctrl Pts',(-0.75656290464667,1.,-2.0065843158773));
#29418=CARTESIAN_POINT('Ctrl Pts',(-0.757442676862724,-1.,-2.00028834739178));
#29419=CARTESIAN_POINT('Ctrl Pts',(-0.757442676862724,1.,-2.00028834739178));
#29420=CARTESIAN_POINT('Ctrl Pts',(-0.758281796766761,-1.,-1.99399831098817));
#29421=CARTESIAN_POINT('Ctrl Pts',(-0.758281796766761,1.,-1.99399831098817));
#29422=CARTESIAN_POINT('Ctrl Pts',(-0.759080037802488,-1.,-1.98771456680874));
#29423=CARTESIAN_POINT('Ctrl Pts',(-0.759080037802488,1.,-1.98771456680874));
#29424=CARTESIAN_POINT('Ctrl Pts',(-0.75983714745219,-1.,-1.98143741418172));
#29425=CARTESIAN_POINT('Ctrl Pts',(-0.75983714745219,1.,-1.98143741418172));
#29426=CARTESIAN_POINT('Ctrl Pts',(-0.760552825409757,-1.,-1.97516705321494));
#29427=CARTESIAN_POINT('Ctrl Pts',(-0.760552825409757,1.,-1.97516705321494));
#29428=CARTESIAN_POINT('Ctrl Pts',(-0.76122669048382,-1.,-1.96890351582499));
#29429=CARTESIAN_POINT('Ctrl Pts',(-0.76122669048382,1.,-1.96890351582499));
#29430=CARTESIAN_POINT('Ctrl Pts',(-0.761858300014423,-1.,-1.96264672744186));
#29431=CARTESIAN_POINT('Ctrl Pts',(-0.761858300014423,1.,-1.96264672744186));
#29432=CARTESIAN_POINT('Ctrl Pts',(-0.762447203806179,-1.,-1.95639665309869));
#29433=CARTESIAN_POINT('Ctrl Pts',(-0.762447203806179,1.,-1.95639665309869));
#29434=CARTESIAN_POINT('Ctrl Pts',(-0.762992990878769,-1.,-1.95015342590024));
#29435=CARTESIAN_POINT('Ctrl Pts',(-0.762992990878769,1.,-1.95015342590024));
#29436=CARTESIAN_POINT('Ctrl Pts',(-0.763495333538629,-1.,-1.9439174661764));
#29437=CARTESIAN_POINT('Ctrl Pts',(-0.763495333538629,1.,-1.9439174661764));
#29438=CARTESIAN_POINT('Ctrl Pts',(-0.763954049121458,-1.,-1.93768964875886));
#29439=CARTESIAN_POINT('Ctrl Pts',(-0.763954049121458,1.,-1.93768964875886));
#29440=CARTESIAN_POINT('Ctrl Pts',(-0.764369010673941,-1.,-1.93147105496382));
#29441=CARTESIAN_POINT('Ctrl Pts',(-0.764369010673941,1.,-1.93147105496382));
#29442=CARTESIAN_POINT('Ctrl Pts',(-0.764740025488211,-1.,-1.92526263537048));
#29443=CARTESIAN_POINT('Ctrl Pts',(-0.764740025488211,1.,-1.92526263537048));
#29444=CARTESIAN_POINT('Ctrl Pts',(-0.765066729667088,-1.,-1.91906491634196));
#29445=CARTESIAN_POINT('Ctrl Pts',(-0.765066729667088,1.,-1.91906491634196));
#29446=CARTESIAN_POINT('Ctrl Pts',(-0.765348465884722,-1.,-1.91287765805169));
#29447=CARTESIAN_POINT('Ctrl Pts',(-0.765348465884722,1.,-1.91287765805169));
#29448=CARTESIAN_POINT('Ctrl Pts',(-0.765584196937919,-1.,-1.90669961402356));
#29449=CARTESIAN_POINT('Ctrl Pts',(-0.765584196937919,1.,-1.90669961402356));
#29450=CARTESIAN_POINT('Ctrl Pts',(-0.765772772593386,-1.,-1.90052930393596));
#29451=CARTESIAN_POINT('Ctrl Pts',(-0.765772772593386,1.,-1.90052930393596));
#29452=CARTESIAN_POINT('Ctrl Pts',(-0.765913193856978,-1.,-1.89436577771388));
#29453=CARTESIAN_POINT('Ctrl Pts',(-0.765913193856978,1.,-1.89436577771388));
#29454=CARTESIAN_POINT('Ctrl Pts',(-0.766004837062091,-1.,-1.88820926433409));
#29455=CARTESIAN_POINT('Ctrl Pts',(-0.766004837062091,1.,-1.88820926433409));
#29456=CARTESIAN_POINT('Ctrl Pts',(-0.766047794851865,-1.,-1.88206215302561));
#29457=CARTESIAN_POINT('Ctrl Pts',(-0.766047794851865,1.,-1.88206215302561));
#29458=CARTESIAN_POINT('Ctrl Pts',(-0.766042837036744,-1.,-1.87592888967883));
#29459=CARTESIAN_POINT('Ctrl Pts',(-0.766042837036744,1.,-1.87592888967883));
#29460=CARTESIAN_POINT('Ctrl Pts',(-0.765990708546091,-1.,-1.86981398314341));
#29461=CARTESIAN_POINT('Ctrl Pts',(-0.765990708546091,1.,-1.86981398314341));
#29462=CARTESIAN_POINT('Ctrl Pts',(-0.765891519092547,-1.,-1.86372027063312));
#29463=CARTESIAN_POINT('Ctrl Pts',(-0.765891519092547,1.,-1.86372027063312));
#29464=CARTESIAN_POINT('Ctrl Pts',(-0.765744212909318,-1.,-1.85764741390394));
#29465=CARTESIAN_POINT('Ctrl Pts',(-0.765744212909318,1.,-1.85764741390394));
#29466=CARTESIAN_POINT('Ctrl Pts',(-0.765545710619062,-1.,-1.85158945130063));
#29467=CARTESIAN_POINT('Ctrl Pts',(-0.765545710619062,1.,-1.85158945130063));
#29468=CARTESIAN_POINT('Ctrl Pts',(-0.765291664862029,-1.,-1.84553698875924));
#29469=CARTESIAN_POINT('Ctrl Pts',(-0.765291664862029,1.,-1.84553698875924));
#29470=CARTESIAN_POINT('Ctrl Pts',(-0.764978057881737,-1.,-1.83948181064835));
#29471=CARTESIAN_POINT('Ctrl Pts',(-0.764978057881737,1.,-1.83948181064835));
#29472=CARTESIAN_POINT('Ctrl Pts',(-0.764602549687853,-1.,-1.83342077227142));
#29473=CARTESIAN_POINT('Ctrl Pts',(-0.764602549687853,1.,-1.83342077227142));
#29474=CARTESIAN_POINT('Ctrl Pts',(-0.764165902605995,-1.,-1.82735991200065));
#29475=CARTESIAN_POINT('Ctrl Pts',(-0.764165902605995,1.,-1.82735991200065));
#29476=CARTESIAN_POINT('Ctrl Pts',(-0.763673465462726,-1.,-1.82131873145266));
#29477=CARTESIAN_POINT('Ctrl Pts',(-0.763673465462726,1.,-1.82131873145266));
#29478=CARTESIAN_POINT('Ctrl Pts',(-0.763132003836634,-1.,-1.8153211840553));
#29479=CARTESIAN_POINT('Ctrl Pts',(-0.763132003836634,1.,-1.8153211840553));
#29480=CARTESIAN_POINT('Ctrl Pts',(-0.762546129463938,-1.,-1.80938551463965));
#29481=CARTESIAN_POINT('Ctrl Pts',(-0.762546129463938,1.,-1.80938551463965));
#29482=CARTESIAN_POINT('Ctrl Pts',(-0.761915336443547,-1.,-1.80351583877342));
#29483=CARTESIAN_POINT('Ctrl Pts',(-0.761915336443547,1.,-1.80351583877342));
#29484=CARTESIAN_POINT('Ctrl Pts',(-0.761229695230558,-1.,-1.79768986997783));
#29485=CARTESIAN_POINT('Ctrl Pts',(-0.761229695230558,1.,-1.79768986997783));
#29486=CARTESIAN_POINT('Ctrl Pts',(-0.760469555880749,-1.,-1.7918581561088));
#29487=CARTESIAN_POINT('Ctrl Pts',(-0.760469555880749,1.,-1.7918581561088));
#29488=CARTESIAN_POINT('Ctrl Pts',(-0.759614401110189,-1.,-1.78596964884604));
#29489=CARTESIAN_POINT('Ctrl Pts',(-0.759614401110189,1.,-1.78596964884604));
#29490=CARTESIAN_POINT('Ctrl Pts',(-0.758650626677518,-1.,-1.77999411220945));
#29491=CARTESIAN_POINT('Ctrl Pts',(-0.758650626677518,1.,-1.77999411220945));
#29492=CARTESIAN_POINT('Ctrl Pts',(-0.757578264077029,-1.,-1.77394167108292));
#29493=CARTESIAN_POINT('Ctrl Pts',(-0.757578264077029,1.,-1.77394167108292));
#29494=CARTESIAN_POINT('Ctrl Pts',(-0.75642189602781,-1.,-1.76789396002998));
#29495=CARTESIAN_POINT('Ctrl Pts',(-0.75642189602781,1.,-1.76789396002998));
#29496=CARTESIAN_POINT('Ctrl Pts',(-0.755220979974461,-1.,-1.76197817240128));
#29497=CARTESIAN_POINT('Ctrl Pts',(-0.755220979974461,1.,-1.76197817240128));
#29498=CARTESIAN_POINT('Ctrl Pts',(-0.754009254027829,-1.,-1.75631083600019));
#29499=CARTESIAN_POINT('Ctrl Pts',(-0.754009254027829,1.,-1.75631083600019));
#29500=CARTESIAN_POINT('Ctrl Pts',(-0.752797683531314,-1.,-1.75095139468794));
#29501=CARTESIAN_POINT('Ctrl Pts',(-0.752797683531314,1.,-1.75095139468794));
#29502=CARTESIAN_POINT('Ctrl Pts',(-0.751555614164482,-1.,-1.74585086852502));
#29503=CARTESIAN_POINT('Ctrl Pts',(-0.751555614164482,1.,-1.74585086852502));
#29504=CARTESIAN_POINT('Ctrl Pts',(-0.750193435981249,-1.,-1.74080458267114));
#29505=CARTESIAN_POINT('Ctrl Pts',(-0.750193435981249,1.,-1.74080458267114));
#29506=CARTESIAN_POINT('Ctrl Pts',(-0.74858246295687,-1.,-1.7355035168033));
#29507=CARTESIAN_POINT('Ctrl Pts',(-0.74858246295687,1.,-1.7355035168033));
#29508=CARTESIAN_POINT('Ctrl Pts',(-0.746574710097752,-1.,-1.72958533647714));
#29509=CARTESIAN_POINT('Ctrl Pts',(-0.746574710097752,1.,-1.72958533647714));
#29510=CARTESIAN_POINT('Ctrl Pts',(-0.744021445433093,-1.,-1.72268229916769));
#29511=CARTESIAN_POINT('Ctrl Pts',(-0.744021445433093,1.,-1.72268229916769));
#29512=CARTESIAN_POINT('Ctrl Pts',(-0.74079516202821,-1.,-1.71447789751001));
#29513=CARTESIAN_POINT('Ctrl Pts',(-0.74079516202821,1.,-1.71447789751001));
#29514=CARTESIAN_POINT('Ctrl Pts',(-0.736799665716932,-1.,-1.70473309004249));
#29515=CARTESIAN_POINT('Ctrl Pts',(-0.736799665716932,1.,-1.70473309004249));
#29516=CARTESIAN_POINT('Ctrl Pts',(-0.731963238685357,-1.,-1.69326921972915));
#29517=CARTESIAN_POINT('Ctrl Pts',(-0.731963238685357,1.,-1.69326921972915));
#29518=CARTESIAN_POINT('Ctrl Pts',(-0.726235967982445,-1.,-1.67996158451922));
#29519=CARTESIAN_POINT('Ctrl Pts',(-0.726235967982445,1.,-1.67996158451922));
#29520=CARTESIAN_POINT('Ctrl Pts',(-0.71958543378795,-1.,-1.66472880551777));
#29521=CARTESIAN_POINT('Ctrl Pts',(-0.71958543378795,1.,-1.66472880551777));
#29522=CARTESIAN_POINT('Ctrl Pts',(-0.711993139340447,-1.,-1.64752408828442));
#29523=CARTESIAN_POINT('Ctrl Pts',(-0.711993139340447,1.,-1.64752408828442));
#29524=CARTESIAN_POINT('Ctrl Pts',(-0.705159151977294,-1.,-1.6321654166204));
#29525=CARTESIAN_POINT('Ctrl Pts',(-0.705159151977294,1.,-1.6321654166204));
#29526=CARTESIAN_POINT('Ctrl Pts',(-0.699605146398837,-1.,-1.61974673471117));
#29527=CARTESIAN_POINT('Ctrl Pts',(-0.699605146398837,1.,-1.61974673471117));
#29528=CARTESIAN_POINT('Ctrl Pts',(-0.69571209787897,-1.,-1.61106790957619));
#29529=CARTESIAN_POINT('Ctrl Pts',(-0.69571209787897,1.,-1.61106790957619));
#29530=CARTESIAN_POINT('Ctrl Pts',(-0.693717979106305,-1.,-1.60662857109684));
#29531=CARTESIAN_POINT('Ctrl Pts',(-0.693717979106305,1.,-1.60662857109684));
#29532=CARTESIAN_POINT('',(-0.745574324794401,1.,-2.0698113262342));
#29533=CARTESIAN_POINT('Ctrl Pts',(-0.745574324794401,1.,-2.0698113262342));
#29534=CARTESIAN_POINT('Ctrl Pts',(-0.745832791378367,1.,-2.06854248895728));
#29535=CARTESIAN_POINT('Ctrl Pts',(-0.7463458715442,1.,-2.06600523016815));
#29536=CARTESIAN_POINT('Ctrl Pts',(-0.747103932787919,1.,-2.06220058927826));
#29537=CARTESIAN_POINT('Ctrl Pts',(-0.748091554183802,1.,-2.05713023031006));
#29538=CARTESIAN_POINT('Ctrl Pts',(-0.749287468665046,1.,-2.05079645592154));
#29539=CARTESIAN_POINT('Ctrl Pts',(-0.750444657875576,1.,-2.04446689147979));
#29540=CARTESIAN_POINT('Ctrl Pts',(-0.751562963361115,1.,-2.03814160092099));
#29541=CARTESIAN_POINT('Ctrl Pts',(-0.752642180487211,1.,-2.03182068456221));
#29542=CARTESIAN_POINT('Ctrl Pts',(-0.753682061112768,1.,-2.02550428623313));
#29543=CARTESIAN_POINT('Ctrl Pts',(-0.754682330722816,1.,-2.01919259405809));
#29544=CARTESIAN_POINT('Ctrl Pts',(-0.755642704957865,1.,-2.01288584328084));
#29545=CARTESIAN_POINT('Ctrl Pts',(-0.75656290464667,1.,-2.0065843158773));
#29546=CARTESIAN_POINT('Ctrl Pts',(-0.757442676862724,1.,-2.00028834739178));
#29547=CARTESIAN_POINT('Ctrl Pts',(-0.758281796766761,1.,-1.99399831098817));
#29548=CARTESIAN_POINT('Ctrl Pts',(-0.759080037802488,1.,-1.98771456680874));
#29549=CARTESIAN_POINT('Ctrl Pts',(-0.75983714745219,1.,-1.98143741418172));
#29550=CARTESIAN_POINT('Ctrl Pts',(-0.760552825409757,1.,-1.97516705321494));
#29551=CARTESIAN_POINT('Ctrl Pts',(-0.76122669048382,1.,-1.96890351582499));
#29552=CARTESIAN_POINT('Ctrl Pts',(-0.761858300014423,1.,-1.96264672744186));
#29553=CARTESIAN_POINT('Ctrl Pts',(-0.762447203806179,1.,-1.95639665309869));
#29554=CARTESIAN_POINT('Ctrl Pts',(-0.762992990878769,1.,-1.95015342590024));
#29555=CARTESIAN_POINT('Ctrl Pts',(-0.763495333538629,1.,-1.9439174661764));
#29556=CARTESIAN_POINT('Ctrl Pts',(-0.763954049121458,1.,-1.93768964875886));
#29557=CARTESIAN_POINT('Ctrl Pts',(-0.764369010673941,1.,-1.93147105496382));
#29558=CARTESIAN_POINT('Ctrl Pts',(-0.764740025488211,1.,-1.92526263537048));
#29559=CARTESIAN_POINT('Ctrl Pts',(-0.765066729667088,1.,-1.91906491634196));
#29560=CARTESIAN_POINT('Ctrl Pts',(-0.765348465884722,1.,-1.91287765805169));
#29561=CARTESIAN_POINT('Ctrl Pts',(-0.765584196937919,1.,-1.90669961402356));
#29562=CARTESIAN_POINT('Ctrl Pts',(-0.765772772593386,1.,-1.90052930393596));
#29563=CARTESIAN_POINT('Ctrl Pts',(-0.765913193856978,1.,-1.89436577771388));
#29564=CARTESIAN_POINT('Ctrl Pts',(-0.766004837062091,1.,-1.88820926433409));
#29565=CARTESIAN_POINT('Ctrl Pts',(-0.766047794851865,1.,-1.88206215302561));
#29566=CARTESIAN_POINT('Ctrl Pts',(-0.766042837036744,1.,-1.87592888967883));
#29567=CARTESIAN_POINT('Ctrl Pts',(-0.765990708546091,1.,-1.86981398314341));
#29568=CARTESIAN_POINT('Ctrl Pts',(-0.765891519092547,1.,-1.86372027063312));
#29569=CARTESIAN_POINT('Ctrl Pts',(-0.765744212909318,1.,-1.85764741390394));
#29570=CARTESIAN_POINT('Ctrl Pts',(-0.765545710619062,1.,-1.85158945130063));
#29571=CARTESIAN_POINT('Ctrl Pts',(-0.765291664862029,1.,-1.84553698875924));
#29572=CARTESIAN_POINT('Ctrl Pts',(-0.764978057881737,1.,-1.83948181064835));
#29573=CARTESIAN_POINT('Ctrl Pts',(-0.764602549687853,1.,-1.83342077227142));
#29574=CARTESIAN_POINT('Ctrl Pts',(-0.764165902605995,1.,-1.82735991200065));
#29575=CARTESIAN_POINT('Ctrl Pts',(-0.763673465462726,1.,-1.82131873145266));
#29576=CARTESIAN_POINT('Ctrl Pts',(-0.763132003836634,1.,-1.8153211840553));
#29577=CARTESIAN_POINT('Ctrl Pts',(-0.762546129463938,1.,-1.80938551463965));
#29578=CARTESIAN_POINT('Ctrl Pts',(-0.761915336443547,1.,-1.80351583877342));
#29579=CARTESIAN_POINT('Ctrl Pts',(-0.761229695230558,1.,-1.79768986997783));
#29580=CARTESIAN_POINT('Ctrl Pts',(-0.760469555880749,1.,-1.7918581561088));
#29581=CARTESIAN_POINT('Ctrl Pts',(-0.759614401110189,1.,-1.78596964884604));
#29582=CARTESIAN_POINT('Ctrl Pts',(-0.758650626677518,1.,-1.77999411220945));
#29583=CARTESIAN_POINT('Ctrl Pts',(-0.757578264077029,1.,-1.77394167108292));
#29584=CARTESIAN_POINT('Ctrl Pts',(-0.75642189602781,1.,-1.76789396002998));
#29585=CARTESIAN_POINT('Ctrl Pts',(-0.755220979974461,1.,-1.76197817240128));
#29586=CARTESIAN_POINT('Ctrl Pts',(-0.754009254027829,1.,-1.75631083600019));
#29587=CARTESIAN_POINT('Ctrl Pts',(-0.752797683531314,1.,-1.75095139468794));
#29588=CARTESIAN_POINT('Ctrl Pts',(-0.751555614164482,1.,-1.74585086852502));
#29589=CARTESIAN_POINT('Ctrl Pts',(-0.750193435981249,1.,-1.74080458267114));
#29590=CARTESIAN_POINT('Ctrl Pts',(-0.74858246295687,1.,-1.7355035168033));
#29591=CARTESIAN_POINT('Ctrl Pts',(-0.746574710097752,1.,-1.72958533647714));
#29592=CARTESIAN_POINT('Ctrl Pts',(-0.744021445433093,1.,-1.72268229916769));
#29593=CARTESIAN_POINT('Ctrl Pts',(-0.74079516202821,1.,-1.71447789751001));
#29594=CARTESIAN_POINT('Ctrl Pts',(-0.736799665716932,1.,-1.70473309004249));
#29595=CARTESIAN_POINT('Ctrl Pts',(-0.731963238685357,1.,-1.69326921972915));
#29596=CARTESIAN_POINT('Ctrl Pts',(-0.726235967982445,1.,-1.67996158451922));
#29597=CARTESIAN_POINT('Ctrl Pts',(-0.71958543378795,1.,-1.66472880551777));
#29598=CARTESIAN_POINT('Ctrl Pts',(-0.711993139340447,1.,-1.64752408828442));
#29599=CARTESIAN_POINT('Ctrl Pts',(-0.705159151977294,1.,-1.6321654166204));
#29600=CARTESIAN_POINT('Ctrl Pts',(-0.699605146398837,1.,-1.61974673471117));
#29601=CARTESIAN_POINT('Ctrl Pts',(-0.69571209787897,1.,-1.61106790957619));
#29602=CARTESIAN_POINT('Ctrl Pts',(-0.693717979106305,1.,-1.60662857109684));
#29603=CARTESIAN_POINT('',(-0.745574324794401,0.,-2.0698113262342));
#29604=CARTESIAN_POINT('Origin',(-0.61342227326009,0.,-2.11275013067528));
#29605=CARTESIAN_POINT('',(-0.61342227326009,1.,-2.11275013067528));
#29606=CARTESIAN_POINT('',(-0.745574324794401,1.,-2.0698113262342));
#29607=CARTESIAN_POINT('',(-0.61342227326009,0.,-2.11275013067528));
#29608=CARTESIAN_POINT('Ctrl Pts',(-0.383122945602004,-1.,-1.7075470150345));
#29609=CARTESIAN_POINT('Ctrl Pts',(-0.383122945602004,1.,-1.7075470150345));
#29610=CARTESIAN_POINT('Ctrl Pts',(-0.384119047315542,-1.,-1.71231062891958));
#29611=CARTESIAN_POINT('Ctrl Pts',(-0.384119047315542,1.,-1.71231062891958));
#29612=CARTESIAN_POINT('Ctrl Pts',(-0.38607079032701,-1.,-1.72162022246158));
#29613=CARTESIAN_POINT('Ctrl Pts',(-0.38607079032701,1.,-1.72162022246158));
#29614=CARTESIAN_POINT('Ctrl Pts',(-0.388877023509191,-1.,-1.7349317097561));
#29615=CARTESIAN_POINT('Ctrl Pts',(-0.388877023509191,1.,-1.7349317097561));
#29616=CARTESIAN_POINT('Ctrl Pts',(-0.392375812294307,-1.,-1.75137405313962));
#29617=CARTESIAN_POINT('Ctrl Pts',(-0.392375812294307,1.,-1.75137405313962));
#29618=CARTESIAN_POINT('Ctrl Pts',(-0.39634619612042,-1.,-1.7697556004756));
#29619=CARTESIAN_POINT('Ctrl Pts',(-0.39634619612042,1.,-1.7697556004756));
#29620=CARTESIAN_POINT('Ctrl Pts',(-0.39991940378308,-1.,-1.78598826347533));
#29621=CARTESIAN_POINT('Ctrl Pts',(-0.39991940378308,1.,-1.78598826347533));
#29622=CARTESIAN_POINT('Ctrl Pts',(-0.403107976170441,-1.,-1.80012077176221));
#29623=CARTESIAN_POINT('Ctrl Pts',(-0.403107976170441,1.,-1.80012077176221));
#29624=CARTESIAN_POINT('Ctrl Pts',(-0.405933518411838,-1.,-1.81223801813988));
#29625=CARTESIAN_POINT('Ctrl Pts',(-0.405933518411838,1.,-1.81223801813988));
#29626=CARTESIAN_POINT('Ctrl Pts',(-0.408428948108533,-1.,-1.8224702267854));
#29627=CARTESIAN_POINT('Ctrl Pts',(-0.408428948108533,1.,-1.8224702267854));
#29628=CARTESIAN_POINT('Ctrl Pts',(-0.410641256301675,-1.,-1.83100408895216));
#29629=CARTESIAN_POINT('Ctrl Pts',(-0.410641256301675,1.,-1.83100408895216));
#29630=CARTESIAN_POINT('Ctrl Pts',(-0.412633125322162,-1.,-1.83808953475839));
#29631=CARTESIAN_POINT('Ctrl Pts',(-0.412633125322162,1.,-1.83808953475839));
#29632=CARTESIAN_POINT('Ctrl Pts',(-0.41448743825434,-1.,-1.8440575707371));
#29633=CARTESIAN_POINT('Ctrl Pts',(-0.41448743825434,1.,-1.8440575707371));
#29634=CARTESIAN_POINT('Ctrl Pts',(-0.416300022038864,-1.,-1.84929312929882));
#29635=CARTESIAN_POINT('Ctrl Pts',(-0.416300022038864,1.,-1.84929312929882));
#29636=CARTESIAN_POINT('Ctrl Pts',(-0.418164129143534,-1.,-1.85417632856234));
#29637=CARTESIAN_POINT('Ctrl Pts',(-0.418164129143534,1.,-1.85417632856234));
#29638=CARTESIAN_POINT('Ctrl Pts',(-0.420157287975619,-1.,-1.85903281096686));
#29639=CARTESIAN_POINT('Ctrl Pts',(-0.420157287975619,1.,-1.85903281096686));
#29640=CARTESIAN_POINT('Ctrl Pts',(-0.422327307418275,-1.,-1.86408083334028));
#29641=CARTESIAN_POINT('Ctrl Pts',(-0.422327307418275,1.,-1.86408083334028));
#29642=CARTESIAN_POINT('Ctrl Pts',(-0.424678177291359,-1.,-1.86937803944323));
#29643=CARTESIAN_POINT('Ctrl Pts',(-0.424678177291359,1.,-1.86937803944323));
#29644=CARTESIAN_POINT('Ctrl Pts',(-0.427183828519102,-1.,-1.87486989291484));
#29645=CARTESIAN_POINT('Ctrl Pts',(-0.427183828519102,1.,-1.87486989291484));
#29646=CARTESIAN_POINT('Ctrl Pts',(-0.429803062482344,-1.,-1.88044229001832));
#29647=CARTESIAN_POINT('Ctrl Pts',(-0.429803062482344,1.,-1.88044229001832));
#29648=CARTESIAN_POINT('Ctrl Pts',(-0.432493038548748,-1.,-1.88596913666793));
#29649=CARTESIAN_POINT('Ctrl Pts',(-0.432493038548748,1.,-1.88596913666793));
#29650=CARTESIAN_POINT('Ctrl Pts',(-0.435225660963383,-1.,-1.89136993975504));
#29651=CARTESIAN_POINT('Ctrl Pts',(-0.435225660963383,1.,-1.89136993975504));
#29652=CARTESIAN_POINT('Ctrl Pts',(-0.437995003948244,-1.,-1.89663648956466));
#29653=CARTESIAN_POINT('Ctrl Pts',(-0.437995003948244,1.,-1.89663648956466));
#29654=CARTESIAN_POINT('Ctrl Pts',(-0.440807833704038,-1.,-1.90180124389086));
#29655=CARTESIAN_POINT('Ctrl Pts',(-0.440807833704038,1.,-1.90180124389086));
#29656=CARTESIAN_POINT('Ctrl Pts',(-0.443677556849151,-1.,-1.90691756144898));
#29657=CARTESIAN_POINT('Ctrl Pts',(-0.443677556849151,1.,-1.90691756144898));
#29658=CARTESIAN_POINT('Ctrl Pts',(-0.446617343485711,-1.,-1.9120369998112));
#29659=CARTESIAN_POINT('Ctrl Pts',(-0.446617343485711,1.,-1.9120369998112));
#29660=CARTESIAN_POINT('Ctrl Pts',(-0.449632260106662,-1.,-1.91718342555755));
#29661=CARTESIAN_POINT('Ctrl Pts',(-0.449632260106662,1.,-1.91718342555755));
#29662=CARTESIAN_POINT('Ctrl Pts',(-0.452719478359432,-1.,-1.92235380648502));
#29663=CARTESIAN_POINT('Ctrl Pts',(-0.452719478359432,1.,-1.92235380648502));
#29664=CARTESIAN_POINT('Ctrl Pts',(-0.455872005174371,-1.,-1.92753067150476));
#29665=CARTESIAN_POINT('Ctrl Pts',(-0.455872005174371,1.,-1.92753067150476));
#29666=CARTESIAN_POINT('Ctrl Pts',(-0.459081234547926,-1.,-1.93269066517934));
#29667=CARTESIAN_POINT('Ctrl Pts',(-0.459081234547926,1.,-1.93269066517934));
#29668=CARTESIAN_POINT('Ctrl Pts',(-0.462340031009056,-1.,-1.93781486640821));
#29669=CARTESIAN_POINT('Ctrl Pts',(-0.462340031009056,1.,-1.93781486640821));
#29670=CARTESIAN_POINT('Ctrl Pts',(-0.46564546202603,-1.,-1.9428979419619));
#29671=CARTESIAN_POINT('Ctrl Pts',(-0.46564546202603,1.,-1.9428979419619));
#29672=CARTESIAN_POINT('Ctrl Pts',(-0.468997482913135,-1.,-1.94794381136514));
#29673=CARTESIAN_POINT('Ctrl Pts',(-0.468997482913135,1.,-1.94794381136514));
#29674=CARTESIAN_POINT('Ctrl Pts',(-0.472397672264072,-1.,-1.95296148278133));
#29675=CARTESIAN_POINT('Ctrl Pts',(-0.472397672264072,1.,-1.95296148278133));
#29676=CARTESIAN_POINT('Ctrl Pts',(-0.475848034683176,-1.,-1.95796111148177));
#29677=CARTESIAN_POINT('Ctrl Pts',(-0.475848034683176,1.,-1.95796111148177));
#29678=CARTESIAN_POINT('Ctrl Pts',(-0.479349583074855,-1.,-1.96294933055943));
#29679=CARTESIAN_POINT('Ctrl Pts',(-0.479349583074855,1.,-1.96294933055943));
#29680=CARTESIAN_POINT('Ctrl Pts',(-0.482901662120691,-1.,-1.96792703422362));
#29681=CARTESIAN_POINT('Ctrl Pts',(-0.482901662120691,1.,-1.96792703422362));
#29682=CARTESIAN_POINT('Ctrl Pts',(-0.486502692907659,-1.,-1.97289186263272));
#29683=CARTESIAN_POINT('Ctrl Pts',(-0.486502692907659,1.,-1.97289186263272));
#29684=CARTESIAN_POINT('Ctrl Pts',(-0.490150627860952,-1.,-1.97783973019229));
#29685=CARTESIAN_POINT('Ctrl Pts',(-0.490150627860952,1.,-1.97783973019229));
#29686=CARTESIAN_POINT('Ctrl Pts',(-0.493843476541495,-1.,-1.98276658761821));
#29687=CARTESIAN_POINT('Ctrl Pts',(-0.493843476541495,1.,-1.98276658761821));
#29688=CARTESIAN_POINT('Ctrl Pts',(-0.497579909545574,-1.,-1.98767044752932));
#29689=CARTESIAN_POINT('Ctrl Pts',(-0.497579909545574,1.,-1.98767044752932));
#29690=CARTESIAN_POINT('Ctrl Pts',(-0.501359287727146,-1.,-1.99255149126155));
#29691=CARTESIAN_POINT('Ctrl Pts',(-0.501359287727146,1.,-1.99255149126155));
#29692=CARTESIAN_POINT('Ctrl Pts',(-0.505181361323026,-1.,-1.99741107463572));
#29693=CARTESIAN_POINT('Ctrl Pts',(-0.505181361323026,1.,-1.99741107463572));
#29694=CARTESIAN_POINT('Ctrl Pts',(-0.509046069886157,-1.,-2.00225107134734));
#29695=CARTESIAN_POINT('Ctrl Pts',(-0.509046069886157,1.,-2.00225107134734));
#29696=CARTESIAN_POINT('Ctrl Pts',(-0.512953306961792,-1.,-2.00707309946949));
#29697=CARTESIAN_POINT('Ctrl Pts',(-0.512953306961792,1.,-2.00707309946949));
#29698=CARTESIAN_POINT('Ctrl Pts',(-0.516902681728687,-1.,-2.01187773939242));
#29699=CARTESIAN_POINT('Ctrl Pts',(-0.516902681728687,1.,-2.01187773939242));
#29700=CARTESIAN_POINT('Ctrl Pts',(-0.52089359039937,-1.,-2.01666477917286));
#29701=CARTESIAN_POINT('Ctrl Pts',(-0.52089359039937,1.,-2.01666477917286));
#29702=CARTESIAN_POINT('Ctrl Pts',(-0.524925318333476,-1.,-2.02143356304698));
#29703=CARTESIAN_POINT('Ctrl Pts',(-0.524925318333476,1.,-2.02143356304698));
#29704=CARTESIAN_POINT('Ctrl Pts',(-0.528997127241914,-1.,-2.0261832908329));
#29705=CARTESIAN_POINT('Ctrl Pts',(-0.528997127241914,1.,-2.0261832908329));
#29706=CARTESIAN_POINT('Ctrl Pts',(-0.533108355132977,-1.,-2.03091336214426));
#29707=CARTESIAN_POINT('Ctrl Pts',(-0.533108355132977,1.,-2.03091336214426));
#29708=CARTESIAN_POINT('Ctrl Pts',(-0.537258489833262,-1.,-2.03562362954037));
#29709=CARTESIAN_POINT('Ctrl Pts',(-0.537258489833262,1.,-2.03562362954037));
#29710=CARTESIAN_POINT('Ctrl Pts',(-0.541447120615659,-1.,-2.04031422690527));
#29711=CARTESIAN_POINT('Ctrl Pts',(-0.541447120615659,1.,-2.04031422690527));
#29712=CARTESIAN_POINT('Ctrl Pts',(-0.54567390381743,-1.,-2.04498544714588));
#29713=CARTESIAN_POINT('Ctrl Pts',(-0.54567390381743,1.,-2.04498544714588));
#29714=CARTESIAN_POINT('Ctrl Pts',(-0.549938525150295,-1.,-2.04963761077958));
#29715=CARTESIAN_POINT('Ctrl Pts',(-0.549938525150295,1.,-2.04963761077958));
#29716=CARTESIAN_POINT('Ctrl Pts',(-0.554240657463906,-1.,-2.05427091604413));
#29717=CARTESIAN_POINT('Ctrl Pts',(-0.554240657463906,1.,-2.05427091604413));
#29718=CARTESIAN_POINT('Ctrl Pts',(-0.558579940185151,-1.,-2.05888537756462));
#29719=CARTESIAN_POINT('Ctrl Pts',(-0.558579940185151,1.,-2.05888537756462));
#29720=CARTESIAN_POINT('Ctrl Pts',(-0.562955993082261,-1.,-2.06348090160589));
#29721=CARTESIAN_POINT('Ctrl Pts',(-0.562955993082261,1.,-2.06348090160589));
#29722=CARTESIAN_POINT('Ctrl Pts',(-0.567368421181087,-1.,-2.06805732997334));
#29723=CARTESIAN_POINT('Ctrl Pts',(-0.567368421181087,1.,-2.06805732997334));
#29724=CARTESIAN_POINT('Ctrl Pts',(-0.571816823242603,-1.,-2.07261449292824));
#29725=CARTESIAN_POINT('Ctrl Pts',(-0.571816823242603,1.,-2.07261449292824));
#29726=CARTESIAN_POINT('Ctrl Pts',(-0.576300797416844,-1.,-2.07715226767559));
#29727=CARTESIAN_POINT('Ctrl Pts',(-0.576300797416844,1.,-2.07715226767559));
#29728=CARTESIAN_POINT('Ctrl Pts',(-0.580819952108063,-1.,-2.08167059018418));
#29729=CARTESIAN_POINT('Ctrl Pts',(-0.580819952108063,1.,-2.08167059018418));
#29730=CARTESIAN_POINT('Ctrl Pts',(-0.585373918991617,-1.,-2.08616943727951));
#29731=CARTESIAN_POINT('Ctrl Pts',(-0.585373918991617,1.,-2.08616943727951));
#29732=CARTESIAN_POINT('Ctrl Pts',(-0.589962365403406,-1.,-2.09064881812129));
#29733=CARTESIAN_POINT('Ctrl Pts',(-0.589962365403406,1.,-2.09064881812129));
#29734=CARTESIAN_POINT('Ctrl Pts',(-0.594585006052162,-1.,-2.0951087622027));
#29735=CARTESIAN_POINT('Ctrl Pts',(-0.594585006052162,1.,-2.0951087622027));
#29736=CARTESIAN_POINT('Ctrl Pts',(-0.599241616420533,-1.,-2.0995493086477));
#29737=CARTESIAN_POINT('Ctrl Pts',(-0.599241616420533,1.,-2.0995493086477));
#29738=CARTESIAN_POINT('Ctrl Pts',(-0.60393203073603,-1.,-2.10397049886949));
#29739=CARTESIAN_POINT('Ctrl Pts',(-0.60393203073603,1.,-2.10397049886949));
#29740=CARTESIAN_POINT('Ctrl Pts',(-0.607711315454876,-1.,-2.1074919961518));
#29741=CARTESIAN_POINT('Ctrl Pts',(-0.607711315454876,1.,-2.1074919961518));
#29742=CARTESIAN_POINT('Ctrl Pts',(-0.610560911689899,-1.,-2.11012443807238));
#29743=CARTESIAN_POINT('Ctrl Pts',(-0.610560911689899,1.,-2.11012443807238));
#29744=CARTESIAN_POINT('Ctrl Pts',(-0.6124673655618,-1.,-2.11187554259986));
#29745=CARTESIAN_POINT('Ctrl Pts',(-0.6124673655618,1.,-2.11187554259986));
#29746=CARTESIAN_POINT('Ctrl Pts',(-0.61342227326009,-1.,-2.11275013067528));
#29747=CARTESIAN_POINT('Ctrl Pts',(-0.61342227326009,1.,-2.11275013067528));
#29748=CARTESIAN_POINT('',(-0.383122945602004,1.,-1.7075470150345));
#29749=CARTESIAN_POINT('Ctrl Pts',(-0.383122945602004,1.,-1.7075470150345));
#29750=CARTESIAN_POINT('Ctrl Pts',(-0.384119047315542,1.,-1.71231062891958));
#29751=CARTESIAN_POINT('Ctrl Pts',(-0.38607079032701,1.,-1.72162022246158));
#29752=CARTESIAN_POINT('Ctrl Pts',(-0.388877023509191,1.,-1.7349317097561));
#29753=CARTESIAN_POINT('Ctrl Pts',(-0.392375812294307,1.,-1.75137405313962));
#29754=CARTESIAN_POINT('Ctrl Pts',(-0.39634619612042,1.,-1.7697556004756));
#29755=CARTESIAN_POINT('Ctrl Pts',(-0.39991940378308,1.,-1.78598826347533));
#29756=CARTESIAN_POINT('Ctrl Pts',(-0.403107976170441,1.,-1.80012077176221));
#29757=CARTESIAN_POINT('Ctrl Pts',(-0.405933518411838,1.,-1.81223801813988));
#29758=CARTESIAN_POINT('Ctrl Pts',(-0.408428948108533,1.,-1.8224702267854));
#29759=CARTESIAN_POINT('Ctrl Pts',(-0.410641256301675,1.,-1.83100408895216));
#29760=CARTESIAN_POINT('Ctrl Pts',(-0.412633125322162,1.,-1.83808953475839));
#29761=CARTESIAN_POINT('Ctrl Pts',(-0.41448743825434,1.,-1.8440575707371));
#29762=CARTESIAN_POINT('Ctrl Pts',(-0.416300022038864,1.,-1.84929312929882));
#29763=CARTESIAN_POINT('Ctrl Pts',(-0.418164129143534,1.,-1.85417632856234));
#29764=CARTESIAN_POINT('Ctrl Pts',(-0.420157287975619,1.,-1.85903281096686));
#29765=CARTESIAN_POINT('Ctrl Pts',(-0.422327307418275,1.,-1.86408083334028));
#29766=CARTESIAN_POINT('Ctrl Pts',(-0.424678177291359,1.,-1.86937803944323));
#29767=CARTESIAN_POINT('Ctrl Pts',(-0.427183828519102,1.,-1.87486989291484));
#29768=CARTESIAN_POINT('Ctrl Pts',(-0.429803062482344,1.,-1.88044229001832));
#29769=CARTESIAN_POINT('Ctrl Pts',(-0.432493038548748,1.,-1.88596913666793));
#29770=CARTESIAN_POINT('Ctrl Pts',(-0.435225660963383,1.,-1.89136993975504));
#29771=CARTESIAN_POINT('Ctrl Pts',(-0.437995003948244,1.,-1.89663648956466));
#29772=CARTESIAN_POINT('Ctrl Pts',(-0.440807833704038,1.,-1.90180124389086));
#29773=CARTESIAN_POINT('Ctrl Pts',(-0.443677556849151,1.,-1.90691756144898));
#29774=CARTESIAN_POINT('Ctrl Pts',(-0.446617343485711,1.,-1.9120369998112));
#29775=CARTESIAN_POINT('Ctrl Pts',(-0.449632260106662,1.,-1.91718342555755));
#29776=CARTESIAN_POINT('Ctrl Pts',(-0.452719478359432,1.,-1.92235380648502));
#29777=CARTESIAN_POINT('Ctrl Pts',(-0.455872005174371,1.,-1.92753067150476));
#29778=CARTESIAN_POINT('Ctrl Pts',(-0.459081234547926,1.,-1.93269066517934));
#29779=CARTESIAN_POINT('Ctrl Pts',(-0.462340031009056,1.,-1.93781486640821));
#29780=CARTESIAN_POINT('Ctrl Pts',(-0.46564546202603,1.,-1.9428979419619));
#29781=CARTESIAN_POINT('Ctrl Pts',(-0.468997482913135,1.,-1.94794381136514));
#29782=CARTESIAN_POINT('Ctrl Pts',(-0.472397672264072,1.,-1.95296148278133));
#29783=CARTESIAN_POINT('Ctrl Pts',(-0.475848034683176,1.,-1.95796111148177));
#29784=CARTESIAN_POINT('Ctrl Pts',(-0.479349583074855,1.,-1.96294933055943));
#29785=CARTESIAN_POINT('Ctrl Pts',(-0.482901662120691,1.,-1.96792703422362));
#29786=CARTESIAN_POINT('Ctrl Pts',(-0.486502692907659,1.,-1.97289186263272));
#29787=CARTESIAN_POINT('Ctrl Pts',(-0.490150627860952,1.,-1.97783973019229));
#29788=CARTESIAN_POINT('Ctrl Pts',(-0.493843476541495,1.,-1.98276658761821));
#29789=CARTESIAN_POINT('Ctrl Pts',(-0.497579909545574,1.,-1.98767044752932));
#29790=CARTESIAN_POINT('Ctrl Pts',(-0.501359287727146,1.,-1.99255149126155));
#29791=CARTESIAN_POINT('Ctrl Pts',(-0.505181361323026,1.,-1.99741107463572));
#29792=CARTESIAN_POINT('Ctrl Pts',(-0.509046069886157,1.,-2.00225107134734));
#29793=CARTESIAN_POINT('Ctrl Pts',(-0.512953306961792,1.,-2.00707309946949));
#29794=CARTESIAN_POINT('Ctrl Pts',(-0.516902681728687,1.,-2.01187773939242));
#29795=CARTESIAN_POINT('Ctrl Pts',(-0.52089359039937,1.,-2.01666477917286));
#29796=CARTESIAN_POINT('Ctrl Pts',(-0.524925318333476,1.,-2.02143356304698));
#29797=CARTESIAN_POINT('Ctrl Pts',(-0.528997127241914,1.,-2.0261832908329));
#29798=CARTESIAN_POINT('Ctrl Pts',(-0.533108355132977,1.,-2.03091336214426));
#29799=CARTESIAN_POINT('Ctrl Pts',(-0.537258489833262,1.,-2.03562362954037));
#29800=CARTESIAN_POINT('Ctrl Pts',(-0.541447120615659,1.,-2.04031422690527));
#29801=CARTESIAN_POINT('Ctrl Pts',(-0.54567390381743,1.,-2.04498544714588));
#29802=CARTESIAN_POINT('Ctrl Pts',(-0.549938525150295,1.,-2.04963761077958));
#29803=CARTESIAN_POINT('Ctrl Pts',(-0.554240657463906,1.,-2.05427091604413));
#29804=CARTESIAN_POINT('Ctrl Pts',(-0.558579940185151,1.,-2.05888537756462));
#29805=CARTESIAN_POINT('Ctrl Pts',(-0.562955993082261,1.,-2.06348090160589));
#29806=CARTESIAN_POINT('Ctrl Pts',(-0.567368421181087,1.,-2.06805732997334));
#29807=CARTESIAN_POINT('Ctrl Pts',(-0.571816823242603,1.,-2.07261449292824));
#29808=CARTESIAN_POINT('Ctrl Pts',(-0.576300797416844,1.,-2.07715226767559));
#29809=CARTESIAN_POINT('Ctrl Pts',(-0.580819952108063,1.,-2.08167059018418));
#29810=CARTESIAN_POINT('Ctrl Pts',(-0.585373918991617,1.,-2.08616943727951));
#29811=CARTESIAN_POINT('Ctrl Pts',(-0.589962365403406,1.,-2.09064881812129));
#29812=CARTESIAN_POINT('Ctrl Pts',(-0.594585006052162,1.,-2.0951087622027));
#29813=CARTESIAN_POINT('Ctrl Pts',(-0.599241616420533,1.,-2.0995493086477));
#29814=CARTESIAN_POINT('Ctrl Pts',(-0.60393203073603,1.,-2.10397049886949));
#29815=CARTESIAN_POINT('Ctrl Pts',(-0.607711315454876,1.,-2.1074919961518));
#29816=CARTESIAN_POINT('Ctrl Pts',(-0.610560911689899,1.,-2.11012443807238));
#29817=CARTESIAN_POINT('Ctrl Pts',(-0.6124673655618,1.,-2.11187554259986));
#29818=CARTESIAN_POINT('Ctrl Pts',(-0.61342227326009,1.,-2.11275013067528));
#29819=CARTESIAN_POINT('',(-0.383122945602003,0.,-1.7075470150345));
#29820=CARTESIAN_POINT('Origin',(0.,0.,0.));
#29821=CARTESIAN_POINT('',(-0.163289472382896,1.,-1.74236521665491));
#29822=CARTESIAN_POINT('Origin',(0.,1.,0.));
#29823=CARTESIAN_POINT('',(-0.163289472382896,0.,-1.74236521665491));
#29824=CARTESIAN_POINT('Ctrl Pts',(-0.0694764450219581,-1.,-2.19890268624765));
#29825=CARTESIAN_POINT('Ctrl Pts',(-0.0694764450219581,1.,-2.19890268624765));
#29826=CARTESIAN_POINT('Ctrl Pts',(-0.070114353632549,-1.,-2.19777582085423));
#29827=CARTESIAN_POINT('Ctrl Pts',(-0.070114353632549,1.,-2.19777582085423));
#29828=CARTESIAN_POINT('Ctrl Pts',(-0.0713863779526154,-1.,-2.19552129484002));
#29829=CARTESIAN_POINT('Ctrl Pts',(-0.0713863779526154,1.,-2.19552129484002));
#29830=CARTESIAN_POINT('Ctrl Pts',(-0.0732830357306725,-1.,-2.19213712013662));
#29831=CARTESIAN_POINT('Ctrl Pts',(-0.0732830357306725,1.,-2.19213712013662));
#29832=CARTESIAN_POINT('Ctrl Pts',(-0.0757891465836148,-1.,-2.1876201139953));
#29833=CARTESIAN_POINT('Ctrl Pts',(-0.0757891465836148,1.,-2.1876201139953));
#29834=CARTESIAN_POINT('Ctrl Pts',(-0.0788837727685243,-1.,-2.18196589448887));
#29835=CARTESIAN_POINT('Ctrl Pts',(-0.0788837727685243,1.,-2.18196589448887));
#29836=CARTESIAN_POINT('Ctrl Pts',(-0.0819402680872765,-1.,-2.176303712113));
#29837=CARTESIAN_POINT('Ctrl Pts',(-0.0819402680872765,1.,-2.176303712113));
#29838=CARTESIAN_POINT('Ctrl Pts',(-0.0849584620835372,-1.,-2.17063357870952));
#29839=CARTESIAN_POINT('Ctrl Pts',(-0.0849584620835372,1.,-2.17063357870952));
#29840=CARTESIAN_POINT('Ctrl Pts',(-0.0879381291386923,-1.,-2.16495552645014));
#29841=CARTESIAN_POINT('Ctrl Pts',(-0.0879381291386923,1.,-2.16495552645014));
#29842=CARTESIAN_POINT('Ctrl Pts',(-0.0908789888107265,-1.,-2.15926961544516));
#29843=CARTESIAN_POINT('Ctrl Pts',(-0.0908789888107265,1.,-2.15926961544516));
#29844=CARTESIAN_POINT('Ctrl Pts',(-0.0937807218867643,-1.,-2.1535759397817));
#29845=CARTESIAN_POINT('Ctrl Pts',(-0.0937807218867643,1.,-2.1535759397817));
#29846=CARTESIAN_POINT('Ctrl Pts',(-0.0966429852305459,-1.,-2.14787463531795));
#29847=CARTESIAN_POINT('Ctrl Pts',(-0.0966429852305459,1.,-2.14787463531795));
#29848=CARTESIAN_POINT('Ctrl Pts',(-0.0994654261990915,-1.,-2.14216588396025));
#29849=CARTESIAN_POINT('Ctrl Pts',(-0.0994654261990915,1.,-2.14216588396025));
#29850=CARTESIAN_POINT('Ctrl Pts',(-0.1022477005561,-1.,-2.13644992667165));
#29851=CARTESIAN_POINT('Ctrl Pts',(-0.1022477005561,1.,-2.13644992667165));
#29852=CARTESIAN_POINT('Ctrl Pts',(-0.104989479152739,-1.,-2.13072704887293));
#29853=CARTESIAN_POINT('Ctrl Pts',(-0.104989479152739,1.,-2.13072704887293));
#29854=CARTESIAN_POINT('Ctrl Pts',(-0.10769043523109,-1.,-2.12499752307));
#29855=CARTESIAN_POINT('Ctrl Pts',(-0.10769043523109,1.,-2.12499752307));
#29856=CARTESIAN_POINT('Ctrl Pts',(-0.110350236135025,-1.,-2.11926155590865));
#29857=CARTESIAN_POINT('Ctrl Pts',(-0.110350236135025,1.,-2.11926155590865));
#29858=CARTESIAN_POINT('Ctrl Pts',(-0.112968534419737,-1.,-2.11351924490306));
#29859=CARTESIAN_POINT('Ctrl Pts',(-0.112968534419737,1.,-2.11351924490306));
#29860=CARTESIAN_POINT('Ctrl Pts',(-0.115544957687926,-1.,-2.10777050261309));
#29861=CARTESIAN_POINT('Ctrl Pts',(-0.115544957687926,1.,-2.10777050261309));
#29862=CARTESIAN_POINT('Ctrl Pts',(-0.118079107988355,-1.,-2.102015121329));
#29863=CARTESIAN_POINT('Ctrl Pts',(-0.118079107988355,1.,-2.102015121329));
#29864=CARTESIAN_POINT('Ctrl Pts',(-0.120570567965122,-1.,-2.0962529286773));
#29865=CARTESIAN_POINT('Ctrl Pts',(-0.120570567965122,1.,-2.0962529286773));
#29866=CARTESIAN_POINT('Ctrl Pts',(-0.123018905621083,-1.,-2.09048392424825));
#29867=CARTESIAN_POINT('Ctrl Pts',(-0.123018905621083,1.,-2.09048392424825));
#29868=CARTESIAN_POINT('Ctrl Pts',(-0.125423679412061,-1.,-2.08470840653643));
#29869=CARTESIAN_POINT('Ctrl Pts',(-0.125423679412061,1.,-2.08470840653643));
#29870=CARTESIAN_POINT('Ctrl Pts',(-0.12778444527612,-1.,-2.07892715110987));
#29871=CARTESIAN_POINT('Ctrl Pts',(-0.12778444527612,1.,-2.07892715110987));
#29872=CARTESIAN_POINT('Ctrl Pts',(-0.130100748328403,-1.,-2.07314114713063));
#29873=CARTESIAN_POINT('Ctrl Pts',(-0.130100748328403,1.,-2.07314114713063));
#29874=CARTESIAN_POINT('Ctrl Pts',(-0.13237211154771,-1.,-2.06735123910326));
#29875=CARTESIAN_POINT('Ctrl Pts',(-0.13237211154771,1.,-2.06735123910326));
#29876=CARTESIAN_POINT('Ctrl Pts',(-0.134598026192106,-1.,-2.06155781517842));
#29877=CARTESIAN_POINT('Ctrl Pts',(-0.134598026192106,1.,-2.06155781517842));
#29878=CARTESIAN_POINT('Ctrl Pts',(-0.136777941218044,-1.,-2.05576044414264));
#29879=CARTESIAN_POINT('Ctrl Pts',(-0.136777941218044,1.,-2.05576044414264));
#29880=CARTESIAN_POINT('Ctrl Pts',(-0.138911255368966,-1.,-2.04995762001328));
#29881=CARTESIAN_POINT('Ctrl Pts',(-0.138911255368966,1.,-2.04995762001328));
#29882=CARTESIAN_POINT('Ctrl Pts',(-0.140997332152546,-1.,-2.04414757947916));
#29883=CARTESIAN_POINT('Ctrl Pts',(-0.140997332152546,1.,-2.04414757947916));
#29884=CARTESIAN_POINT('Ctrl Pts',(-0.143035515058209,-1.,-2.03832911025912));
#29885=CARTESIAN_POINT('Ctrl Pts',(-0.143035515058209,1.,-2.03832911025912));
#29886=CARTESIAN_POINT('Ctrl Pts',(-0.145025140186057,-1.,-2.03250223739942));
#29887=CARTESIAN_POINT('Ctrl Pts',(-0.145025140186057,1.,-2.03250223739942));
#29888=CARTESIAN_POINT('Ctrl Pts',(-0.146965557332583,-1.,-2.02666926182017));
#29889=CARTESIAN_POINT('Ctrl Pts',(-0.146965557332583,1.,-2.02666926182017));
#29890=CARTESIAN_POINT('Ctrl Pts',(-0.148856124775337,-1.,-2.02083464969894));
#29891=CARTESIAN_POINT('Ctrl Pts',(-0.148856124775337,1.,-2.02083464969894));
#29892=CARTESIAN_POINT('Ctrl Pts',(-0.150696157673078,-1.,-2.01500291940238));
#29893=CARTESIAN_POINT('Ctrl Pts',(-0.150696157673078,1.,-2.01500291940238));
#29894=CARTESIAN_POINT('Ctrl Pts',(-0.15248488362145,-1.,-2.00917680318424));
#29895=CARTESIAN_POINT('Ctrl Pts',(-0.15248488362145,1.,-2.00917680318424));
#29896=CARTESIAN_POINT('Ctrl Pts',(-0.154221403049722,-1.,-2.00335565310543));
#29897=CARTESIAN_POINT('Ctrl Pts',(-0.154221403049722,1.,-2.00335565310543));
#29898=CARTESIAN_POINT('Ctrl Pts',(-0.155904629548783,-1.,-1.99753284771497));
#29899=CARTESIAN_POINT('Ctrl Pts',(-0.155904629548783,1.,-1.99753284771497));
#29900=CARTESIAN_POINT('Ctrl Pts',(-0.157533331459227,-1.,-1.99169810931908));
#29901=CARTESIAN_POINT('Ctrl Pts',(-0.157533331459227,1.,-1.99169810931908));
#29902=CARTESIAN_POINT('Ctrl Pts',(-0.159106226437299,-1.,-1.98584238283292));
#29903=CARTESIAN_POINT('Ctrl Pts',(-0.159106226437299,1.,-1.98584238283292));
#29904=CARTESIAN_POINT('Ctrl Pts',(-0.160622060784611,-1.,-1.97996195437559));
#29905=CARTESIAN_POINT('Ctrl Pts',(-0.160622060784611,1.,-1.97996195437559));
#29906=CARTESIAN_POINT('Ctrl Pts',(-0.162079693556289,-1.,-1.97406280235188));
#29907=CARTESIAN_POINT('Ctrl Pts',(-0.162079693556289,1.,-1.97406280235188));
#29908=CARTESIAN_POINT('Ctrl Pts',(-0.163478185457734,-1.,-1.96816512677967));
#29909=CARTESIAN_POINT('Ctrl Pts',(-0.163478185457734,1.,-1.96816512677967));
#29910=CARTESIAN_POINT('Ctrl Pts',(-0.164816568920269,-1.,-1.96229379940136));
#29911=CARTESIAN_POINT('Ctrl Pts',(-0.164816568920269,1.,-1.96229379940136));
#29912=CARTESIAN_POINT('Ctrl Pts',(-0.166093592002812,-1.,-1.9564675971873));
#29913=CARTESIAN_POINT('Ctrl Pts',(-0.166093592002812,1.,-1.9564675971873));
#29914=CARTESIAN_POINT('Ctrl Pts',(-0.167307501784475,-1.,-1.95069027794294));
#29915=CARTESIAN_POINT('Ctrl Pts',(-0.167307501784475,1.,-1.95069027794294));
#29916=CARTESIAN_POINT('Ctrl Pts',(-0.168455741607556,-1.,-1.94493757756931));
#29917=CARTESIAN_POINT('Ctrl Pts',(-0.168455741607556,1.,-1.94493757756931));
#29918=CARTESIAN_POINT('Ctrl Pts',(-0.169534904817491,-1.,-1.93915639211581));
#29919=CARTESIAN_POINT('Ctrl Pts',(-0.169534904817491,1.,-1.93915639211581));
#29920=CARTESIAN_POINT('Ctrl Pts',(-0.170541253116202,-1.,-1.93329183155539));
#29921=CARTESIAN_POINT('Ctrl Pts',(-0.170541253116202,1.,-1.93329183155539));
#29922=CARTESIAN_POINT('Ctrl Pts',(-0.171471191532988,-1.,-1.92731093582036));
#29923=CARTESIAN_POINT('Ctrl Pts',(-0.171471191532988,1.,-1.92731093582036));
#29924=CARTESIAN_POINT('Ctrl Pts',(-0.172321621259514,-1.,-1.9212233439798));
#29925=CARTESIAN_POINT('Ctrl Pts',(-0.172321621259514,1.,-1.9212233439798));
#29926=CARTESIAN_POINT('Ctrl Pts',(-0.173090695383496,-1.,-1.91511429159527));
#29927=CARTESIAN_POINT('Ctrl Pts',(-0.173090695383496,1.,-1.91511429159527));
#29928=CARTESIAN_POINT('Ctrl Pts',(-0.173776635257817,-1.,-1.90911693975267));
#29929=CARTESIAN_POINT('Ctrl Pts',(-0.173776635257817,1.,-1.90911693975267));
#29930=CARTESIAN_POINT('Ctrl Pts',(-0.174375518661085,-1.,-1.90335253862834));
#29931=CARTESIAN_POINT('Ctrl Pts',(-0.174375518661085,1.,-1.90335253862834));
#29932=CARTESIAN_POINT('Ctrl Pts',(-0.174879405091263,-1.,-1.89788101117132));
#29933=CARTESIAN_POINT('Ctrl Pts',(-0.174879405091263,1.,-1.89788101117132));
#29934=CARTESIAN_POINT('Ctrl Pts',(-0.175274276190844,-1.,-1.892646301985));
#29935=CARTESIAN_POINT('Ctrl Pts',(-0.175274276190844,1.,-1.892646301985));
#29936=CARTESIAN_POINT('Ctrl Pts',(-0.175538155840648,-1.,-1.88742606273259));
#29937=CARTESIAN_POINT('Ctrl Pts',(-0.175538155840648,1.,-1.88742606273259));
#29938=CARTESIAN_POINT('Ctrl Pts',(-0.175644148889699,-1.,-1.88188663145367));
#29939=CARTESIAN_POINT('Ctrl Pts',(-0.175644148889699,1.,-1.88188663145367));
#29940=CARTESIAN_POINT('Ctrl Pts',(-0.175563480746485,-1.,-1.87563767773588));
#29941=CARTESIAN_POINT('Ctrl Pts',(-0.175563480746485,1.,-1.87563767773588));
#29942=CARTESIAN_POINT('Ctrl Pts',(-0.175268337590758,-1.,-1.86828349694799));
#29943=CARTESIAN_POINT('Ctrl Pts',(-0.175268337590758,1.,-1.86828349694799));
#29944=CARTESIAN_POINT('Ctrl Pts',(-0.17473525927603,-1.,-1.85948367088837));
#29945=CARTESIAN_POINT('Ctrl Pts',(-0.17473525927603,1.,-1.85948367088837));
#29946=CARTESIAN_POINT('Ctrl Pts',(-0.173946627587731,-1.,-1.8489811319852));
#29947=CARTESIAN_POINT('Ctrl Pts',(-0.173946627587731,1.,-1.8489811319852));
#29948=CARTESIAN_POINT('Ctrl Pts',(-0.1728894428919,-1.,-1.83658380527692));
#29949=CARTESIAN_POINT('Ctrl Pts',(-0.1728894428919,1.,-1.83658380527692));
#29950=CARTESIAN_POINT('Ctrl Pts',(-0.171554770204119,-1.,-1.82215766811545));
#29951=CARTESIAN_POINT('Ctrl Pts',(-0.171554770204119,1.,-1.82215766811545));
#29952=CARTESIAN_POINT('Ctrl Pts',(-0.169936923904608,-1.,-1.80561530629706));
#29953=CARTESIAN_POINT('Ctrl Pts',(-0.169936923904608,1.,-1.80561530629706));
#29954=CARTESIAN_POINT('Ctrl Pts',(-0.168032772805197,-1.,-1.7869064998507));
#29955=CARTESIAN_POINT('Ctrl Pts',(-0.168032772805197,1.,-1.7869064998507));
#29956=CARTESIAN_POINT('Ctrl Pts',(-0.1662793551464,-1.,-1.77018771684844));
#29957=CARTESIAN_POINT('Ctrl Pts',(-0.1662793551464,1.,-1.77018771684844));
#29958=CARTESIAN_POINT('Ctrl Pts',(-0.164834765707158,-1.,-1.75666056638427));
#29959=CARTESIAN_POINT('Ctrl Pts',(-0.164834765707158,1.,-1.75666056638427));
#29960=CARTESIAN_POINT('Ctrl Pts',(-0.163814161002002,-1.,-1.7472034950333));
#29961=CARTESIAN_POINT('Ctrl Pts',(-0.163814161002002,1.,-1.7472034950333));
#29962=CARTESIAN_POINT('Ctrl Pts',(-0.163289472382896,-1.,-1.74236521665491));
#29963=CARTESIAN_POINT('Ctrl Pts',(-0.163289472382896,1.,-1.74236521665491));
#29964=CARTESIAN_POINT('',(-0.0694764450219581,1.,-2.19890268624765));
#29965=CARTESIAN_POINT('Ctrl Pts',(-0.0694764450219581,1.,-2.19890268624765));
#29966=CARTESIAN_POINT('Ctrl Pts',(-0.070114353632549,1.,-2.19777582085423));
#29967=CARTESIAN_POINT('Ctrl Pts',(-0.0713863779526154,1.,-2.19552129484002));
#29968=CARTESIAN_POINT('Ctrl Pts',(-0.0732830357306725,1.,-2.19213712013662));
#29969=CARTESIAN_POINT('Ctrl Pts',(-0.0757891465836148,1.,-2.1876201139953));
#29970=CARTESIAN_POINT('Ctrl Pts',(-0.0788837727685243,1.,-2.18196589448887));
#29971=CARTESIAN_POINT('Ctrl Pts',(-0.0819402680872765,1.,-2.176303712113));
#29972=CARTESIAN_POINT('Ctrl Pts',(-0.0849584620835372,1.,-2.17063357870952));
#29973=CARTESIAN_POINT('Ctrl Pts',(-0.0879381291386923,1.,-2.16495552645014));
#29974=CARTESIAN_POINT('Ctrl Pts',(-0.0908789888107265,1.,-2.15926961544516));
#29975=CARTESIAN_POINT('Ctrl Pts',(-0.0937807218867643,1.,-2.1535759397817));
#29976=CARTESIAN_POINT('Ctrl Pts',(-0.0966429852305459,1.,-2.14787463531795));
#29977=CARTESIAN_POINT('Ctrl Pts',(-0.0994654261990915,1.,-2.14216588396025));
#29978=CARTESIAN_POINT('Ctrl Pts',(-0.1022477005561,1.,-2.13644992667165));
#29979=CARTESIAN_POINT('Ctrl Pts',(-0.104989479152739,1.,-2.13072704887293));
#29980=CARTESIAN_POINT('Ctrl Pts',(-0.10769043523109,1.,-2.12499752307));
#29981=CARTESIAN_POINT('Ctrl Pts',(-0.110350236135025,1.,-2.11926155590865));
#29982=CARTESIAN_POINT('Ctrl Pts',(-0.112968534419737,1.,-2.11351924490306));
#29983=CARTESIAN_POINT('Ctrl Pts',(-0.115544957687926,1.,-2.10777050261309));
#29984=CARTESIAN_POINT('Ctrl Pts',(-0.118079107988355,1.,-2.102015121329));
#29985=CARTESIAN_POINT('Ctrl Pts',(-0.120570567965122,1.,-2.0962529286773));
#29986=CARTESIAN_POINT('Ctrl Pts',(-0.123018905621083,1.,-2.09048392424825));
#29987=CARTESIAN_POINT('Ctrl Pts',(-0.125423679412061,1.,-2.08470840653643));
#29988=CARTESIAN_POINT('Ctrl Pts',(-0.12778444527612,1.,-2.07892715110987));
#29989=CARTESIAN_POINT('Ctrl Pts',(-0.130100748328403,1.,-2.07314114713063));
#29990=CARTESIAN_POINT('Ctrl Pts',(-0.13237211154771,1.,-2.06735123910326));
#29991=CARTESIAN_POINT('Ctrl Pts',(-0.134598026192106,1.,-2.06155781517842));
#29992=CARTESIAN_POINT('Ctrl Pts',(-0.136777941218044,1.,-2.05576044414264));
#29993=CARTESIAN_POINT('Ctrl Pts',(-0.138911255368966,1.,-2.04995762001328));
#29994=CARTESIAN_POINT('Ctrl Pts',(-0.140997332152546,1.,-2.04414757947916));
#29995=CARTESIAN_POINT('Ctrl Pts',(-0.143035515058209,1.,-2.03832911025912));
#29996=CARTESIAN_POINT('Ctrl Pts',(-0.145025140186057,1.,-2.03250223739942));
#29997=CARTESIAN_POINT('Ctrl Pts',(-0.146965557332583,1.,-2.02666926182017));
#29998=CARTESIAN_POINT('Ctrl Pts',(-0.148856124775337,1.,-2.02083464969894));
#29999=CARTESIAN_POINT('Ctrl Pts',(-0.150696157673078,1.,-2.01500291940238));
#30000=CARTESIAN_POINT('Ctrl Pts',(-0.15248488362145,1.,-2.00917680318424));
#30001=CARTESIAN_POINT('Ctrl Pts',(-0.154221403049722,1.,-2.00335565310543));
#30002=CARTESIAN_POINT('Ctrl Pts',(-0.155904629548783,1.,-1.99753284771497));
#30003=CARTESIAN_POINT('Ctrl Pts',(-0.157533331459227,1.,-1.99169810931908));
#30004=CARTESIAN_POINT('Ctrl Pts',(-0.159106226437299,1.,-1.98584238283292));
#30005=CARTESIAN_POINT('Ctrl Pts',(-0.160622060784611,1.,-1.97996195437559));
#30006=CARTESIAN_POINT('Ctrl Pts',(-0.162079693556289,1.,-1.97406280235188));
#30007=CARTESIAN_POINT('Ctrl Pts',(-0.163478185457734,1.,-1.96816512677967));
#30008=CARTESIAN_POINT('Ctrl Pts',(-0.164816568920269,1.,-1.96229379940136));
#30009=CARTESIAN_POINT('Ctrl Pts',(-0.166093592002812,1.,-1.9564675971873));
#30010=CARTESIAN_POINT('Ctrl Pts',(-0.167307501784475,1.,-1.95069027794294));
#30011=CARTESIAN_POINT('Ctrl Pts',(-0.168455741607556,1.,-1.94493757756931));
#30012=CARTESIAN_POINT('Ctrl Pts',(-0.169534904817491,1.,-1.93915639211581));
#30013=CARTESIAN_POINT('Ctrl Pts',(-0.170541253116202,1.,-1.93329183155539));
#30014=CARTESIAN_POINT('Ctrl Pts',(-0.171471191532988,1.,-1.92731093582036));
#30015=CARTESIAN_POINT('Ctrl Pts',(-0.172321621259514,1.,-1.9212233439798));
#30016=CARTESIAN_POINT('Ctrl Pts',(-0.173090695383496,1.,-1.91511429159527));
#30017=CARTESIAN_POINT('Ctrl Pts',(-0.173776635257817,1.,-1.90911693975267));
#30018=CARTESIAN_POINT('Ctrl Pts',(-0.174375518661085,1.,-1.90335253862834));
#30019=CARTESIAN_POINT('Ctrl Pts',(-0.174879405091263,1.,-1.89788101117132));
#30020=CARTESIAN_POINT('Ctrl Pts',(-0.175274276190844,1.,-1.892646301985));
#30021=CARTESIAN_POINT('Ctrl Pts',(-0.175538155840648,1.,-1.88742606273259));
#30022=CARTESIAN_POINT('Ctrl Pts',(-0.175644148889699,1.,-1.88188663145367));
#30023=CARTESIAN_POINT('Ctrl Pts',(-0.175563480746485,1.,-1.87563767773588));
#30024=CARTESIAN_POINT('Ctrl Pts',(-0.175268337590758,1.,-1.86828349694799));
#30025=CARTESIAN_POINT('Ctrl Pts',(-0.17473525927603,1.,-1.85948367088837));
#30026=CARTESIAN_POINT('Ctrl Pts',(-0.173946627587731,1.,-1.8489811319852));
#30027=CARTESIAN_POINT('Ctrl Pts',(-0.1728894428919,1.,-1.83658380527692));
#30028=CARTESIAN_POINT('Ctrl Pts',(-0.171554770204119,1.,-1.82215766811545));
#30029=CARTESIAN_POINT('Ctrl Pts',(-0.169936923904608,1.,-1.80561530629706));
#30030=CARTESIAN_POINT('Ctrl Pts',(-0.168032772805197,1.,-1.7869064998507));
#30031=CARTESIAN_POINT('Ctrl Pts',(-0.1662793551464,1.,-1.77018771684844));
#30032=CARTESIAN_POINT('Ctrl Pts',(-0.164834765707158,1.,-1.75666056638427));
#30033=CARTESIAN_POINT('Ctrl Pts',(-0.163814161002002,1.,-1.7472034950333));
#30034=CARTESIAN_POINT('Ctrl Pts',(-0.163289472382896,1.,-1.74236521665491));
#30035=CARTESIAN_POINT('',(-0.0694764450219581,0.,-2.19890268624765));
#30036=CARTESIAN_POINT('Origin',(0.0694764450219584,0.,-2.19890268624765));
#30037=CARTESIAN_POINT('',(0.0694764450219584,1.,-2.19890268624765));
#30038=CARTESIAN_POINT('',(-0.0694764450219581,1.,-2.19890268624765));
#30039=CARTESIAN_POINT('',(0.0694764450219584,0.,-2.19890268624765));
#30040=CARTESIAN_POINT('Ctrl Pts',(0.163289472382896,-1.,-1.74236521665491));
#30041=CARTESIAN_POINT('Ctrl Pts',(0.163289472382896,1.,-1.74236521665491));
#30042=CARTESIAN_POINT('Ctrl Pts',(0.163814161002474,-1.,-1.74720349503904));
#30043=CARTESIAN_POINT('Ctrl Pts',(0.163814161002474,1.,-1.74720349503904));
#30044=CARTESIAN_POINT('Ctrl Pts',(0.164834765708484,-1.,-1.75666056640041));
#30045=CARTESIAN_POINT('Ctrl Pts',(0.164834765708484,1.,-1.75666056640041));
#30046=CARTESIAN_POINT('Ctrl Pts',(0.166279355148738,-1.,-1.77018771687692));
#30047=CARTESIAN_POINT('Ctrl Pts',(0.166279355148738,1.,-1.77018771687692));
#30048=CARTESIAN_POINT('Ctrl Pts',(0.16803277280837,-1.,-1.78690649988931));
#30049=CARTESIAN_POINT('Ctrl Pts',(0.16803277280837,1.,-1.78690649988931));
#30050=CARTESIAN_POINT('Ctrl Pts',(0.169936923908078,-1.,-1.80561530633924));
#30051=CARTESIAN_POINT('Ctrl Pts',(0.169936923908078,1.,-1.80561530633924));
#30052=CARTESIAN_POINT('Ctrl Pts',(0.171554770207306,-1.,-1.82215766815414));
#30053=CARTESIAN_POINT('Ctrl Pts',(0.171554770207306,1.,-1.82215766815414));
#30054=CARTESIAN_POINT('Ctrl Pts',(0.17288944289442,-1.,-1.83658380530747));
#30055=CARTESIAN_POINT('Ctrl Pts',(0.17288944289442,1.,-1.83658380530747));
#30056=CARTESIAN_POINT('Ctrl Pts',(0.173946627589401,-1.,-1.84898113200543));
#30057=CARTESIAN_POINT('Ctrl Pts',(0.173946627589401,1.,-1.84898113200543));
#30058=CARTESIAN_POINT('Ctrl Pts',(0.174735259276856,-1.,-1.85948367089838));
#30059=CARTESIAN_POINT('Ctrl Pts',(0.174735259276856,1.,-1.85948367089838));
#30060=CARTESIAN_POINT('Ctrl Pts',(0.175268337590901,-1.,-1.86828349694972));
#30061=CARTESIAN_POINT('Ctrl Pts',(0.175268337590901,1.,-1.86828349694972));
#30062=CARTESIAN_POINT('Ctrl Pts',(0.175563480746205,-1.,-1.87563767773249));
#30063=CARTESIAN_POINT('Ctrl Pts',(0.175563480746205,1.,-1.87563767773249));
#30064=CARTESIAN_POINT('Ctrl Pts',(0.175644148889271,-1.,-1.88188663144846));
#30065=CARTESIAN_POINT('Ctrl Pts',(0.175644148889271,1.,-1.88188663144846));
#30066=CARTESIAN_POINT('Ctrl Pts',(0.175538155840286,-1.,-1.88742606272818));
#30067=CARTESIAN_POINT('Ctrl Pts',(0.175538155840286,1.,-1.88742606272818));
#30068=CARTESIAN_POINT('Ctrl Pts',(0.175274276190664,-1.,-1.89264630198279));
#30069=CARTESIAN_POINT('Ctrl Pts',(0.175274276190664,1.,-1.89264630198279));
#30070=CARTESIAN_POINT('Ctrl Pts',(0.174879405091277,-1.,-1.89788101117148));
#30071=CARTESIAN_POINT('Ctrl Pts',(0.174879405091277,1.,-1.89788101117148));
#30072=CARTESIAN_POINT('Ctrl Pts',(0.174375518661222,-1.,-1.90335253863003));
#30073=CARTESIAN_POINT('Ctrl Pts',(0.174375518661222,1.,-1.90335253863003));
#30074=CARTESIAN_POINT('Ctrl Pts',(0.173776635257984,-1.,-1.90911693975475));
#30075=CARTESIAN_POINT('Ctrl Pts',(0.173776635257984,1.,-1.90911693975475));
#30076=CARTESIAN_POINT('Ctrl Pts',(0.173090695383619,-1.,-1.91511429159681));
#30077=CARTESIAN_POINT('Ctrl Pts',(0.173090695383619,1.,-1.91511429159681));
#30078=CARTESIAN_POINT('Ctrl Pts',(0.172321621259557,-1.,-1.92122334398034));
#30079=CARTESIAN_POINT('Ctrl Pts',(0.172321621259557,1.,-1.92122334398034));
#30080=CARTESIAN_POINT('Ctrl Pts',(0.17147119153296,-1.,-1.92731093582));
#30081=CARTESIAN_POINT('Ctrl Pts',(0.17147119153296,1.,-1.92731093582));
#30082=CARTESIAN_POINT('Ctrl Pts',(0.170541253116136,-1.,-1.93329183155455));
#30083=CARTESIAN_POINT('Ctrl Pts',(0.170541253116136,1.,-1.93329183155455));
#30084=CARTESIAN_POINT('Ctrl Pts',(0.169534904817425,-1.,-1.93915639211497));
#30085=CARTESIAN_POINT('Ctrl Pts',(0.169534904817425,1.,-1.93915639211497));
#30086=CARTESIAN_POINT('Ctrl Pts',(0.168455741607516,-1.,-1.94493757756879));
#30087=CARTESIAN_POINT('Ctrl Pts',(0.168455741607516,1.,-1.94493757756879));
#30088=CARTESIAN_POINT('Ctrl Pts',(0.167307501784469,-1.,-1.95069027794286));
#30089=CARTESIAN_POINT('Ctrl Pts',(0.167307501784469,1.,-1.95069027794286));
#30090=CARTESIAN_POINT('Ctrl Pts',(0.166093592002833,-1.,-1.95646759718755));
#30091=CARTESIAN_POINT('Ctrl Pts',(0.166093592002833,1.,-1.95646759718755));
#30092=CARTESIAN_POINT('Ctrl Pts',(0.1648165689203,-1.,-1.96229379940174));
#30093=CARTESIAN_POINT('Ctrl Pts',(0.1648165689203,1.,-1.96229379940174));
#30094=CARTESIAN_POINT('Ctrl Pts',(0.16347818545776,-1.,-1.96816512678));
#30095=CARTESIAN_POINT('Ctrl Pts',(0.16347818545776,1.,-1.96816512678));
#30096=CARTESIAN_POINT('Ctrl Pts',(0.162079693556302,-1.,-1.97406280235204));
#30097=CARTESIAN_POINT('Ctrl Pts',(0.162079693556302,1.,-1.97406280235204));
#30098=CARTESIAN_POINT('Ctrl Pts',(0.16062206078461,-1.,-1.97996195437557));
#30099=CARTESIAN_POINT('Ctrl Pts',(0.16062206078461,1.,-1.97996195437557));
#30100=CARTESIAN_POINT('Ctrl Pts',(0.159106226437288,-1.,-1.98584238283279));
#30101=CARTESIAN_POINT('Ctrl Pts',(0.159106226437288,1.,-1.98584238283279));
#30102=CARTESIAN_POINT('Ctrl Pts',(0.157533331459215,-1.,-1.99169810931893));
#30103=CARTESIAN_POINT('Ctrl Pts',(0.157533331459215,1.,-1.99169810931893));
#30104=CARTESIAN_POINT('Ctrl Pts',(0.155904629548774,-1.,-1.99753284771487));
#30105=CARTESIAN_POINT('Ctrl Pts',(0.155904629548774,1.,-1.99753284771487));
#30106=CARTESIAN_POINT('Ctrl Pts',(0.154221403049719,-1.,-2.00335565310539));
#30107=CARTESIAN_POINT('Ctrl Pts',(0.154221403049719,1.,-2.00335565310539));
#30108=CARTESIAN_POINT('Ctrl Pts',(0.152484883621452,-1.,-2.00917680318426));
#30109=CARTESIAN_POINT('Ctrl Pts',(0.152484883621452,1.,-2.00917680318426));
#30110=CARTESIAN_POINT('Ctrl Pts',(0.150696157673084,-1.,-2.01500291940243));
#30111=CARTESIAN_POINT('Ctrl Pts',(0.150696157673084,1.,-2.01500291940243));
#30112=CARTESIAN_POINT('Ctrl Pts',(0.148856124775343,-1.,-2.02083464969897));
#30113=CARTESIAN_POINT('Ctrl Pts',(0.148856124775343,1.,-2.02083464969897));
#30114=CARTESIAN_POINT('Ctrl Pts',(0.146965557332586,-1.,-2.02666926182017));
#30115=CARTESIAN_POINT('Ctrl Pts',(0.146965557332586,1.,-2.02666926182017));
#30116=CARTESIAN_POINT('Ctrl Pts',(0.145025140186058,-1.,-2.03250223739941));
#30117=CARTESIAN_POINT('Ctrl Pts',(0.145025140186058,1.,-2.03250223739941));
#30118=CARTESIAN_POINT('Ctrl Pts',(0.143035515058208,-1.,-2.03832911025913));
#30119=CARTESIAN_POINT('Ctrl Pts',(0.143035515058208,1.,-2.03832911025913));
#30120=CARTESIAN_POINT('Ctrl Pts',(0.140997332152545,-1.,-2.04414757947919));
#30121=CARTESIAN_POINT('Ctrl Pts',(0.140997332152545,1.,-2.04414757947919));
#30122=CARTESIAN_POINT('Ctrl Pts',(0.138911255368966,-1.,-2.04995762001333));
#30123=CARTESIAN_POINT('Ctrl Pts',(0.138911255368966,1.,-2.04995762001333));
#30124=CARTESIAN_POINT('Ctrl Pts',(0.136777941218044,-1.,-2.0557604441427));
#30125=CARTESIAN_POINT('Ctrl Pts',(0.136777941218044,1.,-2.0557604441427));
#30126=CARTESIAN_POINT('Ctrl Pts',(0.134598026192107,-1.,-2.06155781517844));
#30127=CARTESIAN_POINT('Ctrl Pts',(0.134598026192107,1.,-2.06155781517844));
#30128=CARTESIAN_POINT('Ctrl Pts',(0.13237211154771,-1.,-2.06735123910319));
#30129=CARTESIAN_POINT('Ctrl Pts',(0.13237211154771,1.,-2.06735123910319));
#30130=CARTESIAN_POINT('Ctrl Pts',(0.1301007483284,-1.,-2.07314114713047));
#30131=CARTESIAN_POINT('Ctrl Pts',(0.1301007483284,1.,-2.07314114713047));
#30132=CARTESIAN_POINT('Ctrl Pts',(0.127784445276116,-1.,-2.07892715110967));
#30133=CARTESIAN_POINT('Ctrl Pts',(0.127784445276116,1.,-2.07892715110967));
#30134=CARTESIAN_POINT('Ctrl Pts',(0.125423679412058,-1.,-2.08470840653628));
#30135=CARTESIAN_POINT('Ctrl Pts',(0.125423679412058,1.,-2.08470840653628));
#30136=CARTESIAN_POINT('Ctrl Pts',(0.123018905621083,-1.,-2.09048392424826));
#30137=CARTESIAN_POINT('Ctrl Pts',(0.123018905621083,1.,-2.09048392424826));
#30138=CARTESIAN_POINT('Ctrl Pts',(0.120570567965129,-1.,-2.09625292867756));
#30139=CARTESIAN_POINT('Ctrl Pts',(0.120570567965129,1.,-2.09625292867756));
#30140=CARTESIAN_POINT('Ctrl Pts',(0.118079107988368,-1.,-2.10201512132945));
#30141=CARTESIAN_POINT('Ctrl Pts',(0.118079107988368,1.,-2.10201512132945));
#30142=CARTESIAN_POINT('Ctrl Pts',(0.11554495768794,-1.,-2.10777050261359));
#30143=CARTESIAN_POINT('Ctrl Pts',(0.11554495768794,1.,-2.10777050261359));
#30144=CARTESIAN_POINT('Ctrl Pts',(0.112968534419746,-1.,-2.11351924490335));
#30145=CARTESIAN_POINT('Ctrl Pts',(0.112968534419746,1.,-2.11351924490335));
#30146=CARTESIAN_POINT('Ctrl Pts',(0.11035023613502,-1.,-2.11926155590849));
#30147=CARTESIAN_POINT('Ctrl Pts',(0.11035023613502,1.,-2.11926155590849));
#30148=CARTESIAN_POINT('Ctrl Pts',(0.107690435231068,-1.,-2.12499752306927));
#30149=CARTESIAN_POINT('Ctrl Pts',(0.107690435231068,1.,-2.12499752306927));
#30150=CARTESIAN_POINT('Ctrl Pts',(0.104989479152703,-1.,-2.1307270488718));
#30151=CARTESIAN_POINT('Ctrl Pts',(0.104989479152703,1.,-2.1307270488718));
#30152=CARTESIAN_POINT('Ctrl Pts',(0.102247700556064,-1.,-2.13644992667052));
#30153=CARTESIAN_POINT('Ctrl Pts',(0.102247700556064,1.,-2.13644992667052));
#30154=CARTESIAN_POINT('Ctrl Pts',(0.0994654261990743,-1.,-2.14216588395974));
#30155=CARTESIAN_POINT('Ctrl Pts',(0.0994654261990743,1.,-2.14216588395974));
#30156=CARTESIAN_POINT('Ctrl Pts',(0.0966429852305689,-1.,-2.14787463531864));
#30157=CARTESIAN_POINT('Ctrl Pts',(0.0966429852305689,1.,-2.14787463531864));
#30158=CARTESIAN_POINT('Ctrl Pts',(0.0937807218868345,-1.,-2.15357593978377));
#30159=CARTESIAN_POINT('Ctrl Pts',(0.0937807218868345,1.,-2.15357593978377));
#30160=CARTESIAN_POINT('Ctrl Pts',(0.0908789888108266,-1.,-2.15926961544808));
#30161=CARTESIAN_POINT('Ctrl Pts',(0.0908789888108266,1.,-2.15926961544808));
#30162=CARTESIAN_POINT('Ctrl Pts',(0.0879381291387823,-1.,-2.16495552645275));
#30163=CARTESIAN_POINT('Ctrl Pts',(0.0879381291387823,1.,-2.16495552645275));
#30164=CARTESIAN_POINT('Ctrl Pts',(0.0849584620835643,-1.,-2.17063357871031));
#30165=CARTESIAN_POINT('Ctrl Pts',(0.0849584620835643,1.,-2.17063357871031));
#30166=CARTESIAN_POINT('Ctrl Pts',(0.0819402680871939,-1.,-2.1763037121106));
#30167=CARTESIAN_POINT('Ctrl Pts',(0.0819402680871939,1.,-2.1763037121106));
#30168=CARTESIAN_POINT('Ctrl Pts',(0.0788837727683228,-1.,-2.18196589448304));
#30169=CARTESIAN_POINT('Ctrl Pts',(0.0788837727683228,1.,-2.18196589448304));
#30170=CARTESIAN_POINT('Ctrl Pts',(0.0757891465833411,-1.,-2.1876201139874));
#30171=CARTESIAN_POINT('Ctrl Pts',(0.0757891465833411,1.,-2.1876201139874));
#30172=CARTESIAN_POINT('Ctrl Pts',(0.0732830357304276,-1.,-2.19213712012956));
#30173=CARTESIAN_POINT('Ctrl Pts',(0.0732830357304276,1.,-2.19213712012956));
#30174=CARTESIAN_POINT('Ctrl Pts',(0.0713863779524627,-1.,-2.19552129483562));
#30175=CARTESIAN_POINT('Ctrl Pts',(0.0713863779524627,1.,-2.19552129483562));
#30176=CARTESIAN_POINT('Ctrl Pts',(0.0701143536324926,-1.,-2.19777582085261));
#30177=CARTESIAN_POINT('Ctrl Pts',(0.0701143536324926,1.,-2.19777582085261));
#30178=CARTESIAN_POINT('Ctrl Pts',(0.0694764450219584,-1.,-2.19890268624765));
#30179=CARTESIAN_POINT('Ctrl Pts',(0.0694764450219584,1.,-2.19890268624765));
#30180=CARTESIAN_POINT('',(0.163289472382896,1.,-1.74236521665491));
#30181=CARTESIAN_POINT('Ctrl Pts',(0.163289472382896,1.,-1.74236521665491));
#30182=CARTESIAN_POINT('Ctrl Pts',(0.163814161002474,1.,-1.74720349503904));
#30183=CARTESIAN_POINT('Ctrl Pts',(0.164834765708484,1.,-1.75666056640041));
#30184=CARTESIAN_POINT('Ctrl Pts',(0.166279355148738,1.,-1.77018771687692));
#30185=CARTESIAN_POINT('Ctrl Pts',(0.16803277280837,1.,-1.78690649988931));
#30186=CARTESIAN_POINT('Ctrl Pts',(0.169936923908078,1.,-1.80561530633924));
#30187=CARTESIAN_POINT('Ctrl Pts',(0.171554770207306,1.,-1.82215766815414));
#30188=CARTESIAN_POINT('Ctrl Pts',(0.17288944289442,1.,-1.83658380530747));
#30189=CARTESIAN_POINT('Ctrl Pts',(0.173946627589401,1.,-1.84898113200543));
#30190=CARTESIAN_POINT('Ctrl Pts',(0.174735259276856,1.,-1.85948367089838));
#30191=CARTESIAN_POINT('Ctrl Pts',(0.175268337590901,1.,-1.86828349694972));
#30192=CARTESIAN_POINT('Ctrl Pts',(0.175563480746205,1.,-1.87563767773249));
#30193=CARTESIAN_POINT('Ctrl Pts',(0.175644148889271,1.,-1.88188663144846));
#30194=CARTESIAN_POINT('Ctrl Pts',(0.175538155840286,1.,-1.88742606272818));
#30195=CARTESIAN_POINT('Ctrl Pts',(0.175274276190664,1.,-1.89264630198279));
#30196=CARTESIAN_POINT('Ctrl Pts',(0.174879405091277,1.,-1.89788101117148));
#30197=CARTESIAN_POINT('Ctrl Pts',(0.174375518661222,1.,-1.90335253863003));
#30198=CARTESIAN_POINT('Ctrl Pts',(0.173776635257984,1.,-1.90911693975475));
#30199=CARTESIAN_POINT('Ctrl Pts',(0.173090695383619,1.,-1.91511429159681));
#30200=CARTESIAN_POINT('Ctrl Pts',(0.172321621259557,1.,-1.92122334398034));
#30201=CARTESIAN_POINT('Ctrl Pts',(0.17147119153296,1.,-1.92731093582));
#30202=CARTESIAN_POINT('Ctrl Pts',(0.170541253116136,1.,-1.93329183155455));
#30203=CARTESIAN_POINT('Ctrl Pts',(0.169534904817425,1.,-1.93915639211497));
#30204=CARTESIAN_POINT('Ctrl Pts',(0.168455741607516,1.,-1.94493757756879));
#30205=CARTESIAN_POINT('Ctrl Pts',(0.167307501784469,1.,-1.95069027794286));
#30206=CARTESIAN_POINT('Ctrl Pts',(0.166093592002833,1.,-1.95646759718755));
#30207=CARTESIAN_POINT('Ctrl Pts',(0.1648165689203,1.,-1.96229379940174));
#30208=CARTESIAN_POINT('Ctrl Pts',(0.16347818545776,1.,-1.96816512678));
#30209=CARTESIAN_POINT('Ctrl Pts',(0.162079693556302,1.,-1.97406280235204));
#30210=CARTESIAN_POINT('Ctrl Pts',(0.16062206078461,1.,-1.97996195437557));
#30211=CARTESIAN_POINT('Ctrl Pts',(0.159106226437288,1.,-1.98584238283279));
#30212=CARTESIAN_POINT('Ctrl Pts',(0.157533331459215,1.,-1.99169810931893));
#30213=CARTESIAN_POINT('Ctrl Pts',(0.155904629548774,1.,-1.99753284771487));
#30214=CARTESIAN_POINT('Ctrl Pts',(0.154221403049719,1.,-2.00335565310539));
#30215=CARTESIAN_POINT('Ctrl Pts',(0.152484883621452,1.,-2.00917680318426));
#30216=CARTESIAN_POINT('Ctrl Pts',(0.150696157673084,1.,-2.01500291940243));
#30217=CARTESIAN_POINT('Ctrl Pts',(0.148856124775343,1.,-2.02083464969897));
#30218=CARTESIAN_POINT('Ctrl Pts',(0.146965557332586,1.,-2.02666926182017));
#30219=CARTESIAN_POINT('Ctrl Pts',(0.145025140186058,1.,-2.03250223739941));
#30220=CARTESIAN_POINT('Ctrl Pts',(0.143035515058208,1.,-2.03832911025913));
#30221=CARTESIAN_POINT('Ctrl Pts',(0.140997332152545,1.,-2.04414757947919));
#30222=CARTESIAN_POINT('Ctrl Pts',(0.138911255368966,1.,-2.04995762001333));
#30223=CARTESIAN_POINT('Ctrl Pts',(0.136777941218044,1.,-2.0557604441427));
#30224=CARTESIAN_POINT('Ctrl Pts',(0.134598026192107,1.,-2.06155781517844));
#30225=CARTESIAN_POINT('Ctrl Pts',(0.13237211154771,1.,-2.06735123910319));
#30226=CARTESIAN_POINT('Ctrl Pts',(0.1301007483284,1.,-2.07314114713047));
#30227=CARTESIAN_POINT('Ctrl Pts',(0.127784445276116,1.,-2.07892715110967));
#30228=CARTESIAN_POINT('Ctrl Pts',(0.125423679412058,1.,-2.08470840653628));
#30229=CARTESIAN_POINT('Ctrl Pts',(0.123018905621083,1.,-2.09048392424826));
#30230=CARTESIAN_POINT('Ctrl Pts',(0.120570567965129,1.,-2.09625292867756));
#30231=CARTESIAN_POINT('Ctrl Pts',(0.118079107988368,1.,-2.10201512132945));
#30232=CARTESIAN_POINT('Ctrl Pts',(0.11554495768794,1.,-2.10777050261359));
#30233=CARTESIAN_POINT('Ctrl Pts',(0.112968534419746,1.,-2.11351924490335));
#30234=CARTESIAN_POINT('Ctrl Pts',(0.11035023613502,1.,-2.11926155590849));
#30235=CARTESIAN_POINT('Ctrl Pts',(0.107690435231068,1.,-2.12499752306927));
#30236=CARTESIAN_POINT('Ctrl Pts',(0.104989479152703,1.,-2.1307270488718));
#30237=CARTESIAN_POINT('Ctrl Pts',(0.102247700556064,1.,-2.13644992667052));
#30238=CARTESIAN_POINT('Ctrl Pts',(0.0994654261990743,1.,-2.14216588395974));
#30239=CARTESIAN_POINT('Ctrl Pts',(0.0966429852305689,1.,-2.14787463531864));
#30240=CARTESIAN_POINT('Ctrl Pts',(0.0937807218868345,1.,-2.15357593978377));
#30241=CARTESIAN_POINT('Ctrl Pts',(0.0908789888108266,1.,-2.15926961544808));
#30242=CARTESIAN_POINT('Ctrl Pts',(0.0879381291387823,1.,-2.16495552645275));
#30243=CARTESIAN_POINT('Ctrl Pts',(0.0849584620835643,1.,-2.17063357871031));
#30244=CARTESIAN_POINT('Ctrl Pts',(0.0819402680871939,1.,-2.1763037121106));
#30245=CARTESIAN_POINT('Ctrl Pts',(0.0788837727683228,1.,-2.18196589448304));
#30246=CARTESIAN_POINT('Ctrl Pts',(0.0757891465833411,1.,-2.1876201139874));
#30247=CARTESIAN_POINT('Ctrl Pts',(0.0732830357304276,1.,-2.19213712012956));
#30248=CARTESIAN_POINT('Ctrl Pts',(0.0713863779524627,1.,-2.19552129483562));
#30249=CARTESIAN_POINT('Ctrl Pts',(0.0701143536324926,1.,-2.19777582085261));
#30250=CARTESIAN_POINT('Ctrl Pts',(0.0694764450219584,1.,-2.19890268624765));
#30251=CARTESIAN_POINT('',(0.163289472382896,0.,-1.74236521665491));
#30252=CARTESIAN_POINT('Origin',(0.,0.,0.));
#30253=CARTESIAN_POINT('',(0.383122945602004,1.,-1.7075470150345));
#30254=CARTESIAN_POINT('Origin',(0.,1.,0.));
#30255=CARTESIAN_POINT('',(0.383122945602004,0.,-1.7075470150345));
#30256=CARTESIAN_POINT('Ctrl Pts',(0.61342227326009,-1.,-2.11275013067528));
#30257=CARTESIAN_POINT('Ctrl Pts',(0.61342227326009,1.,-2.11275013067528));
#30258=CARTESIAN_POINT('Ctrl Pts',(0.61246736556225,-1.,-2.11187554260142));
#30259=CARTESIAN_POINT('Ctrl Pts',(0.61246736556225,1.,-2.11187554260142));
#30260=CARTESIAN_POINT('Ctrl Pts',(0.610560911691113,-1.,-2.11012443807661));
#30261=CARTESIAN_POINT('Ctrl Pts',(0.610560911691113,1.,-2.11012443807661));
#30262=CARTESIAN_POINT('Ctrl Pts',(0.607711315456826,-1.,-2.10749199615859));
#30263=CARTESIAN_POINT('Ctrl Pts',(0.607711315456826,1.,-2.10749199615859));
#30264=CARTESIAN_POINT('Ctrl Pts',(0.603932030738212,-1.,-2.10397049887709));
#30265=CARTESIAN_POINT('Ctrl Pts',(0.603932030738212,1.,-2.10397049887709));
#30266=CARTESIAN_POINT('Ctrl Pts',(0.599241616422144,-1.,-2.09954930865331));
#30267=CARTESIAN_POINT('Ctrl Pts',(0.599241616422144,1.,-2.09954930865331));
#30268=CARTESIAN_POINT('Ctrl Pts',(0.594585006052823,-1.,-2.09510876220501));
#30269=CARTESIAN_POINT('Ctrl Pts',(0.594585006052823,1.,-2.09510876220501));
#30270=CARTESIAN_POINT('Ctrl Pts',(0.589962365403189,-1.,-2.09064881812053));
#30271=CARTESIAN_POINT('Ctrl Pts',(0.589962365403189,1.,-2.09064881812053));
#30272=CARTESIAN_POINT('Ctrl Pts',(0.585373918990895,-1.,-2.086169437277));
#30273=CARTESIAN_POINT('Ctrl Pts',(0.585373918990895,1.,-2.086169437277));
#30274=CARTESIAN_POINT('Ctrl Pts',(0.580819952107256,-1.,-2.08167059018138));
#30275=CARTESIAN_POINT('Ctrl Pts',(0.580819952107256,1.,-2.08167059018138));
#30276=CARTESIAN_POINT('Ctrl Pts',(0.576300797416274,-1.,-2.07715226767361));
#30277=CARTESIAN_POINT('Ctrl Pts',(0.576300797416274,1.,-2.07715226767361));
#30278=CARTESIAN_POINT('Ctrl Pts',(0.571816823242411,-1.,-2.07261449292758));
#30279=CARTESIAN_POINT('Ctrl Pts',(0.571816823242411,1.,-2.07261449292758));
#30280=CARTESIAN_POINT('Ctrl Pts',(0.567368421181229,-1.,-2.06805732997383));
#30281=CARTESIAN_POINT('Ctrl Pts',(0.567368421181229,1.,-2.06805732997383));
#30282=CARTESIAN_POINT('Ctrl Pts',(0.562955993082574,-1.,-2.06348090160697));
#30283=CARTESIAN_POINT('Ctrl Pts',(0.562955993082574,1.,-2.06348090160697));
#30284=CARTESIAN_POINT('Ctrl Pts',(0.558579940185467,-1.,-2.05888537756571));
#30285=CARTESIAN_POINT('Ctrl Pts',(0.558579940185467,1.,-2.05888537756571));
#30286=CARTESIAN_POINT('Ctrl Pts',(0.554240657464109,-1.,-2.05427091604482));
#30287=CARTESIAN_POINT('Ctrl Pts',(0.554240657464109,1.,-2.05427091604482));
#30288=CARTESIAN_POINT('Ctrl Pts',(0.549938525150342,-1.,-2.04963761077974));
#30289=CARTESIAN_POINT('Ctrl Pts',(0.549938525150342,1.,-2.04963761077974));
#30290=CARTESIAN_POINT('Ctrl Pts',(0.545673903817348,-1.,-2.0449854471456));
#30291=CARTESIAN_POINT('Ctrl Pts',(0.545673903817348,1.,-2.0449854471456));
#30292=CARTESIAN_POINT('Ctrl Pts',(0.54144712061552,-1.,-2.0403142269048));
#30293=CARTESIAN_POINT('Ctrl Pts',(0.54144712061552,1.,-2.0403142269048));
#30294=CARTESIAN_POINT('Ctrl Pts',(0.537258489833134,-1.,-2.03562362953993));
#30295=CARTESIAN_POINT('Ctrl Pts',(0.537258489833134,1.,-2.03562362953993));
#30296=CARTESIAN_POINT('Ctrl Pts',(0.533108355132905,-1.,-2.03091336214401));
#30297=CARTESIAN_POINT('Ctrl Pts',(0.533108355132905,1.,-2.03091336214401));
#30298=CARTESIAN_POINT('Ctrl Pts',(0.52899712724191,-1.,-2.02618329083289));
#30299=CARTESIAN_POINT('Ctrl Pts',(0.52899712724191,1.,-2.02618329083289));
#30300=CARTESIAN_POINT('Ctrl Pts',(0.524925318333518,-1.,-2.02143356304712));
#30301=CARTESIAN_POINT('Ctrl Pts',(0.524925318333518,1.,-2.02143356304712));
#30302=CARTESIAN_POINT('Ctrl Pts',(0.520893590399428,-1.,-2.01666477917306));
#30303=CARTESIAN_POINT('Ctrl Pts',(0.520893590399428,1.,-2.01666477917306));
#30304=CARTESIAN_POINT('Ctrl Pts',(0.516902681728733,-1.,-2.01187773939257));
#30305=CARTESIAN_POINT('Ctrl Pts',(0.516902681728733,1.,-2.01187773939257));
#30306=CARTESIAN_POINT('Ctrl Pts',(0.512953306961813,-1.,-2.00707309946955));
#30307=CARTESIAN_POINT('Ctrl Pts',(0.512953306961813,1.,-2.00707309946955));
#30308=CARTESIAN_POINT('Ctrl Pts',(0.509046069886152,-1.,-2.00225107134733));
#30309=CARTESIAN_POINT('Ctrl Pts',(0.509046069886152,1.,-2.00225107134733));
#30310=CARTESIAN_POINT('Ctrl Pts',(0.505181361323011,-1.,-1.99741107463567));
#30311=CARTESIAN_POINT('Ctrl Pts',(0.505181361323011,1.,-1.99741107463567));
#30312=CARTESIAN_POINT('Ctrl Pts',(0.501359287727129,-1.,-1.9925514912615));
#30313=CARTESIAN_POINT('Ctrl Pts',(0.501359287727129,1.,-1.9925514912615));
#30314=CARTESIAN_POINT('Ctrl Pts',(0.497579909545564,-1.,-1.98767044752929));
#30315=CARTESIAN_POINT('Ctrl Pts',(0.497579909545564,1.,-1.98767044752929));
#30316=CARTESIAN_POINT('Ctrl Pts',(0.493843476541492,-1.,-1.9827665876182));
#30317=CARTESIAN_POINT('Ctrl Pts',(0.493843476541492,1.,-1.9827665876182));
#30318=CARTESIAN_POINT('Ctrl Pts',(0.490150627860955,-1.,-1.97783973019229));
#30319=CARTESIAN_POINT('Ctrl Pts',(0.490150627860955,1.,-1.97783973019229));
#30320=CARTESIAN_POINT('Ctrl Pts',(0.486502692907661,-1.,-1.97289186263272));
#30321=CARTESIAN_POINT('Ctrl Pts',(0.486502692907661,1.,-1.97289186263272));
#30322=CARTESIAN_POINT('Ctrl Pts',(0.482901662120686,-1.,-1.96792703422358));
#30323=CARTESIAN_POINT('Ctrl Pts',(0.482901662120686,1.,-1.96792703422358));
#30324=CARTESIAN_POINT('Ctrl Pts',(0.479349583074846,-1.,-1.96294933055938));
#30325=CARTESIAN_POINT('Ctrl Pts',(0.479349583074846,1.,-1.96294933055938));
#30326=CARTESIAN_POINT('Ctrl Pts',(0.475848034683171,-1.,-1.95796111148175));
#30327=CARTESIAN_POINT('Ctrl Pts',(0.475848034683171,1.,-1.95796111148175));
#30328=CARTESIAN_POINT('Ctrl Pts',(0.472397672264079,-1.,-1.95296148278136));
#30329=CARTESIAN_POINT('Ctrl Pts',(0.472397672264079,1.,-1.95296148278136));
#30330=CARTESIAN_POINT('Ctrl Pts',(0.468997482913158,-1.,-1.94794381136524));
#30331=CARTESIAN_POINT('Ctrl Pts',(0.468997482913158,1.,-1.94794381136524));
#30332=CARTESIAN_POINT('Ctrl Pts',(0.465645462026064,-1.,-1.94289794196205));
#30333=CARTESIAN_POINT('Ctrl Pts',(0.465645462026064,1.,-1.94289794196205));
#30334=CARTESIAN_POINT('Ctrl Pts',(0.462340031009087,-1.,-1.93781486640834));
#30335=CARTESIAN_POINT('Ctrl Pts',(0.462340031009087,1.,-1.93781486640834));
#30336=CARTESIAN_POINT('Ctrl Pts',(0.459081234547931,-1.,-1.93269066517936));
#30337=CARTESIAN_POINT('Ctrl Pts',(0.459081234547931,1.,-1.93269066517936));
#30338=CARTESIAN_POINT('Ctrl Pts',(0.455872005174335,-1.,-1.92753067150461));
#30339=CARTESIAN_POINT('Ctrl Pts',(0.455872005174335,1.,-1.92753067150461));
#30340=CARTESIAN_POINT('Ctrl Pts',(0.452719478359356,-1.,-1.9223538064847));
#30341=CARTESIAN_POINT('Ctrl Pts',(0.452719478359356,1.,-1.9223538064847));
#30342=CARTESIAN_POINT('Ctrl Pts',(0.449632260106572,-1.,-1.91718342555717));
#30343=CARTESIAN_POINT('Ctrl Pts',(0.449632260106572,1.,-1.91718342555717));
#30344=CARTESIAN_POINT('Ctrl Pts',(0.446617343485651,-1.,-1.91203699981095));
#30345=CARTESIAN_POINT('Ctrl Pts',(0.446617343485651,1.,-1.91203699981095));
#30346=CARTESIAN_POINT('Ctrl Pts',(0.44367755684917,-1.,-1.90691756144906));
#30347=CARTESIAN_POINT('Ctrl Pts',(0.44367755684917,1.,-1.90691756144906));
#30348=CARTESIAN_POINT('Ctrl Pts',(0.44080783370416,-1.,-1.90180124389137));
#30349=CARTESIAN_POINT('Ctrl Pts',(0.44080783370416,1.,-1.90180124389137));
#30350=CARTESIAN_POINT('Ctrl Pts',(0.437995003948443,-1.,-1.89663648956549));
#30351=CARTESIAN_POINT('Ctrl Pts',(0.437995003948443,1.,-1.89663648956549));
#30352=CARTESIAN_POINT('Ctrl Pts',(0.43522566096358,-1.,-1.89136993975585));
#30353=CARTESIAN_POINT('Ctrl Pts',(0.43522566096358,1.,-1.89136993975585));
#30354=CARTESIAN_POINT('Ctrl Pts',(0.432493038548833,-1.,-1.88596913666828));
#30355=CARTESIAN_POINT('Ctrl Pts',(0.432493038548833,1.,-1.88596913666828));
#30356=CARTESIAN_POINT('Ctrl Pts',(0.429803062482217,-1.,-1.88044229001779));
#30357=CARTESIAN_POINT('Ctrl Pts',(0.429803062482217,1.,-1.88044229001779));
#30358=CARTESIAN_POINT('Ctrl Pts',(0.427183828518743,-1.,-1.87486989291334));
#30359=CARTESIAN_POINT('Ctrl Pts',(0.427183828518743,1.,-1.87486989291334));
#30360=CARTESIAN_POINT('Ctrl Pts',(0.424678177290876,-1.,-1.8693780394412));
#30361=CARTESIAN_POINT('Ctrl Pts',(0.424678177290876,1.,-1.8693780394412));
#30362=CARTESIAN_POINT('Ctrl Pts',(0.422327307417884,-1.,-1.86408083333863));
#30363=CARTESIAN_POINT('Ctrl Pts',(0.422327307417884,1.,-1.86408083333863));
#30364=CARTESIAN_POINT('Ctrl Pts',(0.420157287975583,-1.,-1.8590328109667));
#30365=CARTESIAN_POINT('Ctrl Pts',(0.420157287975583,1.,-1.8590328109667));
#30366=CARTESIAN_POINT('Ctrl Pts',(0.418164129144045,-1.,-1.8541763285645));
#30367=CARTESIAN_POINT('Ctrl Pts',(0.418164129144045,1.,-1.8541763285645));
#30368=CARTESIAN_POINT('Ctrl Pts',(0.416300022039885,-1.,-1.84929312930314));
#30369=CARTESIAN_POINT('Ctrl Pts',(0.416300022039885,1.,-1.84929312930314));
#30370=CARTESIAN_POINT('Ctrl Pts',(0.414487438255542,-1.,-1.84405757074218));
#30371=CARTESIAN_POINT('Ctrl Pts',(0.414487438255542,1.,-1.84405757074218));
#30372=CARTESIAN_POINT('Ctrl Pts',(0.412633125322945,-1.,-1.8380895347617));
#30373=CARTESIAN_POINT('Ctrl Pts',(0.412633125322945,1.,-1.8380895347617));
#30374=CARTESIAN_POINT('Ctrl Pts',(0.410641256301276,-1.,-1.83100408895047));
#30375=CARTESIAN_POINT('Ctrl Pts',(0.410641256301276,1.,-1.83100408895047));
#30376=CARTESIAN_POINT('Ctrl Pts',(0.408428948106227,-1.,-1.82247022677562));
#30377=CARTESIAN_POINT('Ctrl Pts',(0.408428948106227,1.,-1.82247022677562));
#30378=CARTESIAN_POINT('Ctrl Pts',(0.405933518407175,-1.,-1.81223801812013));
#30379=CARTESIAN_POINT('Ctrl Pts',(0.405933518407175,1.,-1.81223801812013));
#30380=CARTESIAN_POINT('Ctrl Pts',(0.403107976163396,-1.,-1.80012077173238));
#30381=CARTESIAN_POINT('Ctrl Pts',(0.403107976163396,1.,-1.80012077173238));
#30382=CARTESIAN_POINT('Ctrl Pts',(0.399919403774155,-1.,-1.78598826343754));
#30383=CARTESIAN_POINT('Ctrl Pts',(0.399919403774155,1.,-1.78598826343754));
#30384=CARTESIAN_POINT('Ctrl Pts',(0.396346196110688,-1.,-1.76975560043442));
#30385=CARTESIAN_POINT('Ctrl Pts',(0.396346196110688,1.,-1.76975560043442));
#30386=CARTESIAN_POINT('Ctrl Pts',(0.392375812285395,-1.,-1.75137405310193));
#30387=CARTESIAN_POINT('Ctrl Pts',(0.392375812285395,1.,-1.75137405310193));
#30388=CARTESIAN_POINT('Ctrl Pts',(0.388877023502615,-1.,-1.73493170972829));
#30389=CARTESIAN_POINT('Ctrl Pts',(0.388877023502615,1.,-1.73493170972829));
#30390=CARTESIAN_POINT('Ctrl Pts',(0.386070790323281,-1.,-1.72162022244582));
#30391=CARTESIAN_POINT('Ctrl Pts',(0.386070790323281,1.,-1.72162022244582));
#30392=CARTESIAN_POINT('Ctrl Pts',(0.384119047314215,-1.,-1.71231062891398));
#30393=CARTESIAN_POINT('Ctrl Pts',(0.384119047314215,1.,-1.71231062891398));
#30394=CARTESIAN_POINT('Ctrl Pts',(0.383122945602004,-1.,-1.7075470150345));
#30395=CARTESIAN_POINT('Ctrl Pts',(0.383122945602004,1.,-1.7075470150345));
#30396=CARTESIAN_POINT('',(0.61342227326009,1.,-2.11275013067528));
#30397=CARTESIAN_POINT('Ctrl Pts',(0.61342227326009,1.,-2.11275013067528));
#30398=CARTESIAN_POINT('Ctrl Pts',(0.61246736556225,1.,-2.11187554260142));
#30399=CARTESIAN_POINT('Ctrl Pts',(0.610560911691113,1.,-2.11012443807661));
#30400=CARTESIAN_POINT('Ctrl Pts',(0.607711315456826,1.,-2.10749199615859));
#30401=CARTESIAN_POINT('Ctrl Pts',(0.603932030738212,1.,-2.10397049887709));
#30402=CARTESIAN_POINT('Ctrl Pts',(0.599241616422144,1.,-2.09954930865331));
#30403=CARTESIAN_POINT('Ctrl Pts',(0.594585006052823,1.,-2.09510876220501));
#30404=CARTESIAN_POINT('Ctrl Pts',(0.589962365403189,1.,-2.09064881812053));
#30405=CARTESIAN_POINT('Ctrl Pts',(0.585373918990895,1.,-2.086169437277));
#30406=CARTESIAN_POINT('Ctrl Pts',(0.580819952107256,1.,-2.08167059018138));
#30407=CARTESIAN_POINT('Ctrl Pts',(0.576300797416274,1.,-2.07715226767361));
#30408=CARTESIAN_POINT('Ctrl Pts',(0.571816823242411,1.,-2.07261449292758));
#30409=CARTESIAN_POINT('Ctrl Pts',(0.567368421181229,1.,-2.06805732997383));
#30410=CARTESIAN_POINT('Ctrl Pts',(0.562955993082574,1.,-2.06348090160697));
#30411=CARTESIAN_POINT('Ctrl Pts',(0.558579940185467,1.,-2.05888537756571));
#30412=CARTESIAN_POINT('Ctrl Pts',(0.554240657464109,1.,-2.05427091604482));
#30413=CARTESIAN_POINT('Ctrl Pts',(0.549938525150342,1.,-2.04963761077974));
#30414=CARTESIAN_POINT('Ctrl Pts',(0.545673903817348,1.,-2.0449854471456));
#30415=CARTESIAN_POINT('Ctrl Pts',(0.54144712061552,1.,-2.0403142269048));
#30416=CARTESIAN_POINT('Ctrl Pts',(0.537258489833134,1.,-2.03562362953993));
#30417=CARTESIAN_POINT('Ctrl Pts',(0.533108355132905,1.,-2.03091336214401));
#30418=CARTESIAN_POINT('Ctrl Pts',(0.52899712724191,1.,-2.02618329083289));
#30419=CARTESIAN_POINT('Ctrl Pts',(0.524925318333518,1.,-2.02143356304712));
#30420=CARTESIAN_POINT('Ctrl Pts',(0.520893590399428,1.,-2.01666477917306));
#30421=CARTESIAN_POINT('Ctrl Pts',(0.516902681728733,1.,-2.01187773939257));
#30422=CARTESIAN_POINT('Ctrl Pts',(0.512953306961813,1.,-2.00707309946955));
#30423=CARTESIAN_POINT('Ctrl Pts',(0.509046069886152,1.,-2.00225107134733));
#30424=CARTESIAN_POINT('Ctrl Pts',(0.505181361323011,1.,-1.99741107463567));
#30425=CARTESIAN_POINT('Ctrl Pts',(0.501359287727129,1.,-1.9925514912615));
#30426=CARTESIAN_POINT('Ctrl Pts',(0.497579909545564,1.,-1.98767044752929));
#30427=CARTESIAN_POINT('Ctrl Pts',(0.493843476541492,1.,-1.9827665876182));
#30428=CARTESIAN_POINT('Ctrl Pts',(0.490150627860955,1.,-1.97783973019229));
#30429=CARTESIAN_POINT('Ctrl Pts',(0.486502692907661,1.,-1.97289186263272));
#30430=CARTESIAN_POINT('Ctrl Pts',(0.482901662120686,1.,-1.96792703422358));
#30431=CARTESIAN_POINT('Ctrl Pts',(0.479349583074846,1.,-1.96294933055938));
#30432=CARTESIAN_POINT('Ctrl Pts',(0.475848034683171,1.,-1.95796111148175));
#30433=CARTESIAN_POINT('Ctrl Pts',(0.472397672264079,1.,-1.95296148278136));
#30434=CARTESIAN_POINT('Ctrl Pts',(0.468997482913158,1.,-1.94794381136524));
#30435=CARTESIAN_POINT('Ctrl Pts',(0.465645462026064,1.,-1.94289794196205));
#30436=CARTESIAN_POINT('Ctrl Pts',(0.462340031009087,1.,-1.93781486640834));
#30437=CARTESIAN_POINT('Ctrl Pts',(0.459081234547931,1.,-1.93269066517936));
#30438=CARTESIAN_POINT('Ctrl Pts',(0.455872005174335,1.,-1.92753067150461));
#30439=CARTESIAN_POINT('Ctrl Pts',(0.452719478359356,1.,-1.9223538064847));
#30440=CARTESIAN_POINT('Ctrl Pts',(0.449632260106572,1.,-1.91718342555717));
#30441=CARTESIAN_POINT('Ctrl Pts',(0.446617343485651,1.,-1.91203699981095));
#30442=CARTESIAN_POINT('Ctrl Pts',(0.44367755684917,1.,-1.90691756144906));
#30443=CARTESIAN_POINT('Ctrl Pts',(0.44080783370416,1.,-1.90180124389137));
#30444=CARTESIAN_POINT('Ctrl Pts',(0.437995003948443,1.,-1.89663648956549));
#30445=CARTESIAN_POINT('Ctrl Pts',(0.43522566096358,1.,-1.89136993975585));
#30446=CARTESIAN_POINT('Ctrl Pts',(0.432493038548833,1.,-1.88596913666828));
#30447=CARTESIAN_POINT('Ctrl Pts',(0.429803062482217,1.,-1.88044229001779));
#30448=CARTESIAN_POINT('Ctrl Pts',(0.427183828518743,1.,-1.87486989291334));
#30449=CARTESIAN_POINT('Ctrl Pts',(0.424678177290876,1.,-1.8693780394412));
#30450=CARTESIAN_POINT('Ctrl Pts',(0.422327307417884,1.,-1.86408083333863));
#30451=CARTESIAN_POINT('Ctrl Pts',(0.420157287975583,1.,-1.8590328109667));
#30452=CARTESIAN_POINT('Ctrl Pts',(0.418164129144045,1.,-1.8541763285645));
#30453=CARTESIAN_POINT('Ctrl Pts',(0.416300022039885,1.,-1.84929312930314));
#30454=CARTESIAN_POINT('Ctrl Pts',(0.414487438255542,1.,-1.84405757074218));
#30455=CARTESIAN_POINT('Ctrl Pts',(0.412633125322945,1.,-1.8380895347617));
#30456=CARTESIAN_POINT('Ctrl Pts',(0.410641256301276,1.,-1.83100408895047));
#30457=CARTESIAN_POINT('Ctrl Pts',(0.408428948106227,1.,-1.82247022677562));
#30458=CARTESIAN_POINT('Ctrl Pts',(0.405933518407175,1.,-1.81223801812013));
#30459=CARTESIAN_POINT('Ctrl Pts',(0.403107976163396,1.,-1.80012077173238));
#30460=CARTESIAN_POINT('Ctrl Pts',(0.399919403774155,1.,-1.78598826343754));
#30461=CARTESIAN_POINT('Ctrl Pts',(0.396346196110688,1.,-1.76975560043442));
#30462=CARTESIAN_POINT('Ctrl Pts',(0.392375812285395,1.,-1.75137405310193));
#30463=CARTESIAN_POINT('Ctrl Pts',(0.388877023502615,1.,-1.73493170972829));
#30464=CARTESIAN_POINT('Ctrl Pts',(0.386070790323281,1.,-1.72162022244582));
#30465=CARTESIAN_POINT('Ctrl Pts',(0.384119047314215,1.,-1.71231062891398));
#30466=CARTESIAN_POINT('Ctrl Pts',(0.383122945602004,1.,-1.7075470150345));
#30467=CARTESIAN_POINT('',(0.61342227326009,0.,-2.11275013067528));
#30468=CARTESIAN_POINT('Origin',(0.745574324794401,0.,-2.0698113262342));
#30469=CARTESIAN_POINT('',(0.745574324794401,1.,-2.0698113262342));
#30470=CARTESIAN_POINT('',(0.61342227326009,1.,-2.11275013067528));
#30471=CARTESIAN_POINT('',(0.745574324794401,0.,-2.0698113262342));
#30472=CARTESIAN_POINT('Ctrl Pts',(0.693717979106306,-1.,-1.60662857109684));
#30473=CARTESIAN_POINT('Ctrl Pts',(0.693717979106306,1.,-1.60662857109684));
#30474=CARTESIAN_POINT('Ctrl Pts',(0.695712097881194,-1.,-1.61106790958151));
#30475=CARTESIAN_POINT('Ctrl Pts',(0.695712097881194,1.,-1.61106790958151));
#30476=CARTESIAN_POINT('Ctrl Pts',(0.699605146405088,-1.,-1.61974673472612));
#30477=CARTESIAN_POINT('Ctrl Pts',(0.699605146405088,1.,-1.61974673472612));
#30478=CARTESIAN_POINT('Ctrl Pts',(0.705159151988319,-1.,-1.63216541664676));
#30479=CARTESIAN_POINT('Ctrl Pts',(0.705159151988319,1.,-1.63216541664676));
#30480=CARTESIAN_POINT('Ctrl Pts',(0.711993139355394,-1.,-1.64752408832016));
#30481=CARTESIAN_POINT('Ctrl Pts',(0.711993139355394,1.,-1.64752408832016));
#30482=CARTESIAN_POINT('Ctrl Pts',(0.719585433804282,-1.,-1.6647288055568));
#30483=CARTESIAN_POINT('Ctrl Pts',(0.719585433804282,1.,-1.6647288055568));
#30484=CARTESIAN_POINT('Ctrl Pts',(0.726235967997433,-1.,-1.67996158455503));
#30485=CARTESIAN_POINT('Ctrl Pts',(0.726235967997433,1.,-1.67996158455503));
#30486=CARTESIAN_POINT('Ctrl Pts',(0.731963238697195,-1.,-1.69326921975743));
#30487=CARTESIAN_POINT('Ctrl Pts',(0.731963238697195,1.,-1.69326921975743));
#30488=CARTESIAN_POINT('Ctrl Pts',(0.736799665724771,-1.,-1.70473309006121));
#30489=CARTESIAN_POINT('Ctrl Pts',(0.736799665724771,1.,-1.70473309006121));
#30490=CARTESIAN_POINT('Ctrl Pts',(0.740795162032087,-1.,-1.71447789751927));
#30491=CARTESIAN_POINT('Ctrl Pts',(0.740795162032087,1.,-1.71447789751927));
#30492=CARTESIAN_POINT('Ctrl Pts',(0.744021445433764,-1.,-1.7226822991693));
#30493=CARTESIAN_POINT('Ctrl Pts',(0.744021445433764,1.,-1.7226822991693));
#30494=CARTESIAN_POINT('Ctrl Pts',(0.746574710096436,-1.,-1.72958533647399));
#30495=CARTESIAN_POINT('Ctrl Pts',(0.746574710096436,1.,-1.72958533647399));
#30496=CARTESIAN_POINT('Ctrl Pts',(0.748582462954854,-1.,-1.73550351679848));
#30497=CARTESIAN_POINT('Ctrl Pts',(0.748582462954854,1.,-1.73550351679848));
#30498=CARTESIAN_POINT('Ctrl Pts',(0.75019343597954,-1.,-1.74080458266705));
#30499=CARTESIAN_POINT('Ctrl Pts',(0.75019343597954,1.,-1.74080458266705));
#30500=CARTESIAN_POINT('Ctrl Pts',(0.751555614163629,-1.,-1.74585086852298));
#30501=CARTESIAN_POINT('Ctrl Pts',(0.751555614163629,1.,-1.74585086852298));
#30502=CARTESIAN_POINT('Ctrl Pts',(0.752797683531377,-1.,-1.75095139468809));
#30503=CARTESIAN_POINT('Ctrl Pts',(0.752797683531377,1.,-1.75095139468809));
#30504=CARTESIAN_POINT('Ctrl Pts',(0.75400925402848,-1.,-1.75631083600175));
#30505=CARTESIAN_POINT('Ctrl Pts',(0.75400925402848,1.,-1.75631083600175));
#30506=CARTESIAN_POINT('Ctrl Pts',(0.755220979975262,-1.,-1.7619781724032));
#30507=CARTESIAN_POINT('Ctrl Pts',(0.755220979975262,1.,-1.7619781724032));
#30508=CARTESIAN_POINT('Ctrl Pts',(0.756421896028403,-1.,-1.76789396003141));
#30509=CARTESIAN_POINT('Ctrl Pts',(0.756421896028403,1.,-1.76789396003141));
#30510=CARTESIAN_POINT('Ctrl Pts',(0.757578264077238,-1.,-1.77394167108342));
#30511=CARTESIAN_POINT('Ctrl Pts',(0.757578264077238,1.,-1.77394167108342));
#30512=CARTESIAN_POINT('Ctrl Pts',(0.75865062667738,-1.,-1.77999411220912));
#30513=CARTESIAN_POINT('Ctrl Pts',(0.75865062667738,1.,-1.77999411220912));
#30514=CARTESIAN_POINT('Ctrl Pts',(0.759614401109868,-1.,-1.78596964884527));
#30515=CARTESIAN_POINT('Ctrl Pts',(0.759614401109868,1.,-1.78596964884527));
#30516=CARTESIAN_POINT('Ctrl Pts',(0.760469555880425,-1.,-1.79185815610802));
#30517=CARTESIAN_POINT('Ctrl Pts',(0.760469555880425,1.,-1.79185815610802));
#30518=CARTESIAN_POINT('Ctrl Pts',(0.761229695230359,-1.,-1.79768986997735));
#30519=CARTESIAN_POINT('Ctrl Pts',(0.761229695230359,1.,-1.79768986997735));
#30520=CARTESIAN_POINT('Ctrl Pts',(0.761915336443515,-1.,-1.80351583877334));
#30521=CARTESIAN_POINT('Ctrl Pts',(0.761915336443515,1.,-1.80351583877334));
#30522=CARTESIAN_POINT('Ctrl Pts',(0.762546129464036,-1.,-1.80938551463989));
#30523=CARTESIAN_POINT('Ctrl Pts',(0.762546129464036,1.,-1.80938551463989));
#30524=CARTESIAN_POINT('Ctrl Pts',(0.763132003836783,-1.,-1.81532118405566));
#30525=CARTESIAN_POINT('Ctrl Pts',(0.763132003836783,1.,-1.81532118405566));
#30526=CARTESIAN_POINT('Ctrl Pts',(0.763673465462854,-1.,-1.82131873145297));
#30527=CARTESIAN_POINT('Ctrl Pts',(0.763673465462854,1.,-1.82131873145297));
#30528=CARTESIAN_POINT('Ctrl Pts',(0.764165902606055,-1.,-1.8273599120008));
#30529=CARTESIAN_POINT('Ctrl Pts',(0.764165902606055,1.,-1.8273599120008));
#30530=CARTESIAN_POINT('Ctrl Pts',(0.764602549687845,-1.,-1.8334207722714));
#30531=CARTESIAN_POINT('Ctrl Pts',(0.764602549687845,1.,-1.8334207722714));
#30532=CARTESIAN_POINT('Ctrl Pts',(0.764978057881687,-1.,-1.83948181064823));
#30533=CARTESIAN_POINT('Ctrl Pts',(0.764978057881687,1.,-1.83948181064823));
#30534=CARTESIAN_POINT('Ctrl Pts',(0.765291664861971,-1.,-1.84553698875911));
#30535=CARTESIAN_POINT('Ctrl Pts',(0.765291664861971,1.,-1.84553698875911));
#30536=CARTESIAN_POINT('Ctrl Pts',(0.765545710619023,-1.,-1.85158945130054));
#30537=CARTESIAN_POINT('Ctrl Pts',(0.765545710619023,1.,-1.85158945130054));
#30538=CARTESIAN_POINT('Ctrl Pts',(0.765744212909305,-1.,-1.85764741390391));
#30539=CARTESIAN_POINT('Ctrl Pts',(0.765744212909305,1.,-1.85764741390391));
#30540=CARTESIAN_POINT('Ctrl Pts',(0.765891519092557,-1.,-1.86372027063315));
#30541=CARTESIAN_POINT('Ctrl Pts',(0.765891519092557,1.,-1.86372027063315));
#30542=CARTESIAN_POINT('Ctrl Pts',(0.765990708546111,-1.,-1.86981398314345));
#30543=CARTESIAN_POINT('Ctrl Pts',(0.765990708546111,1.,-1.86981398314345));
#30544=CARTESIAN_POINT('Ctrl Pts',(0.766042837036759,-1.,-1.87592888967886));
#30545=CARTESIAN_POINT('Ctrl Pts',(0.766042837036759,1.,-1.87592888967886));
#30546=CARTESIAN_POINT('Ctrl Pts',(0.766047794851868,-1.,-1.88206215302561));
#30547=CARTESIAN_POINT('Ctrl Pts',(0.766047794851868,1.,-1.88206215302561));
#30548=CARTESIAN_POINT('Ctrl Pts',(0.76600483706209,-1.,-1.88820926433409));
#30549=CARTESIAN_POINT('Ctrl Pts',(0.76600483706209,1.,-1.88820926433409));
#30550=CARTESIAN_POINT('Ctrl Pts',(0.765913193856979,-1.,-1.89436577771389));
#30551=CARTESIAN_POINT('Ctrl Pts',(0.765913193856979,1.,-1.89436577771389));
#30552=CARTESIAN_POINT('Ctrl Pts',(0.765772772593395,-1.,-1.90052930393599));
#30553=CARTESIAN_POINT('Ctrl Pts',(0.765772772593395,1.,-1.90052930393599));
#30554=CARTESIAN_POINT('Ctrl Pts',(0.765584196937936,-1.,-1.90669961402362));
#30555=CARTESIAN_POINT('Ctrl Pts',(0.765584196937936,1.,-1.90669961402362));
#30556=CARTESIAN_POINT('Ctrl Pts',(0.765348465884739,-1.,-1.91287765805174));
#30557=CARTESIAN_POINT('Ctrl Pts',(0.765348465884739,1.,-1.91287765805174));
#30558=CARTESIAN_POINT('Ctrl Pts',(0.765066729667095,-1.,-1.91906491634197));
#30559=CARTESIAN_POINT('Ctrl Pts',(0.765066729667095,1.,-1.91906491634197));
#30560=CARTESIAN_POINT('Ctrl Pts',(0.764740025488189,-1.,-1.92526263537041));
#30561=CARTESIAN_POINT('Ctrl Pts',(0.764740025488189,1.,-1.92526263537041));
#30562=CARTESIAN_POINT('Ctrl Pts',(0.764369010673889,-1.,-1.93147105496367));
#30563=CARTESIAN_POINT('Ctrl Pts',(0.764369010673889,1.,-1.93147105496367));
#30564=CARTESIAN_POINT('Ctrl Pts',(0.763954049121393,-1.,-1.93768964875867));
#30565=CARTESIAN_POINT('Ctrl Pts',(0.763954049121393,1.,-1.93768964875867));
#30566=CARTESIAN_POINT('Ctrl Pts',(0.76349533353858,-1.,-1.94391746617626));
#30567=CARTESIAN_POINT('Ctrl Pts',(0.76349533353858,1.,-1.94391746617626));
#30568=CARTESIAN_POINT('Ctrl Pts',(0.762992990878774,-1.,-1.95015342590025));
#30569=CARTESIAN_POINT('Ctrl Pts',(0.762992990878774,1.,-1.95015342590025));
#30570=CARTESIAN_POINT('Ctrl Pts',(0.762447203806263,-1.,-1.95639665309893));
#30571=CARTESIAN_POINT('Ctrl Pts',(0.762447203806263,1.,-1.95639665309893));
#30572=CARTESIAN_POINT('Ctrl Pts',(0.761858300014575,-1.,-1.96264672744229));
#30573=CARTESIAN_POINT('Ctrl Pts',(0.761858300014575,1.,-1.96264672744229));
#30574=CARTESIAN_POINT('Ctrl Pts',(0.761226690483986,-1.,-1.96890351582545));
#30575=CARTESIAN_POINT('Ctrl Pts',(0.761226690483986,1.,-1.96890351582545));
#30576=CARTESIAN_POINT('Ctrl Pts',(0.760552825409855,-1.,-1.97516705321521));
#30577=CARTESIAN_POINT('Ctrl Pts',(0.760552825409855,1.,-1.97516705321521));
#30578=CARTESIAN_POINT('Ctrl Pts',(0.759837147452135,-1.,-1.98143741418156));
#30579=CARTESIAN_POINT('Ctrl Pts',(0.759837147452135,1.,-1.98143741418156));
#30580=CARTESIAN_POINT('Ctrl Pts',(0.759080037802242,-1.,-1.98771456680806));
#30581=CARTESIAN_POINT('Ctrl Pts',(0.759080037802242,1.,-1.98771456680806));
#30582=CARTESIAN_POINT('Ctrl Pts',(0.758281796766377,-1.,-1.9939983109871));
#30583=CARTESIAN_POINT('Ctrl Pts',(0.758281796766377,1.,-1.9939983109871));
#30584=CARTESIAN_POINT('Ctrl Pts',(0.757442676862341,-1.,-2.00028834739072));
#30585=CARTESIAN_POINT('Ctrl Pts',(0.757442676862341,1.,-2.00028834739072));
#30586=CARTESIAN_POINT('Ctrl Pts',(0.756562904646496,-1.,-2.00658431587682));
#30587=CARTESIAN_POINT('Ctrl Pts',(0.756562904646496,1.,-2.00658431587682));
#30588=CARTESIAN_POINT('Ctrl Pts',(0.7556427049581,-1.,-2.01288584328149));
#30589=CARTESIAN_POINT('Ctrl Pts',(0.7556427049581,1.,-2.01288584328149));
#30590=CARTESIAN_POINT('Ctrl Pts',(0.75468233072352,-1.,-2.01919259406003));
#30591=CARTESIAN_POINT('Ctrl Pts',(0.75468233072352,1.,-2.01919259406003));
#30592=CARTESIAN_POINT('Ctrl Pts',(0.753682061113765,-1.,-2.02550428623587));
#30593=CARTESIAN_POINT('Ctrl Pts',(0.753682061113765,1.,-2.02550428623587));
#30594=CARTESIAN_POINT('Ctrl Pts',(0.752642180488104,-1.,-2.03182068456467));
#30595=CARTESIAN_POINT('Ctrl Pts',(0.752642180488104,1.,-2.03182068456467));
#30596=CARTESIAN_POINT('Ctrl Pts',(0.751562963361383,-1.,-2.03814160092173));
#30597=CARTESIAN_POINT('Ctrl Pts',(0.751562963361383,1.,-2.03814160092173));
#30598=CARTESIAN_POINT('Ctrl Pts',(0.750444657874758,-1.,-2.04446689147754));
#30599=CARTESIAN_POINT('Ctrl Pts',(0.750444657874758,1.,-2.04446689147754));
#30600=CARTESIAN_POINT('Ctrl Pts',(0.749287468663053,-1.,-2.05079645591606));
#30601=CARTESIAN_POINT('Ctrl Pts',(0.749287468663053,1.,-2.05079645591606));
#30602=CARTESIAN_POINT('Ctrl Pts',(0.748091554181101,-1.,-2.05713023030263));
#30603=CARTESIAN_POINT('Ctrl Pts',(0.748091554181101,1.,-2.05713023030263));
#30604=CARTESIAN_POINT('Ctrl Pts',(0.747103932785504,-1.,-2.06220058927162));
#30605=CARTESIAN_POINT('Ctrl Pts',(0.747103932785504,1.,-2.06220058927162));
#30606=CARTESIAN_POINT('Ctrl Pts',(0.746345871542695,-1.,-2.06600523016401));
#30607=CARTESIAN_POINT('Ctrl Pts',(0.746345871542695,1.,-2.06600523016401));
#30608=CARTESIAN_POINT('Ctrl Pts',(0.74583279137781,-1.,-2.06854248895575));
#30609=CARTESIAN_POINT('Ctrl Pts',(0.74583279137781,1.,-2.06854248895575));
#30610=CARTESIAN_POINT('Ctrl Pts',(0.745574324794401,-1.,-2.0698113262342));
#30611=CARTESIAN_POINT('Ctrl Pts',(0.745574324794401,1.,-2.0698113262342));
#30612=CARTESIAN_POINT('',(0.693717979106306,1.,-1.60662857109684));
#30613=CARTESIAN_POINT('Ctrl Pts',(0.693717979106306,1.,-1.60662857109684));
#30614=CARTESIAN_POINT('Ctrl Pts',(0.695712097881194,1.,-1.61106790958151));
#30615=CARTESIAN_POINT('Ctrl Pts',(0.699605146405088,1.,-1.61974673472612));
#30616=CARTESIAN_POINT('Ctrl Pts',(0.705159151988319,1.,-1.63216541664676));
#30617=CARTESIAN_POINT('Ctrl Pts',(0.711993139355394,1.,-1.64752408832016));
#30618=CARTESIAN_POINT('Ctrl Pts',(0.719585433804282,1.,-1.6647288055568));
#30619=CARTESIAN_POINT('Ctrl Pts',(0.726235967997433,1.,-1.67996158455503));
#30620=CARTESIAN_POINT('Ctrl Pts',(0.731963238697195,1.,-1.69326921975743));
#30621=CARTESIAN_POINT('Ctrl Pts',(0.736799665724771,1.,-1.70473309006121));
#30622=CARTESIAN_POINT('Ctrl Pts',(0.740795162032087,1.,-1.71447789751927));
#30623=CARTESIAN_POINT('Ctrl Pts',(0.744021445433764,1.,-1.7226822991693));
#30624=CARTESIAN_POINT('Ctrl Pts',(0.746574710096436,1.,-1.72958533647399));
#30625=CARTESIAN_POINT('Ctrl Pts',(0.748582462954854,1.,-1.73550351679848));
#30626=CARTESIAN_POINT('Ctrl Pts',(0.75019343597954,1.,-1.74080458266705));
#30627=CARTESIAN_POINT('Ctrl Pts',(0.751555614163629,1.,-1.74585086852298));
#30628=CARTESIAN_POINT('Ctrl Pts',(0.752797683531377,1.,-1.75095139468809));
#30629=CARTESIAN_POINT('Ctrl Pts',(0.75400925402848,1.,-1.75631083600175));
#30630=CARTESIAN_POINT('Ctrl Pts',(0.755220979975262,1.,-1.7619781724032));
#30631=CARTESIAN_POINT('Ctrl Pts',(0.756421896028403,1.,-1.76789396003141));
#30632=CARTESIAN_POINT('Ctrl Pts',(0.757578264077238,1.,-1.77394167108342));
#30633=CARTESIAN_POINT('Ctrl Pts',(0.75865062667738,1.,-1.77999411220912));
#30634=CARTESIAN_POINT('Ctrl Pts',(0.759614401109868,1.,-1.78596964884527));
#30635=CARTESIAN_POINT('Ctrl Pts',(0.760469555880425,1.,-1.79185815610802));
#30636=CARTESIAN_POINT('Ctrl Pts',(0.761229695230359,1.,-1.79768986997735));
#30637=CARTESIAN_POINT('Ctrl Pts',(0.761915336443515,1.,-1.80351583877334));
#30638=CARTESIAN_POINT('Ctrl Pts',(0.762546129464036,1.,-1.80938551463989));
#30639=CARTESIAN_POINT('Ctrl Pts',(0.763132003836783,1.,-1.81532118405566));
#30640=CARTESIAN_POINT('Ctrl Pts',(0.763673465462854,1.,-1.82131873145297));
#30641=CARTESIAN_POINT('Ctrl Pts',(0.764165902606055,1.,-1.8273599120008));
#30642=CARTESIAN_POINT('Ctrl Pts',(0.764602549687845,1.,-1.8334207722714));
#30643=CARTESIAN_POINT('Ctrl Pts',(0.764978057881687,1.,-1.83948181064823));
#30644=CARTESIAN_POINT('Ctrl Pts',(0.765291664861971,1.,-1.84553698875911));
#30645=CARTESIAN_POINT('Ctrl Pts',(0.765545710619023,1.,-1.85158945130054));
#30646=CARTESIAN_POINT('Ctrl Pts',(0.765744212909305,1.,-1.85764741390391));
#30647=CARTESIAN_POINT('Ctrl Pts',(0.765891519092557,1.,-1.86372027063315));
#30648=CARTESIAN_POINT('Ctrl Pts',(0.765990708546111,1.,-1.86981398314345));
#30649=CARTESIAN_POINT('Ctrl Pts',(0.766042837036759,1.,-1.87592888967886));
#30650=CARTESIAN_POINT('Ctrl Pts',(0.766047794851868,1.,-1.88206215302561));
#30651=CARTESIAN_POINT('Ctrl Pts',(0.76600483706209,1.,-1.88820926433409));
#30652=CARTESIAN_POINT('Ctrl Pts',(0.765913193856979,1.,-1.89436577771389));
#30653=CARTESIAN_POINT('Ctrl Pts',(0.765772772593395,1.,-1.90052930393599));
#30654=CARTESIAN_POINT('Ctrl Pts',(0.765584196937936,1.,-1.90669961402362));
#30655=CARTESIAN_POINT('Ctrl Pts',(0.765348465884739,1.,-1.91287765805174));
#30656=CARTESIAN_POINT('Ctrl Pts',(0.765066729667095,1.,-1.91906491634197));
#30657=CARTESIAN_POINT('Ctrl Pts',(0.764740025488189,1.,-1.92526263537041));
#30658=CARTESIAN_POINT('Ctrl Pts',(0.764369010673889,1.,-1.93147105496367));
#30659=CARTESIAN_POINT('Ctrl Pts',(0.763954049121393,1.,-1.93768964875867));
#30660=CARTESIAN_POINT('Ctrl Pts',(0.76349533353858,1.,-1.94391746617626));
#30661=CARTESIAN_POINT('Ctrl Pts',(0.762992990878774,1.,-1.95015342590025));
#30662=CARTESIAN_POINT('Ctrl Pts',(0.762447203806263,1.,-1.95639665309893));
#30663=CARTESIAN_POINT('Ctrl Pts',(0.761858300014575,1.,-1.96264672744229));
#30664=CARTESIAN_POINT('Ctrl Pts',(0.761226690483986,1.,-1.96890351582545));
#30665=CARTESIAN_POINT('Ctrl Pts',(0.760552825409855,1.,-1.97516705321521));
#30666=CARTESIAN_POINT('Ctrl Pts',(0.759837147452135,1.,-1.98143741418156));
#30667=CARTESIAN_POINT('Ctrl Pts',(0.759080037802242,1.,-1.98771456680806));
#30668=CARTESIAN_POINT('Ctrl Pts',(0.758281796766377,1.,-1.9939983109871));
#30669=CARTESIAN_POINT('Ctrl Pts',(0.757442676862341,1.,-2.00028834739072));
#30670=CARTESIAN_POINT('Ctrl Pts',(0.756562904646496,1.,-2.00658431587682));
#30671=CARTESIAN_POINT('Ctrl Pts',(0.7556427049581,1.,-2.01288584328149));
#30672=CARTESIAN_POINT('Ctrl Pts',(0.75468233072352,1.,-2.01919259406003));
#30673=CARTESIAN_POINT('Ctrl Pts',(0.753682061113765,1.,-2.02550428623587));
#30674=CARTESIAN_POINT('Ctrl Pts',(0.752642180488104,1.,-2.03182068456467));
#30675=CARTESIAN_POINT('Ctrl Pts',(0.751562963361383,1.,-2.03814160092173));
#30676=CARTESIAN_POINT('Ctrl Pts',(0.750444657874758,1.,-2.04446689147754));
#30677=CARTESIAN_POINT('Ctrl Pts',(0.749287468663053,1.,-2.05079645591606));
#30678=CARTESIAN_POINT('Ctrl Pts',(0.748091554181101,1.,-2.05713023030263));
#30679=CARTESIAN_POINT('Ctrl Pts',(0.747103932785504,1.,-2.06220058927162));
#30680=CARTESIAN_POINT('Ctrl Pts',(0.746345871542695,1.,-2.06600523016401));
#30681=CARTESIAN_POINT('Ctrl Pts',(0.74583279137781,1.,-2.06854248895575));
#30682=CARTESIAN_POINT('Ctrl Pts',(0.745574324794401,1.,-2.0698113262342));
#30683=CARTESIAN_POINT('',(0.693717979106306,0.,-1.60662857109684));
#30684=CARTESIAN_POINT('Origin',(0.,0.,0.));
#30685=CARTESIAN_POINT('',(0.892032620296855,1.,-1.5055822144029));
#30686=CARTESIAN_POINT('Origin',(0.,1.,0.));
#30687=CARTESIAN_POINT('',(0.892032620296855,0.,-1.5055822144029));
#30688=CARTESIAN_POINT('Ctrl Pts',(1.23627494547115,-1.,-1.81978687191668));
#30689=CARTESIAN_POINT('Ctrl Pts',(1.23627494547115,1.,-1.81978687191668));
#30690=CARTESIAN_POINT('Ctrl Pts',(1.23509651170476,-1.,-1.81925017193666));
#30691=CARTESIAN_POINT('Ctrl Pts',(1.23509651170476,1.,-1.81925017193666));
#30692=CARTESIAN_POINT('Ctrl Pts',(1.2327422452705,-1.,-1.81817389921279));
#30693=CARTESIAN_POINT('Ctrl Pts',(1.2327422452705,1.,-1.81817389921279));
#30694=CARTESIAN_POINT('Ctrl Pts',(1.2292186489137,-1.,-1.8165508718364));
#30695=CARTESIAN_POINT('Ctrl Pts',(1.2292186489137,1.,-1.8165508718364));
#30696=CARTESIAN_POINT('Ctrl Pts',(1.2245361330495,-1.,-1.81436959210434));
#30697=CARTESIAN_POINT('Ctrl Pts',(1.2245361330495,1.,-1.81436959210434));
#30698=CARTESIAN_POINT('Ctrl Pts',(1.21870906103557,-1.,-1.81161420806656));
#30699=CARTESIAN_POINT('Ctrl Pts',(1.21870906103557,1.,-1.81161420806656));
#30700=CARTESIAN_POINT('Ctrl Pts',(1.21290815708314,-1.,-1.80882996917129));
#30701=CARTESIAN_POINT('Ctrl Pts',(1.21290815708314,1.,-1.80882996917129));
#30702=CARTESIAN_POINT('Ctrl Pts',(1.20713356605475,-1.,-1.80601678480707));
#30703=CARTESIAN_POINT('Ctrl Pts',(1.20713356605475,1.,-1.80601678480707));
#30704=CARTESIAN_POINT('Ctrl Pts',(1.20138548938974,-1.,-1.80317454838603));
#30705=CARTESIAN_POINT('Ctrl Pts',(1.20138548938974,1.,-1.80317454838603));
#30706=CARTESIAN_POINT('Ctrl Pts',(1.19566418930242,-1.,-1.80030314369879));
#30707=CARTESIAN_POINT('Ctrl Pts',(1.19566418930242,1.,-1.80030314369879));
#30708=CARTESIAN_POINT('Ctrl Pts',(1.18996997934445,-1.,-1.79740245923478));
#30709=CARTESIAN_POINT('Ctrl Pts',(1.18996997934445,1.,-1.79740245923478));
#30710=CARTESIAN_POINT('Ctrl Pts',(1.18430321697432,-1.,-1.79447240321515));
#30711=CARTESIAN_POINT('Ctrl Pts',(1.18430321697432,1.,-1.79447240321515));
#30712=CARTESIAN_POINT('Ctrl Pts',(1.17866429440809,-1.,-1.79151291552689));
#30713=CARTESIAN_POINT('Ctrl Pts',(1.17866429440809,1.,-1.79151291552689));
#30714=CARTESIAN_POINT('Ctrl Pts',(1.17305363177328,-1.,-1.78852398877617));
#30715=CARTESIAN_POINT('Ctrl Pts',(1.17305363177328,1.,-1.78852398877617));
#30716=CARTESIAN_POINT('Ctrl Pts',(1.16747166312303,-1.,-1.78550566040443));
#30717=CARTESIAN_POINT('Ctrl Pts',(1.16747166312303,1.,-1.78550566040443));
#30718=CARTESIAN_POINT('Ctrl Pts',(1.16191881298499,-1.,-1.78245795881009));
#30719=CARTESIAN_POINT('Ctrl Pts',(1.16191881298499,1.,-1.78245795881009));
#30720=CARTESIAN_POINT('Ctrl Pts',(1.15639547194698,-1.,-1.77938085564275));
#30721=CARTESIAN_POINT('Ctrl Pts',(1.15639547194698,1.,-1.77938085564275));
#30722=CARTESIAN_POINT('Ctrl Pts',(1.15090197841514,-1.,-1.7762742255701));
#30723=CARTESIAN_POINT('Ctrl Pts',(1.15090197841514,1.,-1.7762742255701));
#30724=CARTESIAN_POINT('Ctrl Pts',(1.1454385822692,-1.,-1.77313777896194));
#30725=CARTESIAN_POINT('Ctrl Pts',(1.1454385822692,1.,-1.77313777896194));
#30726=CARTESIAN_POINT('Ctrl Pts',(1.14000548336975,-1.,-1.76997111386769));
#30727=CARTESIAN_POINT('Ctrl Pts',(1.14000548336975,1.,-1.76997111386769));
#30728=CARTESIAN_POINT('Ctrl Pts',(1.1346029180462,-1.,-1.76677384551862));
#30729=CARTESIAN_POINT('Ctrl Pts',(1.1346029180462,1.,-1.76677384551862));
#30730=CARTESIAN_POINT('Ctrl Pts',(1.12923123555075,-1.,-1.7635457196617));
#30731=CARTESIAN_POINT('Ctrl Pts',(1.12923123555075,1.,-1.7635457196617));
#30732=CARTESIAN_POINT('Ctrl Pts',(1.12389096855086,-1.,-1.76028671825096));
#30733=CARTESIAN_POINT('Ctrl Pts',(1.12389096855086,1.,-1.76028671825096));
#30734=CARTESIAN_POINT('Ctrl Pts',(1.11858293216763,-1.,-1.75699720772105));
#30735=CARTESIAN_POINT('Ctrl Pts',(1.11858293216763,1.,-1.75699720772105));
#30736=CARTESIAN_POINT('Ctrl Pts',(1.11330807582551,-1.,-1.7536777209463));
#30737=CARTESIAN_POINT('Ctrl Pts',(1.11330807582551,1.,-1.7536777209463));
#30738=CARTESIAN_POINT('Ctrl Pts',(1.10806728183007,-1.,-1.7503286607592));
#30739=CARTESIAN_POINT('Ctrl Pts',(1.10806728183007,1.,-1.7503286607592));
#30740=CARTESIAN_POINT('Ctrl Pts',(1.10286118991143,-1.,-1.74695004214923));
#30741=CARTESIAN_POINT('Ctrl Pts',(1.10286118991143,1.,-1.74695004214923));
#30742=CARTESIAN_POINT('Ctrl Pts',(1.09768999241225,-1.,-1.74354119236208));
#30743=CARTESIAN_POINT('Ctrl Pts',(1.09768999241225,1.,-1.74354119236208));
#30744=CARTESIAN_POINT('Ctrl Pts',(1.09255329056493,-1.,-1.74010053962247));
#30745=CARTESIAN_POINT('Ctrl Pts',(1.09255329056493,1.,-1.74010053962247));
#30746=CARTESIAN_POINT('Ctrl Pts',(1.08745056285427,-1.,-1.73662628326091));
#30747=CARTESIAN_POINT('Ctrl Pts',(1.08745056285427,1.,-1.73662628326091));
#30748=CARTESIAN_POINT('Ctrl Pts',(1.08238162784749,-1.,-1.73311705663407));
#30749=CARTESIAN_POINT('Ctrl Pts',(1.08238162784749,1.,-1.73311705663407));
#30750=CARTESIAN_POINT('Ctrl Pts',(1.0773470373727,-1.,-1.72957248977424));
#30751=CARTESIAN_POINT('Ctrl Pts',(1.0773470373727,1.,-1.72957248977424));
#30752=CARTESIAN_POINT('Ctrl Pts',(1.07234866990252,-1.,-1.72599406198488));
#30753=CARTESIAN_POINT('Ctrl Pts',(1.07234866990252,1.,-1.72599406198488));
#30754=CARTESIAN_POINT('Ctrl Pts',(1.06738966975462,-1.,-1.72238500928453));
#30755=CARTESIAN_POINT('Ctrl Pts',(1.06738966975462,1.,-1.72238500928453));
#30756=CARTESIAN_POINT('Ctrl Pts',(1.06247324680647,-1.,-1.71874858456904));
#30757=CARTESIAN_POINT('Ctrl Pts',(1.06247324680647,1.,-1.71874858456904));
#30758=CARTESIAN_POINT('Ctrl Pts',(1.05760163192479,-1.,-1.7150865442702));
#30759=CARTESIAN_POINT('Ctrl Pts',(1.05760163192479,1.,-1.7150865442702));
#30760=CARTESIAN_POINT('Ctrl Pts',(1.05277517202855,-1.,-1.71139783543989));
#30761=CARTESIAN_POINT('Ctrl Pts',(1.05277517202855,1.,-1.71139783543989));
#30762=CARTESIAN_POINT('Ctrl Pts',(1.04799085404995,-1.,-1.70767646263649));
#30763=CARTESIAN_POINT('Ctrl Pts',(1.04799085404995,1.,-1.70767646263649));
#30764=CARTESIAN_POINT('Ctrl Pts',(1.04324363334554,-1.,-1.70391338707982));
#30765=CARTESIAN_POINT('Ctrl Pts',(1.04324363334554,1.,-1.70391338707982));
#30766=CARTESIAN_POINT('Ctrl Pts',(1.03852922490789,-1.,-1.70010052930962));
#30767=CARTESIAN_POINT('Ctrl Pts',(1.03852922490789,1.,-1.70010052930962));
#30768=CARTESIAN_POINT('Ctrl Pts',(1.03384646003588,-1.,-1.69623414782771));
#30769=CARTESIAN_POINT('Ctrl Pts',(1.03384646003588,1.,-1.69623414782771));
#30770=CARTESIAN_POINT('Ctrl Pts',(1.02919977579147,-1.,-1.69231840863458));
#30771=CARTESIAN_POINT('Ctrl Pts',(1.02919977579147,1.,-1.69231840863458));
#30772=CARTESIAN_POINT('Ctrl Pts',(1.02460180535255,-1.,-1.68836910178447));
#30773=CARTESIAN_POINT('Ctrl Pts',(1.02460180535255,1.,-1.68836910178447));
#30774=CARTESIAN_POINT('Ctrl Pts',(1.02006795074201,-1.,-1.68440578021706));
#30775=CARTESIAN_POINT('Ctrl Pts',(1.02006795074201,1.,-1.68440578021706));
#30776=CARTESIAN_POINT('Ctrl Pts',(1.01561026162773,-1.,-1.68044289894798));
#30777=CARTESIAN_POINT('Ctrl Pts',(1.01561026162773,1.,-1.68044289894798));
#30778=CARTESIAN_POINT('Ctrl Pts',(1.01123236493511,-1.,-1.67648246776464));
#30779=CARTESIAN_POINT('Ctrl Pts',(1.01123236493511,1.,-1.67648246776464));
#30780=CARTESIAN_POINT('Ctrl Pts',(1.00692206696414,-1.,-1.67250335383293));
#30781=CARTESIAN_POINT('Ctrl Pts',(1.00692206696414,1.,-1.67250335383293));
#30782=CARTESIAN_POINT('Ctrl Pts',(1.00265091003727,-1.,-1.66846059277303));
#30783=CARTESIAN_POINT('Ctrl Pts',(1.00265091003727,1.,-1.66846059277303));
#30784=CARTESIAN_POINT('Ctrl Pts',(0.998389654952757,-1.,-1.66430758030376));
#30785=CARTESIAN_POINT('Ctrl Pts',(0.998389654952757,1.,-1.66430758030376));
#30786=CARTESIAN_POINT('Ctrl Pts',(0.994121836661305,-1.,-1.66001553809947));
#30787=CARTESIAN_POINT('Ctrl Pts',(0.994121836661305,1.,-1.66001553809947));
#30788=CARTESIAN_POINT('Ctrl Pts',(0.989855627854164,-1.,-1.65559044289699));
#30789=CARTESIAN_POINT('Ctrl Pts',(0.989855627854164,1.,-1.65559044289699));
#30790=CARTESIAN_POINT('Ctrl Pts',(0.98564262292082,-1.,-1.65110016612638));
#30791=CARTESIAN_POINT('Ctrl Pts',(0.98564262292082,1.,-1.65110016612638));
#30792=CARTESIAN_POINT('Ctrl Pts',(0.981562530939489,-1.,-1.64665139190656));
#30793=CARTESIAN_POINT('Ctrl Pts',(0.981562530939489,1.,-1.64665139190656));
#30794=CARTESIAN_POINT('Ctrl Pts',(0.977689794119416,-1.,-1.64233990826687));
#30795=CARTESIAN_POINT('Ctrl Pts',(0.977689794119416,1.,-1.64233990826687));
#30796=CARTESIAN_POINT('Ctrl Pts',(0.974066058287418,-1.,-1.63820952658144));
#30797=CARTESIAN_POINT('Ctrl Pts',(0.974066058287418,1.,-1.63820952658144));
#30798=CARTESIAN_POINT('Ctrl Pts',(0.970669715997509,-1.,-1.63420665729798));
#30799=CARTESIAN_POINT('Ctrl Pts',(0.970669715997509,1.,-1.63420665729798));
#30800=CARTESIAN_POINT('Ctrl Pts',(0.967387853230345,-1.,-1.63013849959462));
#30801=CARTESIAN_POINT('Ctrl Pts',(0.967387853230345,1.,-1.63013849959462));
#30802=CARTESIAN_POINT('Ctrl Pts',(0.964046107040535,-1.,-1.62571930670187));
#30803=CARTESIAN_POINT('Ctrl Pts',(0.964046107040535,1.,-1.62571930670187));
#30804=CARTESIAN_POINT('Ctrl Pts',(0.960438326101728,-1.,-1.62061638140221));
#30805=CARTESIAN_POINT('Ctrl Pts',(0.960438326101728,1.,-1.62061638140221));
#30806=CARTESIAN_POINT('Ctrl Pts',(0.95635442292067,-1.,-1.61449324337085));
#30807=CARTESIAN_POINT('Ctrl Pts',(0.95635442292067,1.,-1.61449324337085));
#30808=CARTESIAN_POINT('Ctrl Pts',(0.951613284356035,-1.,-1.60706069896936));
#30809=CARTESIAN_POINT('Ctrl Pts',(0.951613284356035,1.,-1.60706069896936));
#30810=CARTESIAN_POINT('Ctrl Pts',(0.946078063315257,-1.,-1.59810042043673));
#30811=CARTESIAN_POINT('Ctrl Pts',(0.946078063315257,1.,-1.59810042043673));
#30812=CARTESIAN_POINT('Ctrl Pts',(0.939646377893399,-1.,-1.58744937487176));
#30813=CARTESIAN_POINT('Ctrl Pts',(0.939646377893399,1.,-1.58744937487176));
#30814=CARTESIAN_POINT('Ctrl Pts',(0.932246680108685,-1.,-1.57499388382243));
#30815=CARTESIAN_POINT('Ctrl Pts',(0.932246680108685,1.,-1.57499388382243));
#30816=CARTESIAN_POINT('Ctrl Pts',(0.923832188944341,-1.,-1.56065988578893));
#30817=CARTESIAN_POINT('Ctrl Pts',(0.923832188944341,1.,-1.56065988578893));
#30818=CARTESIAN_POINT('Ctrl Pts',(0.914375919026456,-1.,-1.54440491149498));
#30819=CARTESIAN_POINT('Ctrl Pts',(0.914375919026456,1.,-1.54440491149498));
#30820=CARTESIAN_POINT('Ctrl Pts',(0.905967409625651,-1.,-1.52984849887993));
#30821=CARTESIAN_POINT('Ctrl Pts',(0.905967409625651,1.,-1.52984849887993));
#30822=CARTESIAN_POINT('Ctrl Pts',(0.89918504748351,-1.,-1.51805569590094));
#30823=CARTESIAN_POINT('Ctrl Pts',(0.89918504748351,1.,-1.51805569590094));
#30824=CARTESIAN_POINT('Ctrl Pts',(0.894452006964543,-1.,-1.50980486806688));
#30825=CARTESIAN_POINT('Ctrl Pts',(0.894452006964543,1.,-1.50980486806688));
#30826=CARTESIAN_POINT('Ctrl Pts',(0.892032620296855,-1.,-1.5055822144029));
#30827=CARTESIAN_POINT('Ctrl Pts',(0.892032620296855,1.,-1.5055822144029));
#30828=CARTESIAN_POINT('',(1.23627494547115,1.,-1.81978687191668));
#30829=CARTESIAN_POINT('Ctrl Pts',(1.23627494547115,1.,-1.81978687191668));
#30830=CARTESIAN_POINT('Ctrl Pts',(1.23509651170476,1.,-1.81925017193666));
#30831=CARTESIAN_POINT('Ctrl Pts',(1.2327422452705,1.,-1.81817389921279));
#30832=CARTESIAN_POINT('Ctrl Pts',(1.2292186489137,1.,-1.8165508718364));
#30833=CARTESIAN_POINT('Ctrl Pts',(1.2245361330495,1.,-1.81436959210434));
#30834=CARTESIAN_POINT('Ctrl Pts',(1.21870906103557,1.,-1.81161420806656));
#30835=CARTESIAN_POINT('Ctrl Pts',(1.21290815708314,1.,-1.80882996917129));
#30836=CARTESIAN_POINT('Ctrl Pts',(1.20713356605475,1.,-1.80601678480707));
#30837=CARTESIAN_POINT('Ctrl Pts',(1.20138548938974,1.,-1.80317454838603));
#30838=CARTESIAN_POINT('Ctrl Pts',(1.19566418930242,1.,-1.80030314369879));
#30839=CARTESIAN_POINT('Ctrl Pts',(1.18996997934445,1.,-1.79740245923478));
#30840=CARTESIAN_POINT('Ctrl Pts',(1.18430321697432,1.,-1.79447240321515));
#30841=CARTESIAN_POINT('Ctrl Pts',(1.17866429440809,1.,-1.79151291552689));
#30842=CARTESIAN_POINT('Ctrl Pts',(1.17305363177328,1.,-1.78852398877617));
#30843=CARTESIAN_POINT('Ctrl Pts',(1.16747166312303,1.,-1.78550566040443));
#30844=CARTESIAN_POINT('Ctrl Pts',(1.16191881298499,1.,-1.78245795881009));
#30845=CARTESIAN_POINT('Ctrl Pts',(1.15639547194698,1.,-1.77938085564275));
#30846=CARTESIAN_POINT('Ctrl Pts',(1.15090197841514,1.,-1.7762742255701));
#30847=CARTESIAN_POINT('Ctrl Pts',(1.1454385822692,1.,-1.77313777896194));
#30848=CARTESIAN_POINT('Ctrl Pts',(1.14000548336975,1.,-1.76997111386769));
#30849=CARTESIAN_POINT('Ctrl Pts',(1.1346029180462,1.,-1.76677384551862));
#30850=CARTESIAN_POINT('Ctrl Pts',(1.12923123555075,1.,-1.7635457196617));
#30851=CARTESIAN_POINT('Ctrl Pts',(1.12389096855086,1.,-1.76028671825096));
#30852=CARTESIAN_POINT('Ctrl Pts',(1.11858293216763,1.,-1.75699720772105));
#30853=CARTESIAN_POINT('Ctrl Pts',(1.11330807582551,1.,-1.7536777209463));
#30854=CARTESIAN_POINT('Ctrl Pts',(1.10806728183007,1.,-1.7503286607592));
#30855=CARTESIAN_POINT('Ctrl Pts',(1.10286118991143,1.,-1.74695004214923));
#30856=CARTESIAN_POINT('Ctrl Pts',(1.09768999241225,1.,-1.74354119236208));
#30857=CARTESIAN_POINT('Ctrl Pts',(1.09255329056493,1.,-1.74010053962247));
#30858=CARTESIAN_POINT('Ctrl Pts',(1.08745056285427,1.,-1.73662628326091));
#30859=CARTESIAN_POINT('Ctrl Pts',(1.08238162784749,1.,-1.73311705663407));
#30860=CARTESIAN_POINT('Ctrl Pts',(1.0773470373727,1.,-1.72957248977424));
#30861=CARTESIAN_POINT('Ctrl Pts',(1.07234866990252,1.,-1.72599406198488));
#30862=CARTESIAN_POINT('Ctrl Pts',(1.06738966975462,1.,-1.72238500928453));
#30863=CARTESIAN_POINT('Ctrl Pts',(1.06247324680647,1.,-1.71874858456904));
#30864=CARTESIAN_POINT('Ctrl Pts',(1.05760163192479,1.,-1.7150865442702));
#30865=CARTESIAN_POINT('Ctrl Pts',(1.05277517202855,1.,-1.71139783543989));
#30866=CARTESIAN_POINT('Ctrl Pts',(1.04799085404995,1.,-1.70767646263649));
#30867=CARTESIAN_POINT('Ctrl Pts',(1.04324363334554,1.,-1.70391338707982));
#30868=CARTESIAN_POINT('Ctrl Pts',(1.03852922490789,1.,-1.70010052930962));
#30869=CARTESIAN_POINT('Ctrl Pts',(1.03384646003588,1.,-1.69623414782771));
#30870=CARTESIAN_POINT('Ctrl Pts',(1.02919977579147,1.,-1.69231840863458));
#30871=CARTESIAN_POINT('Ctrl Pts',(1.02460180535255,1.,-1.68836910178447));
#30872=CARTESIAN_POINT('Ctrl Pts',(1.02006795074201,1.,-1.68440578021706));
#30873=CARTESIAN_POINT('Ctrl Pts',(1.01561026162773,1.,-1.68044289894798));
#30874=CARTESIAN_POINT('Ctrl Pts',(1.01123236493511,1.,-1.67648246776464));
#30875=CARTESIAN_POINT('Ctrl Pts',(1.00692206696414,1.,-1.67250335383293));
#30876=CARTESIAN_POINT('Ctrl Pts',(1.00265091003727,1.,-1.66846059277303));
#30877=CARTESIAN_POINT('Ctrl Pts',(0.998389654952757,1.,-1.66430758030376));
#30878=CARTESIAN_POINT('Ctrl Pts',(0.994121836661305,1.,-1.66001553809947));
#30879=CARTESIAN_POINT('Ctrl Pts',(0.989855627854164,1.,-1.65559044289699));
#30880=CARTESIAN_POINT('Ctrl Pts',(0.98564262292082,1.,-1.65110016612638));
#30881=CARTESIAN_POINT('Ctrl Pts',(0.981562530939489,1.,-1.64665139190656));
#30882=CARTESIAN_POINT('Ctrl Pts',(0.977689794119416,1.,-1.64233990826687));
#30883=CARTESIAN_POINT('Ctrl Pts',(0.974066058287418,1.,-1.63820952658144));
#30884=CARTESIAN_POINT('Ctrl Pts',(0.970669715997509,1.,-1.63420665729798));
#30885=CARTESIAN_POINT('Ctrl Pts',(0.967387853230345,1.,-1.63013849959462));
#30886=CARTESIAN_POINT('Ctrl Pts',(0.964046107040535,1.,-1.62571930670187));
#30887=CARTESIAN_POINT('Ctrl Pts',(0.960438326101728,1.,-1.62061638140221));
#30888=CARTESIAN_POINT('Ctrl Pts',(0.95635442292067,1.,-1.61449324337085));
#30889=CARTESIAN_POINT('Ctrl Pts',(0.951613284356035,1.,-1.60706069896936));
#30890=CARTESIAN_POINT('Ctrl Pts',(0.946078063315257,1.,-1.59810042043673));
#30891=CARTESIAN_POINT('Ctrl Pts',(0.939646377893399,1.,-1.58744937487176));
#30892=CARTESIAN_POINT('Ctrl Pts',(0.932246680108685,1.,-1.57499388382243));
#30893=CARTESIAN_POINT('Ctrl Pts',(0.923832188944341,1.,-1.56065988578893));
#30894=CARTESIAN_POINT('Ctrl Pts',(0.914375919026456,1.,-1.54440491149498));
#30895=CARTESIAN_POINT('Ctrl Pts',(0.905967409625651,1.,-1.52984849887993));
#30896=CARTESIAN_POINT('Ctrl Pts',(0.89918504748351,1.,-1.51805569590094));
#30897=CARTESIAN_POINT('Ctrl Pts',(0.894452006964543,1.,-1.50980486806688));
#30898=CARTESIAN_POINT('Ctrl Pts',(0.892032620296855,1.,-1.5055822144029));
#30899=CARTESIAN_POINT('',(1.23627494547115,0.,-1.81978687191668));
#30900=CARTESIAN_POINT('Origin',(1.34869019493419,0.,-1.73811241238545));
#30901=CARTESIAN_POINT('',(1.34869019493419,1.,-1.73811241238545));
#30902=CARTESIAN_POINT('',(1.23627494547115,1.,-1.81978687191668));
#30903=CARTESIAN_POINT('',(1.34869019493419,0.,-1.73811241238545));
#30904=CARTESIAN_POINT('Ctrl Pts',(1.15624053661742,-1.,-1.31362392696032));
#30905=CARTESIAN_POINT('Ctrl Pts',(1.15624053661742,1.,-1.31362392696032));
#30906=CARTESIAN_POINT('Ctrl Pts',(1.15950888730809,-1.,-1.31722977216397));
#30907=CARTESIAN_POINT('Ctrl Pts',(1.15950888730809,1.,-1.31722977216397));
#30908=CARTESIAN_POINT('Ctrl Pts',(1.16589330093588,-1.,-1.32428080721772));
#30909=CARTESIAN_POINT('Ctrl Pts',(1.16589330093588,1.,-1.32428080721772));
#30910=CARTESIAN_POINT('Ctrl Pts',(1.17501305789857,-1.,-1.33437539347008));
#30911=CARTESIAN_POINT('Ctrl Pts',(1.17501305789857,1.,-1.33437539347008));
#30912=CARTESIAN_POINT('Ctrl Pts',(1.18625865667441,-1.,-1.34687054001093));
#30913=CARTESIAN_POINT('Ctrl Pts',(1.18625865667441,1.,-1.34687054001093));
#30914=CARTESIAN_POINT('Ctrl Pts',(1.1987959077932,-1.,-1.36088705043885));
#30915=CARTESIAN_POINT('Ctrl Pts',(1.1987959077932,1.,-1.36088705043885));
#30916=CARTESIAN_POINT('Ctrl Pts',(1.20982812925645,-1.,-1.37331915607905));
#30917=CARTESIAN_POINT('Ctrl Pts',(1.20982812925645,1.,-1.37331915607905));
#30918=CARTESIAN_POINT('Ctrl Pts',(1.21938737280852,-1.,-1.38420564527715));
#30919=CARTESIAN_POINT('Ctrl Pts',(1.21938737280852,1.,-1.38420564527715));
#30920=CARTESIAN_POINT('Ctrl Pts',(1.22752961899387,-1.,-1.39361389568796));
#30921=CARTESIAN_POINT('Ctrl Pts',(1.22752961899387,1.,-1.39361389568796));
#30922=CARTESIAN_POINT('Ctrl Pts',(1.23434087290423,-1.,-1.40164708206106));
#30923=CARTESIAN_POINT('Ctrl Pts',(1.23434087290423,1.,-1.40164708206106));
#30924=CARTESIAN_POINT('Ctrl Pts',(1.23994455029534,-1.,-1.40845295531283));
#30925=CARTESIAN_POINT('Ctrl Pts',(1.23994455029534,1.,-1.40845295531283));
#30926=CARTESIAN_POINT('Ctrl Pts',(1.24450600513056,-1.,-1.41422913175179));
#30927=CARTESIAN_POINT('Ctrl Pts',(1.24450600513056,1.,-1.41422913175179));
#30928=CARTESIAN_POINT('Ctrl Pts',(1.24824430986571,-1.,-1.41923722596025));
#30929=CARTESIAN_POINT('Ctrl Pts',(1.24824430986571,1.,-1.41923722596025));
#30930=CARTESIAN_POINT('Ctrl Pts',(1.2514145557001,-1.,-1.42378102115575));
#30931=CARTESIAN_POINT('Ctrl Pts',(1.2514145557001,1.,-1.42378102115575));
#30932=CARTESIAN_POINT('Ctrl Pts',(1.25426945222639,-1.,-1.42815938799387));
#30933=CARTESIAN_POINT('Ctrl Pts',(1.25426945222639,1.,-1.42815938799387));
#30934=CARTESIAN_POINT('Ctrl Pts',(1.25702687965755,-1.,-1.43262645609691));
#30935=CARTESIAN_POINT('Ctrl Pts',(1.25702687965755,1.,-1.43262645609691));
#30936=CARTESIAN_POINT('Ctrl Pts',(1.25983531012005,-1.,-1.43734919180848));
#30937=CARTESIAN_POINT('Ctrl Pts',(1.25983531012005,1.,-1.43734919180848));
#30938=CARTESIAN_POINT('Ctrl Pts',(1.26273903323858,-1.,-1.44236470511303));
#30939=CARTESIAN_POINT('Ctrl Pts',(1.26273903323858,1.,-1.44236470511303));
#30940=CARTESIAN_POINT('Ctrl Pts',(1.26570925118868,-1.,-1.44761985001662));
#30941=CARTESIAN_POINT('Ctrl Pts',(1.26570925118868,1.,-1.44761985001662));
#30942=CARTESIAN_POINT('Ctrl Pts',(1.2686778680489,-1.,-1.45301422764247));
#30943=CARTESIAN_POINT('Ctrl Pts',(1.2686778680489,1.,-1.45301422764247));
#30944=CARTESIAN_POINT('Ctrl Pts',(1.27156805265289,-1.,-1.45843906294697));
#30945=CARTESIAN_POINT('Ctrl Pts',(1.27156805265289,1.,-1.45843906294697));
#30946=CARTESIAN_POINT('Ctrl Pts',(1.27433119897822,-1.,-1.46382431332476));
#30947=CARTESIAN_POINT('Ctrl Pts',(1.27433119897822,1.,-1.46382431332476));
#30948=CARTESIAN_POINT('Ctrl Pts',(1.27696414831089,-1.,-1.46916035917133));
#30949=CARTESIAN_POINT('Ctrl Pts',(1.27696414831089,1.,-1.46916035917133));
#30950=CARTESIAN_POINT('Ctrl Pts',(1.2794891824849,-1.,-1.4744717526707));
#30951=CARTESIAN_POINT('Ctrl Pts',(1.2794891824849,1.,-1.4744717526707));
#30952=CARTESIAN_POINT('Ctrl Pts',(1.28194158939517,-1.,-1.47980070347096));
#30953=CARTESIAN_POINT('Ctrl Pts',(1.28194158939517,1.,-1.47980070347096));
#30954=CARTESIAN_POINT('Ctrl Pts',(1.28435533880201,-1.,-1.4851881711891));
#30955=CARTESIAN_POINT('Ctrl Pts',(1.28435533880201,1.,-1.4851881711891));
#30956=CARTESIAN_POINT('Ctrl Pts',(1.2867467611644,-1.,-1.4906522831278));
#30957=CARTESIAN_POINT('Ctrl Pts',(1.2867467611644,1.,-1.4906522831278));
#30958=CARTESIAN_POINT('Ctrl Pts',(1.28911506584254,-1.,-1.49618896881754));
#30959=CARTESIAN_POINT('Ctrl Pts',(1.28911506584254,1.,-1.49618896881754));
#30960=CARTESIAN_POINT('Ctrl Pts',(1.29145022885181,-1.,-1.50178230149776));
#30961=CARTESIAN_POINT('Ctrl Pts',(1.29145022885181,1.,-1.50178230149776));
#30962=CARTESIAN_POINT('Ctrl Pts',(1.29373841372842,-1.,-1.50741159078365));
#30963=CARTESIAN_POINT('Ctrl Pts',(1.29373841372842,1.,-1.50741159078365));
#30964=CARTESIAN_POINT('Ctrl Pts',(1.29596850710509,-1.,-1.51305994241402));
#30965=CARTESIAN_POINT('Ctrl Pts',(1.29596850710509,1.,-1.51305994241402));
#30966=CARTESIAN_POINT('Ctrl Pts',(1.29813791800747,-1.,-1.51872184912724));
#30967=CARTESIAN_POINT('Ctrl Pts',(1.29813791800747,1.,-1.51872184912724));
#30968=CARTESIAN_POINT('Ctrl Pts',(1.30024984366328,-1.,-1.52439957861062));
#30969=CARTESIAN_POINT('Ctrl Pts',(1.30024984366328,1.,-1.52439957861062));
#30970=CARTESIAN_POINT('Ctrl Pts',(1.30231064395568,-1.,-1.53009970283891));
#30971=CARTESIAN_POINT('Ctrl Pts',(1.30231064395568,1.,-1.53009970283891));
#30972=CARTESIAN_POINT('Ctrl Pts',(1.30432735639489,-1.,-1.53582981268977));
#30973=CARTESIAN_POINT('Ctrl Pts',(1.30432735639489,1.,-1.53582981268977));
#30974=CARTESIAN_POINT('Ctrl Pts',(1.30630475189556,-1.,-1.54159462645432));
#30975=CARTESIAN_POINT('Ctrl Pts',(1.30630475189556,1.,-1.54159462645432));
#30976=CARTESIAN_POINT('Ctrl Pts',(1.30824393907473,-1.,-1.54739413957185));
#30977=CARTESIAN_POINT('Ctrl Pts',(1.30824393907473,1.,-1.54739413957185));
#30978=CARTESIAN_POINT('Ctrl Pts',(1.31014393684222,-1.,-1.55322568759481));
#30979=CARTESIAN_POINT('Ctrl Pts',(1.31014393684222,1.,-1.55322568759481));
#30980=CARTESIAN_POINT('Ctrl Pts',(1.31200264341696,-1.,-1.55908521254821));
#30981=CARTESIAN_POINT('Ctrl Pts',(1.31200264341696,1.,-1.55908521254821));
#30982=CARTESIAN_POINT('Ctrl Pts',(1.31381795281002,-1.,-1.56496872402353));
#30983=CARTESIAN_POINT('Ctrl Pts',(1.31381795281002,1.,-1.56496872402353));
#30984=CARTESIAN_POINT('Ctrl Pts',(1.31558903860016,-1.,-1.57087397835723));
#30985=CARTESIAN_POINT('Ctrl Pts',(1.31558903860016,1.,-1.57087397835723));
#30986=CARTESIAN_POINT('Ctrl Pts',(1.31731642317187,-1.,-1.5768005650559));
#30987=CARTESIAN_POINT('Ctrl Pts',(1.31731642317187,1.,-1.5768005650559));
#30988=CARTESIAN_POINT('Ctrl Pts',(1.31900135021432,-1.,-1.58274907898834));
#30989=CARTESIAN_POINT('Ctrl Pts',(1.31900135021432,1.,-1.58274907898834));
#30990=CARTESIAN_POINT('Ctrl Pts',(1.32064537110892,-1.,-1.58872057258245));
#30991=CARTESIAN_POINT('Ctrl Pts',(1.32064537110892,1.,-1.58872057258245));
#30992=CARTESIAN_POINT('Ctrl Pts',(1.32224985747682,-1.,-1.59471591079403));
#30993=CARTESIAN_POINT('Ctrl Pts',(1.32224985747682,1.,-1.59471591079403));
#30994=CARTESIAN_POINT('Ctrl Pts',(1.32381550858256,-1.,-1.60073511858687));
#30995=CARTESIAN_POINT('Ctrl Pts',(1.32381550858256,1.,-1.60073511858687));
#30996=CARTESIAN_POINT('Ctrl Pts',(1.32534250785782,-1.,-1.60677758290954));
#30997=CARTESIAN_POINT('Ctrl Pts',(1.32534250785782,1.,-1.60677758290954));
#30998=CARTESIAN_POINT('Ctrl Pts',(1.32683074483356,-1.,-1.6128423401575));
#30999=CARTESIAN_POINT('Ctrl Pts',(1.32683074483356,1.,-1.6128423401575));
#31000=CARTESIAN_POINT('Ctrl Pts',(1.32828000610449,-1.,-1.61892832270724));
#31001=CARTESIAN_POINT('Ctrl Pts',(1.32828000610449,1.,-1.61892832270724));
#31002=CARTESIAN_POINT('Ctrl Pts',(1.3296901950568,-1.,-1.62503464209797));
#31003=CARTESIAN_POINT('Ctrl Pts',(1.3296901950568,1.,-1.62503464209797));
#31004=CARTESIAN_POINT('Ctrl Pts',(1.33106149345645,-1.,-1.63116079730923));
#31005=CARTESIAN_POINT('Ctrl Pts',(1.33106149345645,1.,-1.63116079730923));
#31006=CARTESIAN_POINT('Ctrl Pts',(1.33239425103724,-1.,-1.63730653475089));
#31007=CARTESIAN_POINT('Ctrl Pts',(1.33239425103724,1.,-1.63730653475089));
#31008=CARTESIAN_POINT('Ctrl Pts',(1.33368890676572,-1.,-1.6434717485603));
#31009=CARTESIAN_POINT('Ctrl Pts',(1.33368890676572,1.,-1.6434717485603));
#31010=CARTESIAN_POINT('Ctrl Pts',(1.33494590467993,-1.,-1.6496563728683));
#31011=CARTESIAN_POINT('Ctrl Pts',(1.33494590467993,1.,-1.6496563728683));
#31012=CARTESIAN_POINT('Ctrl Pts',(1.33616559745172,-1.,-1.65586025952593));
#31013=CARTESIAN_POINT('Ctrl Pts',(1.33616559745172,1.,-1.65586025952593));
#31014=CARTESIAN_POINT('Ctrl Pts',(1.33734820885262,-1.,-1.66208312541983));
#31015=CARTESIAN_POINT('Ctrl Pts',(1.33734820885262,1.,-1.66208312541983));
#31016=CARTESIAN_POINT('Ctrl Pts',(1.33849388654388,-1.,-1.66832460783989));
#31017=CARTESIAN_POINT('Ctrl Pts',(1.33849388654388,1.,-1.66832460783989));
#31018=CARTESIAN_POINT('Ctrl Pts',(1.3396027347034,-1.,-1.67458429426086));
#31019=CARTESIAN_POINT('Ctrl Pts',(1.3396027347034,1.,-1.67458429426086));
#31020=CARTESIAN_POINT('Ctrl Pts',(1.34067485185203,-1.,-1.68086176030362));
#31021=CARTESIAN_POINT('Ctrl Pts',(1.34067485185203,1.,-1.68086176030362));
#31022=CARTESIAN_POINT('Ctrl Pts',(1.341710374848,-1.,-1.68715660868764));
#31023=CARTESIAN_POINT('Ctrl Pts',(1.341710374848,1.,-1.68715660868764));
#31024=CARTESIAN_POINT('Ctrl Pts',(1.34270948206319,-1.,-1.6934684849687));
#31025=CARTESIAN_POINT('Ctrl Pts',(1.34270948206319,1.,-1.6934684849687));
#31026=CARTESIAN_POINT('Ctrl Pts',(1.34367237124483,-1.,-1.69979707754427));
#31027=CARTESIAN_POINT('Ctrl Pts',(1.34367237124483,1.,-1.69979707754427));
#31028=CARTESIAN_POINT('Ctrl Pts',(1.34459924533831,-1.,-1.70614212266738));
#31029=CARTESIAN_POINT('Ctrl Pts',(1.34459924533831,1.,-1.70614212266738));
#31030=CARTESIAN_POINT('Ctrl Pts',(1.34549029589416,-1.,-1.71250340686822));
#31031=CARTESIAN_POINT('Ctrl Pts',(1.34549029589416,1.,-1.71250340686822));
#31032=CARTESIAN_POINT('Ctrl Pts',(1.34634568653227,-1.,-1.7188807715049));
#31033=CARTESIAN_POINT('Ctrl Pts',(1.34634568653227,1.,-1.7188807715049));
#31034=CARTESIAN_POINT('Ctrl Pts',(1.34716554819527,-1.,-1.72527410680674));
#31035=CARTESIAN_POINT('Ctrl Pts',(1.34716554819527,1.,-1.72527410680674));
#31036=CARTESIAN_POINT('Ctrl Pts',(1.34779309152035,-1.,-1.7304014965394));
#31037=CARTESIAN_POINT('Ctrl Pts',(1.34779309152035,1.,-1.7304014965394));
#31038=CARTESIAN_POINT('Ctrl Pts',(1.34824783112887,-1.,-1.73425417885907));
#31039=CARTESIAN_POINT('Ctrl Pts',(1.34824783112887,1.,-1.73425417885907));
#31040=CARTESIAN_POINT('Ctrl Pts',(1.34854391898045,-1.,-1.73682580585691));
#31041=CARTESIAN_POINT('Ctrl Pts',(1.34854391898045,1.,-1.73682580585691));
#31042=CARTESIAN_POINT('Ctrl Pts',(1.34869019493419,-1.,-1.73811241238545));
#31043=CARTESIAN_POINT('Ctrl Pts',(1.34869019493419,1.,-1.73811241238545));
#31044=CARTESIAN_POINT('',(1.15624053661742,1.,-1.31362392696032));
#31045=CARTESIAN_POINT('Ctrl Pts',(1.15624053661742,1.,-1.31362392696032));
#31046=CARTESIAN_POINT('Ctrl Pts',(1.15950888730809,1.,-1.31722977216397));
#31047=CARTESIAN_POINT('Ctrl Pts',(1.16589330093588,1.,-1.32428080721772));
#31048=CARTESIAN_POINT('Ctrl Pts',(1.17501305789857,1.,-1.33437539347008));
#31049=CARTESIAN_POINT('Ctrl Pts',(1.18625865667441,1.,-1.34687054001093));
#31050=CARTESIAN_POINT('Ctrl Pts',(1.1987959077932,1.,-1.36088705043885));
#31051=CARTESIAN_POINT('Ctrl Pts',(1.20982812925645,1.,-1.37331915607905));
#31052=CARTESIAN_POINT('Ctrl Pts',(1.21938737280852,1.,-1.38420564527715));
#31053=CARTESIAN_POINT('Ctrl Pts',(1.22752961899387,1.,-1.39361389568796));
#31054=CARTESIAN_POINT('Ctrl Pts',(1.23434087290423,1.,-1.40164708206106));
#31055=CARTESIAN_POINT('Ctrl Pts',(1.23994455029534,1.,-1.40845295531283));
#31056=CARTESIAN_POINT('Ctrl Pts',(1.24450600513056,1.,-1.41422913175179));
#31057=CARTESIAN_POINT('Ctrl Pts',(1.24824430986571,1.,-1.41923722596025));
#31058=CARTESIAN_POINT('Ctrl Pts',(1.2514145557001,1.,-1.42378102115575));
#31059=CARTESIAN_POINT('Ctrl Pts',(1.25426945222639,1.,-1.42815938799387));
#31060=CARTESIAN_POINT('Ctrl Pts',(1.25702687965755,1.,-1.43262645609691));
#31061=CARTESIAN_POINT('Ctrl Pts',(1.25983531012005,1.,-1.43734919180848));
#31062=CARTESIAN_POINT('Ctrl Pts',(1.26273903323858,1.,-1.44236470511303));
#31063=CARTESIAN_POINT('Ctrl Pts',(1.26570925118868,1.,-1.44761985001662));
#31064=CARTESIAN_POINT('Ctrl Pts',(1.2686778680489,1.,-1.45301422764247));
#31065=CARTESIAN_POINT('Ctrl Pts',(1.27156805265289,1.,-1.45843906294697));
#31066=CARTESIAN_POINT('Ctrl Pts',(1.27433119897822,1.,-1.46382431332476));
#31067=CARTESIAN_POINT('Ctrl Pts',(1.27696414831089,1.,-1.46916035917133));
#31068=CARTESIAN_POINT('Ctrl Pts',(1.2794891824849,1.,-1.4744717526707));
#31069=CARTESIAN_POINT('Ctrl Pts',(1.28194158939517,1.,-1.47980070347096));
#31070=CARTESIAN_POINT('Ctrl Pts',(1.28435533880201,1.,-1.4851881711891));
#31071=CARTESIAN_POINT('Ctrl Pts',(1.2867467611644,1.,-1.4906522831278));
#31072=CARTESIAN_POINT('Ctrl Pts',(1.28911506584254,1.,-1.49618896881754));
#31073=CARTESIAN_POINT('Ctrl Pts',(1.29145022885181,1.,-1.50178230149776));
#31074=CARTESIAN_POINT('Ctrl Pts',(1.29373841372842,1.,-1.50741159078365));
#31075=CARTESIAN_POINT('Ctrl Pts',(1.29596850710509,1.,-1.51305994241402));
#31076=CARTESIAN_POINT('Ctrl Pts',(1.29813791800747,1.,-1.51872184912724));
#31077=CARTESIAN_POINT('Ctrl Pts',(1.30024984366328,1.,-1.52439957861062));
#31078=CARTESIAN_POINT('Ctrl Pts',(1.30231064395568,1.,-1.53009970283891));
#31079=CARTESIAN_POINT('Ctrl Pts',(1.30432735639489,1.,-1.53582981268977));
#31080=CARTESIAN_POINT('Ctrl Pts',(1.30630475189556,1.,-1.54159462645432));
#31081=CARTESIAN_POINT('Ctrl Pts',(1.30824393907473,1.,-1.54739413957185));
#31082=CARTESIAN_POINT('Ctrl Pts',(1.31014393684222,1.,-1.55322568759481));
#31083=CARTESIAN_POINT('Ctrl Pts',(1.31200264341696,1.,-1.55908521254821));
#31084=CARTESIAN_POINT('Ctrl Pts',(1.31381795281002,1.,-1.56496872402353));
#31085=CARTESIAN_POINT('Ctrl Pts',(1.31558903860016,1.,-1.57087397835723));
#31086=CARTESIAN_POINT('Ctrl Pts',(1.31731642317187,1.,-1.5768005650559));
#31087=CARTESIAN_POINT('Ctrl Pts',(1.31900135021432,1.,-1.58274907898834));
#31088=CARTESIAN_POINT('Ctrl Pts',(1.32064537110892,1.,-1.58872057258245));
#31089=CARTESIAN_POINT('Ctrl Pts',(1.32224985747682,1.,-1.59471591079403));
#31090=CARTESIAN_POINT('Ctrl Pts',(1.32381550858256,1.,-1.60073511858687));
#31091=CARTESIAN_POINT('Ctrl Pts',(1.32534250785782,1.,-1.60677758290954));
#31092=CARTESIAN_POINT('Ctrl Pts',(1.32683074483356,1.,-1.6128423401575));
#31093=CARTESIAN_POINT('Ctrl Pts',(1.32828000610449,1.,-1.61892832270724));
#31094=CARTESIAN_POINT('Ctrl Pts',(1.3296901950568,1.,-1.62503464209797));
#31095=CARTESIAN_POINT('Ctrl Pts',(1.33106149345645,1.,-1.63116079730923));
#31096=CARTESIAN_POINT('Ctrl Pts',(1.33239425103724,1.,-1.63730653475089));
#31097=CARTESIAN_POINT('Ctrl Pts',(1.33368890676572,1.,-1.6434717485603));
#31098=CARTESIAN_POINT('Ctrl Pts',(1.33494590467993,1.,-1.6496563728683));
#31099=CARTESIAN_POINT('Ctrl Pts',(1.33616559745172,1.,-1.65586025952593));
#31100=CARTESIAN_POINT('Ctrl Pts',(1.33734820885262,1.,-1.66208312541983));
#31101=CARTESIAN_POINT('Ctrl Pts',(1.33849388654388,1.,-1.66832460783989));
#31102=CARTESIAN_POINT('Ctrl Pts',(1.3396027347034,1.,-1.67458429426086));
#31103=CARTESIAN_POINT('Ctrl Pts',(1.34067485185203,1.,-1.68086176030362));
#31104=CARTESIAN_POINT('Ctrl Pts',(1.341710374848,1.,-1.68715660868764));
#31105=CARTESIAN_POINT('Ctrl Pts',(1.34270948206319,1.,-1.6934684849687));
#31106=CARTESIAN_POINT('Ctrl Pts',(1.34367237124483,1.,-1.69979707754427));
#31107=CARTESIAN_POINT('Ctrl Pts',(1.34459924533831,1.,-1.70614212266738));
#31108=CARTESIAN_POINT('Ctrl Pts',(1.34549029589416,1.,-1.71250340686822));
#31109=CARTESIAN_POINT('Ctrl Pts',(1.34634568653227,1.,-1.7188807715049));
#31110=CARTESIAN_POINT('Ctrl Pts',(1.34716554819527,1.,-1.72527410680674));
#31111=CARTESIAN_POINT('Ctrl Pts',(1.34779309152035,1.,-1.7304014965394));
#31112=CARTESIAN_POINT('Ctrl Pts',(1.34824783112887,1.,-1.73425417885907));
#31113=CARTESIAN_POINT('Ctrl Pts',(1.34854391898045,1.,-1.73682580585691));
#31114=CARTESIAN_POINT('Ctrl Pts',(1.34869019493419,1.,-1.73811241238545));
#31115=CARTESIAN_POINT('',(1.15624053661742,0.,-1.31362392696032));
#31116=CARTESIAN_POINT('Origin',(0.,0.,0.));
#31117=CARTESIAN_POINT('',(1.31362392696032,1.,-1.15624053661742));
#31118=CARTESIAN_POINT('Origin',(0.,1.,0.));
#31119=CARTESIAN_POINT('',(1.31362392696032,0.,-1.15624053661742));
#31120=CARTESIAN_POINT('Ctrl Pts',(1.73811241238545,-1.,-1.34869019493419));
#31121=CARTESIAN_POINT('Ctrl Pts',(1.73811241238545,1.,-1.34869019493419));
#31122=CARTESIAN_POINT('Ctrl Pts',(1.73682580585819,-1.,-1.34854391898145));
#31123=CARTESIAN_POINT('Ctrl Pts',(1.73682580585819,1.,-1.34854391898145));
#31124=CARTESIAN_POINT('Ctrl Pts',(1.73425417886254,-1.,-1.34824783113158));
#31125=CARTESIAN_POINT('Ctrl Pts',(1.73425417886254,1.,-1.34824783113158));
#31126=CARTESIAN_POINT('Ctrl Pts',(1.73040149654497,-1.,-1.3477930915247));
#31127=CARTESIAN_POINT('Ctrl Pts',(1.73040149654497,1.,-1.3477930915247));
#31128=CARTESIAN_POINT('Ctrl Pts',(1.72527410681298,-1.,-1.34716554820013));
#31129=CARTESIAN_POINT('Ctrl Pts',(1.72527410681298,1.,-1.34716554820013));
#31130=CARTESIAN_POINT('Ctrl Pts',(1.7188807715095,-1.,-1.34634568653586));
#31131=CARTESIAN_POINT('Ctrl Pts',(1.7188807715095,1.,-1.34634568653586));
#31132=CARTESIAN_POINT('Ctrl Pts',(1.71250340687011,-1.,-1.34549029589563));
#31133=CARTESIAN_POINT('Ctrl Pts',(1.71250340687011,1.,-1.34549029589563));
#31134=CARTESIAN_POINT('Ctrl Pts',(1.70614212266676,-1.,-1.34459924533783));
#31135=CARTESIAN_POINT('Ctrl Pts',(1.70614212266676,1.,-1.34459924533783));
#31136=CARTESIAN_POINT('Ctrl Pts',(1.69979707754221,-1.,-1.34367237124322));
#31137=CARTESIAN_POINT('Ctrl Pts',(1.69979707754221,1.,-1.34367237124322));
#31138=CARTESIAN_POINT('Ctrl Pts',(1.6934684849664,-1.,-1.34270948206139));
#31139=CARTESIAN_POINT('Ctrl Pts',(1.6934684849664,1.,-1.34270948206139));
#31140=CARTESIAN_POINT('Ctrl Pts',(1.68715660868602,-1.,-1.34171037484673));
#31141=CARTESIAN_POINT('Ctrl Pts',(1.68715660868602,1.,-1.34171037484673));
#31142=CARTESIAN_POINT('Ctrl Pts',(1.68086176030308,-1.,-1.3406748518516));
#31143=CARTESIAN_POINT('Ctrl Pts',(1.68086176030308,1.,-1.3406748518516));
#31144=CARTESIAN_POINT('Ctrl Pts',(1.67458429426126,-1.,-1.33960273470372));
#31145=CARTESIAN_POINT('Ctrl Pts',(1.67458429426126,1.,-1.33960273470372));
#31146=CARTESIAN_POINT('Ctrl Pts',(1.66832460784078,-1.,-1.33849388654458));
#31147=CARTESIAN_POINT('Ctrl Pts',(1.66832460784078,1.,-1.33849388654458));
#31148=CARTESIAN_POINT('Ctrl Pts',(1.66208312542073,-1.,-1.33734820885331));
#31149=CARTESIAN_POINT('Ctrl Pts',(1.66208312542073,1.,-1.33734820885331));
#31150=CARTESIAN_POINT('Ctrl Pts',(1.65586025952651,-1.,-1.33616559745217));
#31151=CARTESIAN_POINT('Ctrl Pts',(1.65586025952651,1.,-1.33616559745217));
#31152=CARTESIAN_POINT('Ctrl Pts',(1.64965637286843,-1.,-1.33494590468003));
#31153=CARTESIAN_POINT('Ctrl Pts',(1.64965637286843,1.,-1.33494590468003));
#31154=CARTESIAN_POINT('Ctrl Pts',(1.64347174856007,-1.,-1.33368890676554));
#31155=CARTESIAN_POINT('Ctrl Pts',(1.64347174856007,1.,-1.33368890676554));
#31156=CARTESIAN_POINT('Ctrl Pts',(1.63730653475049,-1.,-1.33239425103694));
#31157=CARTESIAN_POINT('Ctrl Pts',(1.63730653475049,1.,-1.33239425103694));
#31158=CARTESIAN_POINT('Ctrl Pts',(1.63116079730887,-1.,-1.33106149345618));
#31159=CARTESIAN_POINT('Ctrl Pts',(1.63116079730887,1.,-1.33106149345618));
#31160=CARTESIAN_POINT('Ctrl Pts',(1.62503464209777,-1.,-1.32969019505665));
#31161=CARTESIAN_POINT('Ctrl Pts',(1.62503464209777,1.,-1.32969019505665));
#31162=CARTESIAN_POINT('Ctrl Pts',(1.61892832270723,-1.,-1.32828000610448));
#31163=CARTESIAN_POINT('Ctrl Pts',(1.61892832270723,1.,-1.32828000610448));
#31164=CARTESIAN_POINT('Ctrl Pts',(1.61284234015762,-1.,-1.32683074483365));
#31165=CARTESIAN_POINT('Ctrl Pts',(1.61284234015762,1.,-1.32683074483365));
#31166=CARTESIAN_POINT('Ctrl Pts',(1.6067775829097,-1.,-1.32534250785794));
#31167=CARTESIAN_POINT('Ctrl Pts',(1.6067775829097,1.,-1.32534250785794));
#31168=CARTESIAN_POINT('Ctrl Pts',(1.600735118587,-1.,-1.32381550858266));
#31169=CARTESIAN_POINT('Ctrl Pts',(1.600735118587,1.,-1.32381550858266));
#31170=CARTESIAN_POINT('Ctrl Pts',(1.59471591079408,-1.,-1.32224985747686));
#31171=CARTESIAN_POINT('Ctrl Pts',(1.59471591079408,1.,-1.32224985747686));
#31172=CARTESIAN_POINT('Ctrl Pts',(1.58872057258244,-1.,-1.32064537110891));
#31173=CARTESIAN_POINT('Ctrl Pts',(1.58872057258244,1.,-1.32064537110891));
#31174=CARTESIAN_POINT('Ctrl Pts',(1.58274907898829,-1.,-1.31900135021428));
#31175=CARTESIAN_POINT('Ctrl Pts',(1.58274907898829,1.,-1.31900135021428));
#31176=CARTESIAN_POINT('Ctrl Pts',(1.57680056505585,-1.,-1.31731642317183));
#31177=CARTESIAN_POINT('Ctrl Pts',(1.57680056505585,1.,-1.31731642317183));
#31178=CARTESIAN_POINT('Ctrl Pts',(1.57087397835721,-1.,-1.31558903860015));
#31179=CARTESIAN_POINT('Ctrl Pts',(1.57087397835721,1.,-1.31558903860015));
#31180=CARTESIAN_POINT('Ctrl Pts',(1.56496872402352,-1.,-1.31381795281002));
#31181=CARTESIAN_POINT('Ctrl Pts',(1.56496872402352,1.,-1.31381795281002));
#31182=CARTESIAN_POINT('Ctrl Pts',(1.55908521254822,-1.,-1.31200264341696));
#31183=CARTESIAN_POINT('Ctrl Pts',(1.55908521254822,1.,-1.31200264341696));
#31184=CARTESIAN_POINT('Ctrl Pts',(1.55322568759481,-1.,-1.31014393684221));
#31185=CARTESIAN_POINT('Ctrl Pts',(1.55322568759481,1.,-1.31014393684221));
#31186=CARTESIAN_POINT('Ctrl Pts',(1.54739413957183,-1.,-1.30824393907471));
#31187=CARTESIAN_POINT('Ctrl Pts',(1.54739413957183,1.,-1.30824393907471));
#31188=CARTESIAN_POINT('Ctrl Pts',(1.54159462645428,-1.,-1.30630475189553));
#31189=CARTESIAN_POINT('Ctrl Pts',(1.54159462645428,1.,-1.30630475189553));
#31190=CARTESIAN_POINT('Ctrl Pts',(1.53582981268976,-1.,-1.30432735639487));
#31191=CARTESIAN_POINT('Ctrl Pts',(1.53582981268976,1.,-1.30432735639487));
#31192=CARTESIAN_POINT('Ctrl Pts',(1.53009970283893,-1.,-1.3023106439557));
#31193=CARTESIAN_POINT('Ctrl Pts',(1.53009970283893,1.,-1.3023106439557));
#31194=CARTESIAN_POINT('Ctrl Pts',(1.5243995786107,-1.,-1.30024984366334));
#31195=CARTESIAN_POINT('Ctrl Pts',(1.5243995786107,1.,-1.30024984366334));
#31196=CARTESIAN_POINT('Ctrl Pts',(1.51872184912735,-1.,-1.29813791800757));
#31197=CARTESIAN_POINT('Ctrl Pts',(1.51872184912735,1.,-1.29813791800757));
#31198=CARTESIAN_POINT('Ctrl Pts',(1.51305994241412,-1.,-1.29596850710518));
#31199=CARTESIAN_POINT('Ctrl Pts',(1.51305994241412,1.,-1.29596850710518));
#31200=CARTESIAN_POINT('Ctrl Pts',(1.50741159078367,-1.,-1.29373841372843));
#31201=CARTESIAN_POINT('Ctrl Pts',(1.50741159078367,1.,-1.29373841372843));
#31202=CARTESIAN_POINT('Ctrl Pts',(1.50178230149764,-1.,-1.29145022885171));
#31203=CARTESIAN_POINT('Ctrl Pts',(1.50178230149764,1.,-1.29145022885171));
#31204=CARTESIAN_POINT('Ctrl Pts',(1.49618896881729,-1.,-1.28911506584232));
#31205=CARTESIAN_POINT('Ctrl Pts',(1.49618896881729,1.,-1.28911506584232));
#31206=CARTESIAN_POINT('Ctrl Pts',(1.4906522831275,-1.,-1.28674676116415));
#31207=CARTESIAN_POINT('Ctrl Pts',(1.4906522831275,1.,-1.28674676116415));
#31208=CARTESIAN_POINT('Ctrl Pts',(1.48518817118891,-1.,-1.28435533880184));
#31209=CARTESIAN_POINT('Ctrl Pts',(1.48518817118891,1.,-1.28435533880184));
#31210=CARTESIAN_POINT('Ctrl Pts',(1.47980070347102,-1.,-1.28194158939522));
#31211=CARTESIAN_POINT('Ctrl Pts',(1.47980070347102,1.,-1.28194158939522));
#31212=CARTESIAN_POINT('Ctrl Pts',(1.4744717526711,-1.,-1.27948918248524));
#31213=CARTESIAN_POINT('Ctrl Pts',(1.4744717526711,1.,-1.27948918248524));
#31214=CARTESIAN_POINT('Ctrl Pts',(1.46916035917197,-1.,-1.27696414831144));
#31215=CARTESIAN_POINT('Ctrl Pts',(1.46916035917197,1.,-1.27696414831144));
#31216=CARTESIAN_POINT('Ctrl Pts',(1.4638243133254,-1.,-1.27433119897877));
#31217=CARTESIAN_POINT('Ctrl Pts',(1.4638243133254,1.,-1.27433119897877));
#31218=CARTESIAN_POINT('Ctrl Pts',(1.45843906294725,-1.,-1.27156805265312));
#31219=CARTESIAN_POINT('Ctrl Pts',(1.45843906294725,1.,-1.27156805265312));
#31220=CARTESIAN_POINT('Ctrl Pts',(1.45301422764205,-1.,-1.26867786804854));
#31221=CARTESIAN_POINT('Ctrl Pts',(1.45301422764205,1.,-1.26867786804854));
#31222=CARTESIAN_POINT('Ctrl Pts',(1.44761985001544,-1.,-1.26570925118767));
#31223=CARTESIAN_POINT('Ctrl Pts',(1.44761985001544,1.,-1.26570925118767));
#31224=CARTESIAN_POINT('Ctrl Pts',(1.44236470511145,-1.,-1.26273903323723));
#31225=CARTESIAN_POINT('Ctrl Pts',(1.44236470511145,1.,-1.26273903323723));
#31226=CARTESIAN_POINT('Ctrl Pts',(1.43734919180719,-1.,-1.25983531011894));
#31227=CARTESIAN_POINT('Ctrl Pts',(1.43734919180719,1.,-1.25983531011894));
#31228=CARTESIAN_POINT('Ctrl Pts',(1.43262645609679,-1.,-1.25702687965744));
#31229=CARTESIAN_POINT('Ctrl Pts',(1.43262645609679,1.,-1.25702687965744));
#31230=CARTESIAN_POINT('Ctrl Pts',(1.42815938799555,-1.,-1.25426945222783));
#31231=CARTESIAN_POINT('Ctrl Pts',(1.42815938799555,1.,-1.25426945222783));
#31232=CARTESIAN_POINT('Ctrl Pts',(1.42378102115911,-1.,-1.25141455570299));
#31233=CARTESIAN_POINT('Ctrl Pts',(1.42378102115911,1.,-1.25141455570299));
#31234=CARTESIAN_POINT('Ctrl Pts',(1.41923722596421,-1.,-1.24824430986911));
#31235=CARTESIAN_POINT('Ctrl Pts',(1.41923722596421,1.,-1.24824430986911));
#31236=CARTESIAN_POINT('Ctrl Pts',(1.41422913175437,-1.,-1.24450600513278));
#31237=CARTESIAN_POINT('Ctrl Pts',(1.41422913175437,1.,-1.24450600513278));
#31238=CARTESIAN_POINT('Ctrl Pts',(1.40845295531151,-1.,-1.23994455029421));
#31239=CARTESIAN_POINT('Ctrl Pts',(1.40845295531151,1.,-1.23994455029421));
#31240=CARTESIAN_POINT('Ctrl Pts',(1.40164708205345,-1.,-1.23434087289768));
#31241=CARTESIAN_POINT('Ctrl Pts',(1.40164708205345,1.,-1.23434087289768));
#31242=CARTESIAN_POINT('Ctrl Pts',(1.39361389567257,-1.,-1.22752961898063));
#31243=CARTESIAN_POINT('Ctrl Pts',(1.39361389567257,1.,-1.22752961898063));
#31244=CARTESIAN_POINT('Ctrl Pts',(1.38420564525391,-1.,-1.21938737278853));
#31245=CARTESIAN_POINT('Ctrl Pts',(1.38420564525391,1.,-1.21938737278853));
#31246=CARTESIAN_POINT('Ctrl Pts',(1.37331915604962,-1.,-1.20982812923113));
#31247=CARTESIAN_POINT('Ctrl Pts',(1.37331915604962,1.,-1.20982812923113));
#31248=CARTESIAN_POINT('Ctrl Pts',(1.36088705040677,-1.,-1.1987959077656));
#31249=CARTESIAN_POINT('Ctrl Pts',(1.36088705040677,1.,-1.1987959077656));
#31250=CARTESIAN_POINT('Ctrl Pts',(1.34687053998157,-1.,-1.18625865664915));
#31251=CARTESIAN_POINT('Ctrl Pts',(1.34687053998157,1.,-1.18625865664915));
#31252=CARTESIAN_POINT('Ctrl Pts',(1.33437539344842,-1.,-1.17501305787994));
#31253=CARTESIAN_POINT('Ctrl Pts',(1.33437539344842,1.,-1.17501305787994));
#31254=CARTESIAN_POINT('Ctrl Pts',(1.32428080720544,-1.,-1.16589330092532));
#31255=CARTESIAN_POINT('Ctrl Pts',(1.32428080720544,1.,-1.16589330092532));
#31256=CARTESIAN_POINT('Ctrl Pts',(1.3172297721596,-1.,-1.15950888730433));
#31257=CARTESIAN_POINT('Ctrl Pts',(1.3172297721596,1.,-1.15950888730433));
#31258=CARTESIAN_POINT('Ctrl Pts',(1.31362392696032,-1.,-1.15624053661742));
#31259=CARTESIAN_POINT('Ctrl Pts',(1.31362392696032,1.,-1.15624053661742));
#31260=CARTESIAN_POINT('',(1.73811241238545,1.,-1.34869019493419));
#31261=CARTESIAN_POINT('Ctrl Pts',(1.73811241238545,1.,-1.34869019493419));
#31262=CARTESIAN_POINT('Ctrl Pts',(1.73682580585819,1.,-1.34854391898145));
#31263=CARTESIAN_POINT('Ctrl Pts',(1.73425417886254,1.,-1.34824783113158));
#31264=CARTESIAN_POINT('Ctrl Pts',(1.73040149654497,1.,-1.3477930915247));
#31265=CARTESIAN_POINT('Ctrl Pts',(1.72527410681298,1.,-1.34716554820013));
#31266=CARTESIAN_POINT('Ctrl Pts',(1.7188807715095,1.,-1.34634568653586));
#31267=CARTESIAN_POINT('Ctrl Pts',(1.71250340687011,1.,-1.34549029589563));
#31268=CARTESIAN_POINT('Ctrl Pts',(1.70614212266676,1.,-1.34459924533783));
#31269=CARTESIAN_POINT('Ctrl Pts',(1.69979707754221,1.,-1.34367237124322));
#31270=CARTESIAN_POINT('Ctrl Pts',(1.6934684849664,1.,-1.34270948206139));
#31271=CARTESIAN_POINT('Ctrl Pts',(1.68715660868602,1.,-1.34171037484673));
#31272=CARTESIAN_POINT('Ctrl Pts',(1.68086176030308,1.,-1.3406748518516));
#31273=CARTESIAN_POINT('Ctrl Pts',(1.67458429426126,1.,-1.33960273470372));
#31274=CARTESIAN_POINT('Ctrl Pts',(1.66832460784078,1.,-1.33849388654458));
#31275=CARTESIAN_POINT('Ctrl Pts',(1.66208312542073,1.,-1.33734820885331));
#31276=CARTESIAN_POINT('Ctrl Pts',(1.65586025952651,1.,-1.33616559745217));
#31277=CARTESIAN_POINT('Ctrl Pts',(1.64965637286843,1.,-1.33494590468003));
#31278=CARTESIAN_POINT('Ctrl Pts',(1.64347174856007,1.,-1.33368890676554));
#31279=CARTESIAN_POINT('Ctrl Pts',(1.63730653475049,1.,-1.33239425103694));
#31280=CARTESIAN_POINT('Ctrl Pts',(1.63116079730887,1.,-1.33106149345618));
#31281=CARTESIAN_POINT('Ctrl Pts',(1.62503464209777,1.,-1.32969019505665));
#31282=CARTESIAN_POINT('Ctrl Pts',(1.61892832270723,1.,-1.32828000610448));
#31283=CARTESIAN_POINT('Ctrl Pts',(1.61284234015762,1.,-1.32683074483365));
#31284=CARTESIAN_POINT('Ctrl Pts',(1.6067775829097,1.,-1.32534250785794));
#31285=CARTESIAN_POINT('Ctrl Pts',(1.600735118587,1.,-1.32381550858266));
#31286=CARTESIAN_POINT('Ctrl Pts',(1.59471591079408,1.,-1.32224985747686));
#31287=CARTESIAN_POINT('Ctrl Pts',(1.58872057258244,1.,-1.32064537110891));
#31288=CARTESIAN_POINT('Ctrl Pts',(1.58274907898829,1.,-1.31900135021428));
#31289=CARTESIAN_POINT('Ctrl Pts',(1.57680056505585,1.,-1.31731642317183));
#31290=CARTESIAN_POINT('Ctrl Pts',(1.57087397835721,1.,-1.31558903860015));
#31291=CARTESIAN_POINT('Ctrl Pts',(1.56496872402352,1.,-1.31381795281002));
#31292=CARTESIAN_POINT('Ctrl Pts',(1.55908521254822,1.,-1.31200264341696));
#31293=CARTESIAN_POINT('Ctrl Pts',(1.55322568759481,1.,-1.31014393684221));
#31294=CARTESIAN_POINT('Ctrl Pts',(1.54739413957183,1.,-1.30824393907471));
#31295=CARTESIAN_POINT('Ctrl Pts',(1.54159462645428,1.,-1.30630475189553));
#31296=CARTESIAN_POINT('Ctrl Pts',(1.53582981268976,1.,-1.30432735639487));
#31297=CARTESIAN_POINT('Ctrl Pts',(1.53009970283893,1.,-1.3023106439557));
#31298=CARTESIAN_POINT('Ctrl Pts',(1.5243995786107,1.,-1.30024984366334));
#31299=CARTESIAN_POINT('Ctrl Pts',(1.51872184912735,1.,-1.29813791800757));
#31300=CARTESIAN_POINT('Ctrl Pts',(1.51305994241412,1.,-1.29596850710518));
#31301=CARTESIAN_POINT('Ctrl Pts',(1.50741159078367,1.,-1.29373841372843));
#31302=CARTESIAN_POINT('Ctrl Pts',(1.50178230149764,1.,-1.29145022885171));
#31303=CARTESIAN_POINT('Ctrl Pts',(1.49618896881729,1.,-1.28911506584232));
#31304=CARTESIAN_POINT('Ctrl Pts',(1.4906522831275,1.,-1.28674676116415));
#31305=CARTESIAN_POINT('Ctrl Pts',(1.48518817118891,1.,-1.28435533880184));
#31306=CARTESIAN_POINT('Ctrl Pts',(1.47980070347102,1.,-1.28194158939522));
#31307=CARTESIAN_POINT('Ctrl Pts',(1.4744717526711,1.,-1.27948918248524));
#31308=CARTESIAN_POINT('Ctrl Pts',(1.46916035917197,1.,-1.27696414831144));
#31309=CARTESIAN_POINT('Ctrl Pts',(1.4638243133254,1.,-1.27433119897877));
#31310=CARTESIAN_POINT('Ctrl Pts',(1.45843906294725,1.,-1.27156805265312));
#31311=CARTESIAN_POINT('Ctrl Pts',(1.45301422764205,1.,-1.26867786804854));
#31312=CARTESIAN_POINT('Ctrl Pts',(1.44761985001544,1.,-1.26570925118767));
#31313=CARTESIAN_POINT('Ctrl Pts',(1.44236470511145,1.,-1.26273903323723));
#31314=CARTESIAN_POINT('Ctrl Pts',(1.43734919180719,1.,-1.25983531011894));
#31315=CARTESIAN_POINT('Ctrl Pts',(1.43262645609679,1.,-1.25702687965744));
#31316=CARTESIAN_POINT('Ctrl Pts',(1.42815938799555,1.,-1.25426945222783));
#31317=CARTESIAN_POINT('Ctrl Pts',(1.42378102115911,1.,-1.25141455570299));
#31318=CARTESIAN_POINT('Ctrl Pts',(1.41923722596421,1.,-1.24824430986911));
#31319=CARTESIAN_POINT('Ctrl Pts',(1.41422913175437,1.,-1.24450600513278));
#31320=CARTESIAN_POINT('Ctrl Pts',(1.40845295531151,1.,-1.23994455029421));
#31321=CARTESIAN_POINT('Ctrl Pts',(1.40164708205345,1.,-1.23434087289768));
#31322=CARTESIAN_POINT('Ctrl Pts',(1.39361389567257,1.,-1.22752961898063));
#31323=CARTESIAN_POINT('Ctrl Pts',(1.38420564525391,1.,-1.21938737278853));
#31324=CARTESIAN_POINT('Ctrl Pts',(1.37331915604962,1.,-1.20982812923113));
#31325=CARTESIAN_POINT('Ctrl Pts',(1.36088705040677,1.,-1.1987959077656));
#31326=CARTESIAN_POINT('Ctrl Pts',(1.34687053998157,1.,-1.18625865664915));
#31327=CARTESIAN_POINT('Ctrl Pts',(1.33437539344842,1.,-1.17501305787994));
#31328=CARTESIAN_POINT('Ctrl Pts',(1.32428080720544,1.,-1.16589330092532));
#31329=CARTESIAN_POINT('Ctrl Pts',(1.3172297721596,1.,-1.15950888730433));
#31330=CARTESIAN_POINT('Ctrl Pts',(1.31362392696032,1.,-1.15624053661742));
#31331=CARTESIAN_POINT('',(1.73811241238545,0.,-1.34869019493419));
#31332=CARTESIAN_POINT('Origin',(1.81978687191668,0.,-1.23627494547115));
#31333=CARTESIAN_POINT('',(1.81978687191668,1.,-1.23627494547115));
#31334=CARTESIAN_POINT('',(1.73811241238545,1.,-1.34869019493419));
#31335=CARTESIAN_POINT('',(1.81978687191668,0.,-1.23627494547115));
#31336=CARTESIAN_POINT('Ctrl Pts',(1.5055822144029,-1.,-0.892032620296855));
#31337=CARTESIAN_POINT('Ctrl Pts',(1.5055822144029,1.,-0.892032620296855));
#31338=CARTESIAN_POINT('Ctrl Pts',(1.50980486807181,-1.,-0.894452006967538));
#31339=CARTESIAN_POINT('Ctrl Pts',(1.50980486807181,1.,-0.894452006967538));
#31340=CARTESIAN_POINT('Ctrl Pts',(1.51805569591479,-1.,-0.89918504749193));
#31341=CARTESIAN_POINT('Ctrl Pts',(1.51805569591479,1.,-0.89918504749193));
#31342=CARTESIAN_POINT('Ctrl Pts',(1.52984849890434,-1.,-0.905967409640499));
#31343=CARTESIAN_POINT('Ctrl Pts',(1.52984849890434,1.,-0.905967409640499));
#31344=CARTESIAN_POINT('Ctrl Pts',(1.54440491152807,-1.,-0.91437591904658));
#31345=CARTESIAN_POINT('Ctrl Pts',(1.54440491152807,1.,-0.91437591904658));
#31346=CARTESIAN_POINT('Ctrl Pts',(1.56065988582509,-1.,-0.923832188966322));
#31347=CARTESIAN_POINT('Ctrl Pts',(1.56065988582509,1.,-0.923832188966322));
#31348=CARTESIAN_POINT('Ctrl Pts',(1.57499388385561,-1.,-0.932246680128849));
#31349=CARTESIAN_POINT('Ctrl Pts',(1.57499388385561,1.,-0.932246680128849));
#31350=CARTESIAN_POINT('Ctrl Pts',(1.58744937489796,-1.,-0.939646377909319));
#31351=CARTESIAN_POINT('Ctrl Pts',(1.58744937489796,1.,-0.939646377909319));
#31352=CARTESIAN_POINT('Ctrl Pts',(1.59810042045408,-1.,-0.946078063325796));
#31353=CARTESIAN_POINT('Ctrl Pts',(1.59810042045408,1.,-0.946078063325796));
#31354=CARTESIAN_POINT('Ctrl Pts',(1.60706069897794,-1.,-0.951613284361248));
#31355=CARTESIAN_POINT('Ctrl Pts',(1.60706069897794,1.,-0.951613284361248));
#31356=CARTESIAN_POINT('Ctrl Pts',(1.61449324337233,-1.,-0.956354422921573));
#31357=CARTESIAN_POINT('Ctrl Pts',(1.61449324337233,1.,-0.956354422921573));
#31358=CARTESIAN_POINT('Ctrl Pts',(1.62061638139929,-1.,-0.960438326099958));
#31359=CARTESIAN_POINT('Ctrl Pts',(1.62061638139929,1.,-0.960438326099958));
#31360=CARTESIAN_POINT('Ctrl Pts',(1.6257193066974,-1.,-0.964046107037821));
#31361=CARTESIAN_POINT('Ctrl Pts',(1.6257193066974,1.,-0.964046107037821));
#31362=CARTESIAN_POINT('Ctrl Pts',(1.63013849959083,-1.,-0.967387853228041));
#31363=CARTESIAN_POINT('Ctrl Pts',(1.63013849959083,1.,-0.967387853228041));
#31364=CARTESIAN_POINT('Ctrl Pts',(1.63420665729609,-1.,-0.970669715996356));
#31365=CARTESIAN_POINT('Ctrl Pts',(1.63420665729609,1.,-0.970669715996356));
#31366=CARTESIAN_POINT('Ctrl Pts',(1.63820952658157,-1.,-0.974066058287501));
#31367=CARTESIAN_POINT('Ctrl Pts',(1.63820952658157,1.,-0.974066058287501));
#31368=CARTESIAN_POINT('Ctrl Pts',(1.64233990826831,-1.,-0.977689794120297));
#31369=CARTESIAN_POINT('Ctrl Pts',(1.64233990826831,1.,-0.977689794120297));
#31370=CARTESIAN_POINT('Ctrl Pts',(1.64665139190834,-1.,-0.981562530940574));
#31371=CARTESIAN_POINT('Ctrl Pts',(1.64665139190834,1.,-0.981562530940574));
#31372=CARTESIAN_POINT('Ctrl Pts',(1.6511001661277,-1.,-0.985642622921626));
#31373=CARTESIAN_POINT('Ctrl Pts',(1.6511001661277,1.,-0.985642622921626));
#31374=CARTESIAN_POINT('Ctrl Pts',(1.65559044289746,-1.,-0.98985562785445));
#31375=CARTESIAN_POINT('Ctrl Pts',(1.65559044289746,1.,-0.98985562785445));
#31376=CARTESIAN_POINT('Ctrl Pts',(1.66001553809916,-1.,-0.994121836661116));
#31377=CARTESIAN_POINT('Ctrl Pts',(1.66001553809916,1.,-0.994121836661116));
#31378=CARTESIAN_POINT('Ctrl Pts',(1.66430758030304,-1.,-0.998389654952317));
#31379=CARTESIAN_POINT('Ctrl Pts',(1.66430758030304,1.,-0.998389654952317));
#31380=CARTESIAN_POINT('Ctrl Pts',(1.66846059277231,-1.,-1.00265091003682));
#31381=CARTESIAN_POINT('Ctrl Pts',(1.66846059277231,1.,-1.00265091003682));
#31382=CARTESIAN_POINT('Ctrl Pts',(1.67250335383248,-1.,-1.00692206696387));
#31383=CARTESIAN_POINT('Ctrl Pts',(1.67250335383248,1.,-1.00692206696387));
#31384=CARTESIAN_POINT('Ctrl Pts',(1.67648246776457,-1.,-1.01123236493507));
#31385=CARTESIAN_POINT('Ctrl Pts',(1.67648246776457,1.,-1.01123236493507));
#31386=CARTESIAN_POINT('Ctrl Pts',(1.6804428989482,-1.,-1.01561026162787));
#31387=CARTESIAN_POINT('Ctrl Pts',(1.6804428989482,1.,-1.01561026162787));
#31388=CARTESIAN_POINT('Ctrl Pts',(1.68440578021739,-1.,-1.02006795074222));
#31389=CARTESIAN_POINT('Ctrl Pts',(1.68440578021739,1.,-1.02006795074222));
#31390=CARTESIAN_POINT('Ctrl Pts',(1.68836910178475,-1.,-1.02460180535272));
#31391=CARTESIAN_POINT('Ctrl Pts',(1.68836910178475,1.,-1.02460180535272));
#31392=CARTESIAN_POINT('Ctrl Pts',(1.69231840863471,-1.,-1.02919977579155));
#31393=CARTESIAN_POINT('Ctrl Pts',(1.69231840863471,1.,-1.02919977579155));
#31394=CARTESIAN_POINT('Ctrl Pts',(1.69623414782769,-1.,-1.03384646003587));
#31395=CARTESIAN_POINT('Ctrl Pts',(1.69623414782769,1.,-1.03384646003587));
#31396=CARTESIAN_POINT('Ctrl Pts',(1.70010052930951,-1.,-1.03852922490782));
#31397=CARTESIAN_POINT('Ctrl Pts',(1.70010052930951,1.,-1.03852922490782));
#31398=CARTESIAN_POINT('Ctrl Pts',(1.70391338707969,-1.,-1.04324363334546));
#31399=CARTESIAN_POINT('Ctrl Pts',(1.70391338707969,1.,-1.04324363334546));
#31400=CARTESIAN_POINT('Ctrl Pts',(1.70767646263641,-1.,-1.0479908540499));
#31401=CARTESIAN_POINT('Ctrl Pts',(1.70767646263641,1.,-1.0479908540499));
#31402=CARTESIAN_POINT('Ctrl Pts',(1.71139783543986,-1.,-1.05277517202854));
#31403=CARTESIAN_POINT('Ctrl Pts',(1.71139783543986,1.,-1.05277517202854));
#31404=CARTESIAN_POINT('Ctrl Pts',(1.71508654427022,-1.,-1.05760163192481));
#31405=CARTESIAN_POINT('Ctrl Pts',(1.71508654427022,1.,-1.05760163192481));
#31406=CARTESIAN_POINT('Ctrl Pts',(1.71874858456908,-1.,-1.0624732468065));
#31407=CARTESIAN_POINT('Ctrl Pts',(1.71874858456908,1.,-1.0624732468065));
#31408=CARTESIAN_POINT('Ctrl Pts',(1.72238500928456,-1.,-1.06738966975463));
#31409=CARTESIAN_POINT('Ctrl Pts',(1.72238500928456,1.,-1.06738966975463));
#31410=CARTESIAN_POINT('Ctrl Pts',(1.72599406198489,-1.,-1.07234866990252));
#31411=CARTESIAN_POINT('Ctrl Pts',(1.72599406198489,1.,-1.07234866990252));
#31412=CARTESIAN_POINT('Ctrl Pts',(1.72957248977424,-1.,-1.0773470373727));
#31413=CARTESIAN_POINT('Ctrl Pts',(1.72957248977424,1.,-1.0773470373727));
#31414=CARTESIAN_POINT('Ctrl Pts',(1.73311705663407,-1.,-1.08238162784749));
#31415=CARTESIAN_POINT('Ctrl Pts',(1.73311705663407,1.,-1.08238162784749));
#31416=CARTESIAN_POINT('Ctrl Pts',(1.73662628326093,-1.,-1.08745056285429));
#31417=CARTESIAN_POINT('Ctrl Pts',(1.73662628326093,1.,-1.08745056285429));
#31418=CARTESIAN_POINT('Ctrl Pts',(1.74010053962252,-1.,-1.09255329056496));
#31419=CARTESIAN_POINT('Ctrl Pts',(1.74010053962252,1.,-1.09255329056496));
#31420=CARTESIAN_POINT('Ctrl Pts',(1.74354119236212,-1.,-1.09768999241229));
#31421=CARTESIAN_POINT('Ctrl Pts',(1.74354119236212,1.,-1.09768999241229));
#31422=CARTESIAN_POINT('Ctrl Pts',(1.74695004214924,-1.,-1.10286118991144));
#31423=CARTESIAN_POINT('Ctrl Pts',(1.74695004214924,1.,-1.10286118991144));
#31424=CARTESIAN_POINT('Ctrl Pts',(1.75032866075914,-1.,-1.10806728183003));
#31425=CARTESIAN_POINT('Ctrl Pts',(1.75032866075914,1.,-1.10806728183003));
#31426=CARTESIAN_POINT('Ctrl Pts',(1.75367772094617,-1.,-1.11330807582542));
#31427=CARTESIAN_POINT('Ctrl Pts',(1.75367772094617,1.,-1.11330807582542));
#31428=CARTESIAN_POINT('Ctrl Pts',(1.75699720772089,-1.,-1.11858293216752));
#31429=CARTESIAN_POINT('Ctrl Pts',(1.75699720772089,1.,-1.11858293216752));
#31430=CARTESIAN_POINT('Ctrl Pts',(1.76028671825084,-1.,-1.12389096855078));
#31431=CARTESIAN_POINT('Ctrl Pts',(1.76028671825084,1.,-1.12389096855078));
#31432=CARTESIAN_POINT('Ctrl Pts',(1.76354571966171,-1.,-1.12923123555076));
#31433=CARTESIAN_POINT('Ctrl Pts',(1.76354571966171,1.,-1.12923123555076));
#31434=CARTESIAN_POINT('Ctrl Pts',(1.76677384551883,-1.,-1.13460291804635));
#31435=CARTESIAN_POINT('Ctrl Pts',(1.76677384551883,1.,-1.13460291804635));
#31436=CARTESIAN_POINT('Ctrl Pts',(1.76997111386806,-1.,-1.14000548337));
#31437=CARTESIAN_POINT('Ctrl Pts',(1.76997111386806,1.,-1.14000548337));
#31438=CARTESIAN_POINT('Ctrl Pts',(1.77313777896234,-1.,-1.14543858226948));
#31439=CARTESIAN_POINT('Ctrl Pts',(1.77313777896234,1.,-1.14543858226948));
#31440=CARTESIAN_POINT('Ctrl Pts',(1.77627422557034,-1.,-1.15090197841531));
#31441=CARTESIAN_POINT('Ctrl Pts',(1.77627422557034,1.,-1.15090197841531));
#31442=CARTESIAN_POINT('Ctrl Pts',(1.77938085564261,-1.,-1.15639547194689));
#31443=CARTESIAN_POINT('Ctrl Pts',(1.77938085564261,1.,-1.15639547194689));
#31444=CARTESIAN_POINT('Ctrl Pts',(1.78245795880949,-1.,-1.16191881298458));
#31445=CARTESIAN_POINT('Ctrl Pts',(1.78245795880949,1.,-1.16191881298458));
#31446=CARTESIAN_POINT('Ctrl Pts',(1.78550566040349,-1.,-1.16747166312239));
#31447=CARTESIAN_POINT('Ctrl Pts',(1.78550566040349,1.,-1.16747166312239));
#31448=CARTESIAN_POINT('Ctrl Pts',(1.78852398877523,-1.,-1.17305363177265));
#31449=CARTESIAN_POINT('Ctrl Pts',(1.78852398877523,1.,-1.17305363177265));
#31450=CARTESIAN_POINT('Ctrl Pts',(1.79151291552646,-1.,-1.17866429440781));
#31451=CARTESIAN_POINT('Ctrl Pts',(1.79151291552646,1.,-1.17866429440781));
#31452=CARTESIAN_POINT('Ctrl Pts',(1.79447240321572,-1.,-1.18430321697471));
#31453=CARTESIAN_POINT('Ctrl Pts',(1.79447240321572,1.,-1.18430321697471));
#31454=CARTESIAN_POINT('Ctrl Pts',(1.79740245923649,-1.,-1.1899699793456));
#31455=CARTESIAN_POINT('Ctrl Pts',(1.79740245923649,1.,-1.1899699793456));
#31456=CARTESIAN_POINT('Ctrl Pts',(1.80030314370121,-1.,-1.19566418930405));
#31457=CARTESIAN_POINT('Ctrl Pts',(1.80030314370121,1.,-1.19566418930405));
#31458=CARTESIAN_POINT('Ctrl Pts',(1.8031745483882,-1.,-1.2013854893912));
#31459=CARTESIAN_POINT('Ctrl Pts',(1.8031745483882,1.,-1.2013854893912));
#31460=CARTESIAN_POINT('Ctrl Pts',(1.80601678480772,-1.,-1.20713356605519));
#31461=CARTESIAN_POINT('Ctrl Pts',(1.80601678480772,1.,-1.20713356605519));
#31462=CARTESIAN_POINT('Ctrl Pts',(1.80882996916931,-1.,-1.2129081570818));
#31463=CARTESIAN_POINT('Ctrl Pts',(1.80882996916931,1.,-1.2129081570818));
#31464=CARTESIAN_POINT('Ctrl Pts',(1.81161420806172,-1.,-1.2187090610323));
#31465=CARTESIAN_POINT('Ctrl Pts',(1.81161420806172,1.,-1.2187090610323));
#31466=CARTESIAN_POINT('Ctrl Pts',(1.81436959209778,-1.,-1.22453613304507));
#31467=CARTESIAN_POINT('Ctrl Pts',(1.81436959209778,1.,-1.22453613304507));
#31468=CARTESIAN_POINT('Ctrl Pts',(1.81655087183054,-1.,-1.22921864890975));
#31469=CARTESIAN_POINT('Ctrl Pts',(1.81655087183054,1.,-1.22921864890975));
#31470=CARTESIAN_POINT('Ctrl Pts',(1.81817389920914,-1.,-1.23274224526804));
#31471=CARTESIAN_POINT('Ctrl Pts',(1.81817389920914,1.,-1.23274224526804));
#31472=CARTESIAN_POINT('Ctrl Pts',(1.81925017193531,-1.,-1.23509651170384));
#31473=CARTESIAN_POINT('Ctrl Pts',(1.81925017193531,1.,-1.23509651170384));
#31474=CARTESIAN_POINT('Ctrl Pts',(1.81978687191668,-1.,-1.23627494547115));
#31475=CARTESIAN_POINT('Ctrl Pts',(1.81978687191668,1.,-1.23627494547115));
#31476=CARTESIAN_POINT('',(1.5055822144029,1.,-0.892032620296855));
#31477=CARTESIAN_POINT('Ctrl Pts',(1.5055822144029,1.,-0.892032620296855));
#31478=CARTESIAN_POINT('Ctrl Pts',(1.50980486807181,1.,-0.894452006967538));
#31479=CARTESIAN_POINT('Ctrl Pts',(1.51805569591479,1.,-0.89918504749193));
#31480=CARTESIAN_POINT('Ctrl Pts',(1.52984849890434,1.,-0.905967409640499));
#31481=CARTESIAN_POINT('Ctrl Pts',(1.54440491152807,1.,-0.91437591904658));
#31482=CARTESIAN_POINT('Ctrl Pts',(1.56065988582509,1.,-0.923832188966322));
#31483=CARTESIAN_POINT('Ctrl Pts',(1.57499388385561,1.,-0.932246680128849));
#31484=CARTESIAN_POINT('Ctrl Pts',(1.58744937489796,1.,-0.939646377909319));
#31485=CARTESIAN_POINT('Ctrl Pts',(1.59810042045408,1.,-0.946078063325796));
#31486=CARTESIAN_POINT('Ctrl Pts',(1.60706069897794,1.,-0.951613284361248));
#31487=CARTESIAN_POINT('Ctrl Pts',(1.61449324337233,1.,-0.956354422921573));
#31488=CARTESIAN_POINT('Ctrl Pts',(1.62061638139929,1.,-0.960438326099958));
#31489=CARTESIAN_POINT('Ctrl Pts',(1.6257193066974,1.,-0.964046107037821));
#31490=CARTESIAN_POINT('Ctrl Pts',(1.63013849959083,1.,-0.967387853228041));
#31491=CARTESIAN_POINT('Ctrl Pts',(1.63420665729609,1.,-0.970669715996356));
#31492=CARTESIAN_POINT('Ctrl Pts',(1.63820952658157,1.,-0.974066058287501));
#31493=CARTESIAN_POINT('Ctrl Pts',(1.64233990826831,1.,-0.977689794120297));
#31494=CARTESIAN_POINT('Ctrl Pts',(1.64665139190834,1.,-0.981562530940574));
#31495=CARTESIAN_POINT('Ctrl Pts',(1.6511001661277,1.,-0.985642622921626));
#31496=CARTESIAN_POINT('Ctrl Pts',(1.65559044289746,1.,-0.98985562785445));
#31497=CARTESIAN_POINT('Ctrl Pts',(1.66001553809916,1.,-0.994121836661116));
#31498=CARTESIAN_POINT('Ctrl Pts',(1.66430758030304,1.,-0.998389654952317));
#31499=CARTESIAN_POINT('Ctrl Pts',(1.66846059277231,1.,-1.00265091003682));
#31500=CARTESIAN_POINT('Ctrl Pts',(1.67250335383248,1.,-1.00692206696387));
#31501=CARTESIAN_POINT('Ctrl Pts',(1.67648246776457,1.,-1.01123236493507));
#31502=CARTESIAN_POINT('Ctrl Pts',(1.6804428989482,1.,-1.01561026162787));
#31503=CARTESIAN_POINT('Ctrl Pts',(1.68440578021739,1.,-1.02006795074222));
#31504=CARTESIAN_POINT('Ctrl Pts',(1.68836910178475,1.,-1.02460180535272));
#31505=CARTESIAN_POINT('Ctrl Pts',(1.69231840863471,1.,-1.02919977579155));
#31506=CARTESIAN_POINT('Ctrl Pts',(1.69623414782769,1.,-1.03384646003587));
#31507=CARTESIAN_POINT('Ctrl Pts',(1.70010052930951,1.,-1.03852922490782));
#31508=CARTESIAN_POINT('Ctrl Pts',(1.70391338707969,1.,-1.04324363334546));
#31509=CARTESIAN_POINT('Ctrl Pts',(1.70767646263641,1.,-1.0479908540499));
#31510=CARTESIAN_POINT('Ctrl Pts',(1.71139783543986,1.,-1.05277517202854));
#31511=CARTESIAN_POINT('Ctrl Pts',(1.71508654427022,1.,-1.05760163192481));
#31512=CARTESIAN_POINT('Ctrl Pts',(1.71874858456908,1.,-1.0624732468065));
#31513=CARTESIAN_POINT('Ctrl Pts',(1.72238500928456,1.,-1.06738966975463));
#31514=CARTESIAN_POINT('Ctrl Pts',(1.72599406198489,1.,-1.07234866990252));
#31515=CARTESIAN_POINT('Ctrl Pts',(1.72957248977424,1.,-1.0773470373727));
#31516=CARTESIAN_POINT('Ctrl Pts',(1.73311705663407,1.,-1.08238162784749));
#31517=CARTESIAN_POINT('Ctrl Pts',(1.73662628326093,1.,-1.08745056285429));
#31518=CARTESIAN_POINT('Ctrl Pts',(1.74010053962252,1.,-1.09255329056496));
#31519=CARTESIAN_POINT('Ctrl Pts',(1.74354119236212,1.,-1.09768999241229));
#31520=CARTESIAN_POINT('Ctrl Pts',(1.74695004214924,1.,-1.10286118991144));
#31521=CARTESIAN_POINT('Ctrl Pts',(1.75032866075914,1.,-1.10806728183003));
#31522=CARTESIAN_POINT('Ctrl Pts',(1.75367772094617,1.,-1.11330807582542));
#31523=CARTESIAN_POINT('Ctrl Pts',(1.75699720772089,1.,-1.11858293216752));
#31524=CARTESIAN_POINT('Ctrl Pts',(1.76028671825084,1.,-1.12389096855078));
#31525=CARTESIAN_POINT('Ctrl Pts',(1.76354571966171,1.,-1.12923123555076));
#31526=CARTESIAN_POINT('Ctrl Pts',(1.76677384551883,1.,-1.13460291804635));
#31527=CARTESIAN_POINT('Ctrl Pts',(1.76997111386806,1.,-1.14000548337));
#31528=CARTESIAN_POINT('Ctrl Pts',(1.77313777896234,1.,-1.14543858226948));
#31529=CARTESIAN_POINT('Ctrl Pts',(1.77627422557034,1.,-1.15090197841531));
#31530=CARTESIAN_POINT('Ctrl Pts',(1.77938085564261,1.,-1.15639547194689));
#31531=CARTESIAN_POINT('Ctrl Pts',(1.78245795880949,1.,-1.16191881298458));
#31532=CARTESIAN_POINT('Ctrl Pts',(1.78550566040349,1.,-1.16747166312239));
#31533=CARTESIAN_POINT('Ctrl Pts',(1.78852398877523,1.,-1.17305363177265));
#31534=CARTESIAN_POINT('Ctrl Pts',(1.79151291552646,1.,-1.17866429440781));
#31535=CARTESIAN_POINT('Ctrl Pts',(1.79447240321572,1.,-1.18430321697471));
#31536=CARTESIAN_POINT('Ctrl Pts',(1.79740245923649,1.,-1.1899699793456));
#31537=CARTESIAN_POINT('Ctrl Pts',(1.80030314370121,1.,-1.19566418930405));
#31538=CARTESIAN_POINT('Ctrl Pts',(1.8031745483882,1.,-1.2013854893912));
#31539=CARTESIAN_POINT('Ctrl Pts',(1.80601678480772,1.,-1.20713356605519));
#31540=CARTESIAN_POINT('Ctrl Pts',(1.80882996916931,1.,-1.2129081570818));
#31541=CARTESIAN_POINT('Ctrl Pts',(1.81161420806172,1.,-1.2187090610323));
#31542=CARTESIAN_POINT('Ctrl Pts',(1.81436959209778,1.,-1.22453613304507));
#31543=CARTESIAN_POINT('Ctrl Pts',(1.81655087183054,1.,-1.22921864890975));
#31544=CARTESIAN_POINT('Ctrl Pts',(1.81817389920914,1.,-1.23274224526804));
#31545=CARTESIAN_POINT('Ctrl Pts',(1.81925017193531,1.,-1.23509651170384));
#31546=CARTESIAN_POINT('Ctrl Pts',(1.81978687191668,1.,-1.23627494547115));
#31547=CARTESIAN_POINT('',(1.5055822144029,0.,-0.892032620296855));
#31548=CARTESIAN_POINT('Origin',(0.,0.,0.));
#31549=CARTESIAN_POINT('',(1.60662857109684,1.,-0.693717979106306));
#31550=CARTESIAN_POINT('Origin',(0.,1.,0.));
#31551=CARTESIAN_POINT('',(1.60662857109684,0.,-0.693717979106308));
#31552=CARTESIAN_POINT('Ctrl Pts',(2.0698113262342,-1.,-0.745574324794401));
#31553=CARTESIAN_POINT('Ctrl Pts',(2.0698113262342,1.,-0.745574324794401));
#31554=CARTESIAN_POINT('Ctrl Pts',(2.06854248895728,-1.,-0.745832791378367));
#31555=CARTESIAN_POINT('Ctrl Pts',(2.06854248895728,1.,-0.745832791378367));
#31556=CARTESIAN_POINT('Ctrl Pts',(2.06600523016815,-1.,-0.746345871544201));
#31557=CARTESIAN_POINT('Ctrl Pts',(2.06600523016815,1.,-0.746345871544201));
#31558=CARTESIAN_POINT('Ctrl Pts',(2.06220058927826,-1.,-0.74710393278792));
#31559=CARTESIAN_POINT('Ctrl Pts',(2.06220058927826,1.,-0.74710393278792));
#31560=CARTESIAN_POINT('Ctrl Pts',(2.05713023031006,-1.,-0.748091554183803));
#31561=CARTESIAN_POINT('Ctrl Pts',(2.05713023031006,1.,-0.748091554183803));
#31562=CARTESIAN_POINT('Ctrl Pts',(2.05079645592154,-1.,-0.749287468665046));
#31563=CARTESIAN_POINT('Ctrl Pts',(2.05079645592154,1.,-0.749287468665046));
#31564=CARTESIAN_POINT('Ctrl Pts',(2.04446689147979,-1.,-0.750444657875576));
#31565=CARTESIAN_POINT('Ctrl Pts',(2.04446689147979,1.,-0.750444657875576));
#31566=CARTESIAN_POINT('Ctrl Pts',(2.03814160092099,-1.,-0.751562963361115));
#31567=CARTESIAN_POINT('Ctrl Pts',(2.03814160092099,1.,-0.751562963361115));
#31568=CARTESIAN_POINT('Ctrl Pts',(2.03182068456221,-1.,-0.752642180487211));
#31569=CARTESIAN_POINT('Ctrl Pts',(2.03182068456221,1.,-0.752642180487211));
#31570=CARTESIAN_POINT('Ctrl Pts',(2.02550428623313,-1.,-0.753682061112768));
#31571=CARTESIAN_POINT('Ctrl Pts',(2.02550428623313,1.,-0.753682061112768));
#31572=CARTESIAN_POINT('Ctrl Pts',(2.01919259405809,-1.,-0.754682330722816));
#31573=CARTESIAN_POINT('Ctrl Pts',(2.01919259405809,1.,-0.754682330722816));
#31574=CARTESIAN_POINT('Ctrl Pts',(2.01288584328084,-1.,-0.755642704957865));
#31575=CARTESIAN_POINT('Ctrl Pts',(2.01288584328084,1.,-0.755642704957865));
#31576=CARTESIAN_POINT('Ctrl Pts',(2.0065843158773,-1.,-0.756562904646671));
#31577=CARTESIAN_POINT('Ctrl Pts',(2.0065843158773,1.,-0.756562904646671));
#31578=CARTESIAN_POINT('Ctrl Pts',(2.00028834739178,-1.,-0.757442676862724));
#31579=CARTESIAN_POINT('Ctrl Pts',(2.00028834739178,1.,-0.757442676862724));
#31580=CARTESIAN_POINT('Ctrl Pts',(1.99399831098817,-1.,-0.758281796766761));
#31581=CARTESIAN_POINT('Ctrl Pts',(1.99399831098817,1.,-0.758281796766761));
#31582=CARTESIAN_POINT('Ctrl Pts',(1.98771456680874,-1.,-0.759080037802488));
#31583=CARTESIAN_POINT('Ctrl Pts',(1.98771456680874,1.,-0.759080037802488));
#31584=CARTESIAN_POINT('Ctrl Pts',(1.98143741418172,-1.,-0.75983714745219));
#31585=CARTESIAN_POINT('Ctrl Pts',(1.98143741418172,1.,-0.75983714745219));
#31586=CARTESIAN_POINT('Ctrl Pts',(1.97516705321494,-1.,-0.760552825409757));
#31587=CARTESIAN_POINT('Ctrl Pts',(1.97516705321494,1.,-0.760552825409757));
#31588=CARTESIAN_POINT('Ctrl Pts',(1.96890351582499,-1.,-0.761226690483821));
#31589=CARTESIAN_POINT('Ctrl Pts',(1.96890351582499,1.,-0.761226690483821));
#31590=CARTESIAN_POINT('Ctrl Pts',(1.96264672744186,-1.,-0.761858300014424));
#31591=CARTESIAN_POINT('Ctrl Pts',(1.96264672744186,1.,-0.761858300014424));
#31592=CARTESIAN_POINT('Ctrl Pts',(1.95639665309869,-1.,-0.762447203806179));
#31593=CARTESIAN_POINT('Ctrl Pts',(1.95639665309869,1.,-0.762447203806179));
#31594=CARTESIAN_POINT('Ctrl Pts',(1.95015342590024,-1.,-0.762992990878769));
#31595=CARTESIAN_POINT('Ctrl Pts',(1.95015342590024,1.,-0.762992990878769));
#31596=CARTESIAN_POINT('Ctrl Pts',(1.9439174661764,-1.,-0.763495333538629));
#31597=CARTESIAN_POINT('Ctrl Pts',(1.9439174661764,1.,-0.763495333538629));
#31598=CARTESIAN_POINT('Ctrl Pts',(1.93768964875886,-1.,-0.763954049121459));
#31599=CARTESIAN_POINT('Ctrl Pts',(1.93768964875886,1.,-0.763954049121459));
#31600=CARTESIAN_POINT('Ctrl Pts',(1.93147105496382,-1.,-0.764369010673941));
#31601=CARTESIAN_POINT('Ctrl Pts',(1.93147105496382,1.,-0.764369010673941));
#31602=CARTESIAN_POINT('Ctrl Pts',(1.92526263537048,-1.,-0.764740025488212));
#31603=CARTESIAN_POINT('Ctrl Pts',(1.92526263537048,1.,-0.764740025488212));
#31604=CARTESIAN_POINT('Ctrl Pts',(1.91906491634196,-1.,-0.765066729667089));
#31605=CARTESIAN_POINT('Ctrl Pts',(1.91906491634196,1.,-0.765066729667089));
#31606=CARTESIAN_POINT('Ctrl Pts',(1.91287765805169,-1.,-0.765348465884722));
#31607=CARTESIAN_POINT('Ctrl Pts',(1.91287765805169,1.,-0.765348465884722));
#31608=CARTESIAN_POINT('Ctrl Pts',(1.90669961402356,-1.,-0.765584196937919));
#31609=CARTESIAN_POINT('Ctrl Pts',(1.90669961402356,1.,-0.765584196937919));
#31610=CARTESIAN_POINT('Ctrl Pts',(1.90052930393596,-1.,-0.765772772593386));
#31611=CARTESIAN_POINT('Ctrl Pts',(1.90052930393596,1.,-0.765772772593386));
#31612=CARTESIAN_POINT('Ctrl Pts',(1.89436577771388,-1.,-0.765913193856978));
#31613=CARTESIAN_POINT('Ctrl Pts',(1.89436577771388,1.,-0.765913193856978));
#31614=CARTESIAN_POINT('Ctrl Pts',(1.88820926433409,-1.,-0.766004837062091));
#31615=CARTESIAN_POINT('Ctrl Pts',(1.88820926433409,1.,-0.766004837062091));
#31616=CARTESIAN_POINT('Ctrl Pts',(1.88206215302561,-1.,-0.766047794851865));
#31617=CARTESIAN_POINT('Ctrl Pts',(1.88206215302561,1.,-0.766047794851865));
#31618=CARTESIAN_POINT('Ctrl Pts',(1.87592888967883,-1.,-0.766042837036744));
#31619=CARTESIAN_POINT('Ctrl Pts',(1.87592888967883,1.,-0.766042837036744));
#31620=CARTESIAN_POINT('Ctrl Pts',(1.86981398314341,-1.,-0.765990708546091));
#31621=CARTESIAN_POINT('Ctrl Pts',(1.86981398314341,1.,-0.765990708546091));
#31622=CARTESIAN_POINT('Ctrl Pts',(1.86372027063312,-1.,-0.765891519092547));
#31623=CARTESIAN_POINT('Ctrl Pts',(1.86372027063312,1.,-0.765891519092547));
#31624=CARTESIAN_POINT('Ctrl Pts',(1.85764741390394,-1.,-0.765744212909319));
#31625=CARTESIAN_POINT('Ctrl Pts',(1.85764741390394,1.,-0.765744212909319));
#31626=CARTESIAN_POINT('Ctrl Pts',(1.85158945130063,-1.,-0.765545710619063));
#31627=CARTESIAN_POINT('Ctrl Pts',(1.85158945130063,1.,-0.765545710619063));
#31628=CARTESIAN_POINT('Ctrl Pts',(1.84553698875924,-1.,-0.765291664862029));
#31629=CARTESIAN_POINT('Ctrl Pts',(1.84553698875924,1.,-0.765291664862029));
#31630=CARTESIAN_POINT('Ctrl Pts',(1.83948181064835,-1.,-0.764978057881738));
#31631=CARTESIAN_POINT('Ctrl Pts',(1.83948181064835,1.,-0.764978057881738));
#31632=CARTESIAN_POINT('Ctrl Pts',(1.83342077227142,-1.,-0.764602549687853));
#31633=CARTESIAN_POINT('Ctrl Pts',(1.83342077227142,1.,-0.764602549687853));
#31634=CARTESIAN_POINT('Ctrl Pts',(1.82735991200065,-1.,-0.764165902605995));
#31635=CARTESIAN_POINT('Ctrl Pts',(1.82735991200065,1.,-0.764165902605995));
#31636=CARTESIAN_POINT('Ctrl Pts',(1.82131873145266,-1.,-0.763673465462727));
#31637=CARTESIAN_POINT('Ctrl Pts',(1.82131873145266,1.,-0.763673465462727));
#31638=CARTESIAN_POINT('Ctrl Pts',(1.8153211840553,-1.,-0.763132003836634));
#31639=CARTESIAN_POINT('Ctrl Pts',(1.8153211840553,1.,-0.763132003836634));
#31640=CARTESIAN_POINT('Ctrl Pts',(1.80938551463965,-1.,-0.762546129463938));
#31641=CARTESIAN_POINT('Ctrl Pts',(1.80938551463965,1.,-0.762546129463938));
#31642=CARTESIAN_POINT('Ctrl Pts',(1.80351583877342,-1.,-0.761915336443547));
#31643=CARTESIAN_POINT('Ctrl Pts',(1.80351583877342,1.,-0.761915336443547));
#31644=CARTESIAN_POINT('Ctrl Pts',(1.79768986997783,-1.,-0.761229695230558));
#31645=CARTESIAN_POINT('Ctrl Pts',(1.79768986997783,1.,-0.761229695230558));
#31646=CARTESIAN_POINT('Ctrl Pts',(1.7918581561088,-1.,-0.760469555880749));
#31647=CARTESIAN_POINT('Ctrl Pts',(1.7918581561088,1.,-0.760469555880749));
#31648=CARTESIAN_POINT('Ctrl Pts',(1.78596964884604,-1.,-0.75961440111019));
#31649=CARTESIAN_POINT('Ctrl Pts',(1.78596964884604,1.,-0.75961440111019));
#31650=CARTESIAN_POINT('Ctrl Pts',(1.77999411220945,-1.,-0.758650626677519));
#31651=CARTESIAN_POINT('Ctrl Pts',(1.77999411220945,1.,-0.758650626677519));
#31652=CARTESIAN_POINT('Ctrl Pts',(1.77394167108292,-1.,-0.757578264077029));
#31653=CARTESIAN_POINT('Ctrl Pts',(1.77394167108292,1.,-0.757578264077029));
#31654=CARTESIAN_POINT('Ctrl Pts',(1.76789396002998,-1.,-0.75642189602781));
#31655=CARTESIAN_POINT('Ctrl Pts',(1.76789396002998,1.,-0.75642189602781));
#31656=CARTESIAN_POINT('Ctrl Pts',(1.76197817240128,-1.,-0.755220979974462));
#31657=CARTESIAN_POINT('Ctrl Pts',(1.76197817240128,1.,-0.755220979974462));
#31658=CARTESIAN_POINT('Ctrl Pts',(1.75631083600019,-1.,-0.754009254027829));
#31659=CARTESIAN_POINT('Ctrl Pts',(1.75631083600019,1.,-0.754009254027829));
#31660=CARTESIAN_POINT('Ctrl Pts',(1.75095139468794,-1.,-0.752797683531314));
#31661=CARTESIAN_POINT('Ctrl Pts',(1.75095139468794,1.,-0.752797683531314));
#31662=CARTESIAN_POINT('Ctrl Pts',(1.74585086852502,-1.,-0.751555614164483));
#31663=CARTESIAN_POINT('Ctrl Pts',(1.74585086852502,1.,-0.751555614164483));
#31664=CARTESIAN_POINT('Ctrl Pts',(1.74080458267114,-1.,-0.75019343598125));
#31665=CARTESIAN_POINT('Ctrl Pts',(1.74080458267114,1.,-0.75019343598125));
#31666=CARTESIAN_POINT('Ctrl Pts',(1.7355035168033,-1.,-0.74858246295687));
#31667=CARTESIAN_POINT('Ctrl Pts',(1.7355035168033,1.,-0.74858246295687));
#31668=CARTESIAN_POINT('Ctrl Pts',(1.72958533647714,-1.,-0.746574710097752));
#31669=CARTESIAN_POINT('Ctrl Pts',(1.72958533647714,1.,-0.746574710097752));
#31670=CARTESIAN_POINT('Ctrl Pts',(1.72268229916769,-1.,-0.744021445433094));
#31671=CARTESIAN_POINT('Ctrl Pts',(1.72268229916769,1.,-0.744021445433094));
#31672=CARTESIAN_POINT('Ctrl Pts',(1.71447789751001,-1.,-0.74079516202821));
#31673=CARTESIAN_POINT('Ctrl Pts',(1.71447789751001,1.,-0.74079516202821));
#31674=CARTESIAN_POINT('Ctrl Pts',(1.70473309004249,-1.,-0.736799665716932));
#31675=CARTESIAN_POINT('Ctrl Pts',(1.70473309004249,1.,-0.736799665716932));
#31676=CARTESIAN_POINT('Ctrl Pts',(1.69326921972915,-1.,-0.731963238685357));
#31677=CARTESIAN_POINT('Ctrl Pts',(1.69326921972915,1.,-0.731963238685357));
#31678=CARTESIAN_POINT('Ctrl Pts',(1.67996158451922,-1.,-0.726235967982445));
#31679=CARTESIAN_POINT('Ctrl Pts',(1.67996158451922,1.,-0.726235967982445));
#31680=CARTESIAN_POINT('Ctrl Pts',(1.66472880551777,-1.,-0.71958543378795));
#31681=CARTESIAN_POINT('Ctrl Pts',(1.66472880551777,1.,-0.71958543378795));
#31682=CARTESIAN_POINT('Ctrl Pts',(1.64752408828442,-1.,-0.711993139340448));
#31683=CARTESIAN_POINT('Ctrl Pts',(1.64752408828442,1.,-0.711993139340448));
#31684=CARTESIAN_POINT('Ctrl Pts',(1.6321654166204,-1.,-0.705159151977294));
#31685=CARTESIAN_POINT('Ctrl Pts',(1.6321654166204,1.,-0.705159151977294));
#31686=CARTESIAN_POINT('Ctrl Pts',(1.61974673471117,-1.,-0.699605146398837));
#31687=CARTESIAN_POINT('Ctrl Pts',(1.61974673471117,1.,-0.699605146398837));
#31688=CARTESIAN_POINT('Ctrl Pts',(1.61106790957619,-1.,-0.69571209787897));
#31689=CARTESIAN_POINT('Ctrl Pts',(1.61106790957619,1.,-0.69571209787897));
#31690=CARTESIAN_POINT('Ctrl Pts',(1.60662857109684,-1.,-0.693717979106306));
#31691=CARTESIAN_POINT('Ctrl Pts',(1.60662857109684,1.,-0.693717979106306));
#31692=CARTESIAN_POINT('',(2.0698113262342,1.,-0.745574324794401));
#31693=CARTESIAN_POINT('Ctrl Pts',(2.0698113262342,1.,-0.745574324794401));
#31694=CARTESIAN_POINT('Ctrl Pts',(2.06854248895728,1.,-0.745832791378367));
#31695=CARTESIAN_POINT('Ctrl Pts',(2.06600523016815,1.,-0.746345871544201));
#31696=CARTESIAN_POINT('Ctrl Pts',(2.06220058927826,1.,-0.74710393278792));
#31697=CARTESIAN_POINT('Ctrl Pts',(2.05713023031006,1.,-0.748091554183803));
#31698=CARTESIAN_POINT('Ctrl Pts',(2.05079645592154,1.,-0.749287468665046));
#31699=CARTESIAN_POINT('Ctrl Pts',(2.04446689147979,1.,-0.750444657875576));
#31700=CARTESIAN_POINT('Ctrl Pts',(2.03814160092099,1.,-0.751562963361115));
#31701=CARTESIAN_POINT('Ctrl Pts',(2.03182068456221,1.,-0.752642180487211));
#31702=CARTESIAN_POINT('Ctrl Pts',(2.02550428623313,1.,-0.753682061112768));
#31703=CARTESIAN_POINT('Ctrl Pts',(2.01919259405809,1.,-0.754682330722816));
#31704=CARTESIAN_POINT('Ctrl Pts',(2.01288584328084,1.,-0.755642704957865));
#31705=CARTESIAN_POINT('Ctrl Pts',(2.0065843158773,1.,-0.756562904646671));
#31706=CARTESIAN_POINT('Ctrl Pts',(2.00028834739178,1.,-0.757442676862724));
#31707=CARTESIAN_POINT('Ctrl Pts',(1.99399831098817,1.,-0.758281796766761));
#31708=CARTESIAN_POINT('Ctrl Pts',(1.98771456680874,1.,-0.759080037802488));
#31709=CARTESIAN_POINT('Ctrl Pts',(1.98143741418172,1.,-0.75983714745219));
#31710=CARTESIAN_POINT('Ctrl Pts',(1.97516705321494,1.,-0.760552825409757));
#31711=CARTESIAN_POINT('Ctrl Pts',(1.96890351582499,1.,-0.761226690483821));
#31712=CARTESIAN_POINT('Ctrl Pts',(1.96264672744186,1.,-0.761858300014424));
#31713=CARTESIAN_POINT('Ctrl Pts',(1.95639665309869,1.,-0.762447203806179));
#31714=CARTESIAN_POINT('Ctrl Pts',(1.95015342590024,1.,-0.762992990878769));
#31715=CARTESIAN_POINT('Ctrl Pts',(1.9439174661764,1.,-0.763495333538629));
#31716=CARTESIAN_POINT('Ctrl Pts',(1.93768964875886,1.,-0.763954049121459));
#31717=CARTESIAN_POINT('Ctrl Pts',(1.93147105496382,1.,-0.764369010673941));
#31718=CARTESIAN_POINT('Ctrl Pts',(1.92526263537048,1.,-0.764740025488212));
#31719=CARTESIAN_POINT('Ctrl Pts',(1.91906491634196,1.,-0.765066729667089));
#31720=CARTESIAN_POINT('Ctrl Pts',(1.91287765805169,1.,-0.765348465884722));
#31721=CARTESIAN_POINT('Ctrl Pts',(1.90669961402356,1.,-0.765584196937919));
#31722=CARTESIAN_POINT('Ctrl Pts',(1.90052930393596,1.,-0.765772772593386));
#31723=CARTESIAN_POINT('Ctrl Pts',(1.89436577771388,1.,-0.765913193856978));
#31724=CARTESIAN_POINT('Ctrl Pts',(1.88820926433409,1.,-0.766004837062091));
#31725=CARTESIAN_POINT('Ctrl Pts',(1.88206215302561,1.,-0.766047794851865));
#31726=CARTESIAN_POINT('Ctrl Pts',(1.87592888967883,1.,-0.766042837036744));
#31727=CARTESIAN_POINT('Ctrl Pts',(1.86981398314341,1.,-0.765990708546091));
#31728=CARTESIAN_POINT('Ctrl Pts',(1.86372027063312,1.,-0.765891519092547));
#31729=CARTESIAN_POINT('Ctrl Pts',(1.85764741390394,1.,-0.765744212909319));
#31730=CARTESIAN_POINT('Ctrl Pts',(1.85158945130063,1.,-0.765545710619063));
#31731=CARTESIAN_POINT('Ctrl Pts',(1.84553698875924,1.,-0.765291664862029));
#31732=CARTESIAN_POINT('Ctrl Pts',(1.83948181064835,1.,-0.764978057881738));
#31733=CARTESIAN_POINT('Ctrl Pts',(1.83342077227142,1.,-0.764602549687853));
#31734=CARTESIAN_POINT('Ctrl Pts',(1.82735991200065,1.,-0.764165902605995));
#31735=CARTESIAN_POINT('Ctrl Pts',(1.82131873145266,1.,-0.763673465462727));
#31736=CARTESIAN_POINT('Ctrl Pts',(1.8153211840553,1.,-0.763132003836634));
#31737=CARTESIAN_POINT('Ctrl Pts',(1.80938551463965,1.,-0.762546129463938));
#31738=CARTESIAN_POINT('Ctrl Pts',(1.80351583877342,1.,-0.761915336443547));
#31739=CARTESIAN_POINT('Ctrl Pts',(1.79768986997783,1.,-0.761229695230558));
#31740=CARTESIAN_POINT('Ctrl Pts',(1.7918581561088,1.,-0.760469555880749));
#31741=CARTESIAN_POINT('Ctrl Pts',(1.78596964884604,1.,-0.75961440111019));
#31742=CARTESIAN_POINT('Ctrl Pts',(1.77999411220945,1.,-0.758650626677519));
#31743=CARTESIAN_POINT('Ctrl Pts',(1.77394167108292,1.,-0.757578264077029));
#31744=CARTESIAN_POINT('Ctrl Pts',(1.76789396002998,1.,-0.75642189602781));
#31745=CARTESIAN_POINT('Ctrl Pts',(1.76197817240128,1.,-0.755220979974462));
#31746=CARTESIAN_POINT('Ctrl Pts',(1.75631083600019,1.,-0.754009254027829));
#31747=CARTESIAN_POINT('Ctrl Pts',(1.75095139468794,1.,-0.752797683531314));
#31748=CARTESIAN_POINT('Ctrl Pts',(1.74585086852502,1.,-0.751555614164483));
#31749=CARTESIAN_POINT('Ctrl Pts',(1.74080458267114,1.,-0.75019343598125));
#31750=CARTESIAN_POINT('Ctrl Pts',(1.7355035168033,1.,-0.74858246295687));
#31751=CARTESIAN_POINT('Ctrl Pts',(1.72958533647714,1.,-0.746574710097752));
#31752=CARTESIAN_POINT('Ctrl Pts',(1.72268229916769,1.,-0.744021445433094));
#31753=CARTESIAN_POINT('Ctrl Pts',(1.71447789751001,1.,-0.74079516202821));
#31754=CARTESIAN_POINT('Ctrl Pts',(1.70473309004249,1.,-0.736799665716932));
#31755=CARTESIAN_POINT('Ctrl Pts',(1.69326921972915,1.,-0.731963238685357));
#31756=CARTESIAN_POINT('Ctrl Pts',(1.67996158451922,1.,-0.726235967982445));
#31757=CARTESIAN_POINT('Ctrl Pts',(1.66472880551777,1.,-0.71958543378795));
#31758=CARTESIAN_POINT('Ctrl Pts',(1.64752408828442,1.,-0.711993139340448));
#31759=CARTESIAN_POINT('Ctrl Pts',(1.6321654166204,1.,-0.705159151977294));
#31760=CARTESIAN_POINT('Ctrl Pts',(1.61974673471117,1.,-0.699605146398837));
#31761=CARTESIAN_POINT('Ctrl Pts',(1.61106790957619,1.,-0.69571209787897));
#31762=CARTESIAN_POINT('Ctrl Pts',(1.60662857109684,1.,-0.693717979106306));
#31763=CARTESIAN_POINT('',(2.0698113262342,0.,-0.745574324794401));
#31764=CARTESIAN_POINT('Origin',(2.11275013067528,0.,-0.61342227326009));
#31765=CARTESIAN_POINT('',(2.11275013067528,1.,-0.61342227326009));
#31766=CARTESIAN_POINT('',(2.0698113262342,1.,-0.745574324794401));
#31767=CARTESIAN_POINT('',(2.11275013067528,0.,-0.61342227326009));
#31768=CARTESIAN_POINT('Ctrl Pts',(1.7075470150345,-1.,-0.383122945602004));
#31769=CARTESIAN_POINT('Ctrl Pts',(1.7075470150345,1.,-0.383122945602004));
#31770=CARTESIAN_POINT('Ctrl Pts',(1.71231062891958,-1.,-0.384119047315542));
#31771=CARTESIAN_POINT('Ctrl Pts',(1.71231062891958,1.,-0.384119047315542));
#31772=CARTESIAN_POINT('Ctrl Pts',(1.72162022246158,-1.,-0.38607079032701));
#31773=CARTESIAN_POINT('Ctrl Pts',(1.72162022246158,1.,-0.38607079032701));
#31774=CARTESIAN_POINT('Ctrl Pts',(1.7349317097561,-1.,-0.388877023509192));
#31775=CARTESIAN_POINT('Ctrl Pts',(1.7349317097561,1.,-0.388877023509192));
#31776=CARTESIAN_POINT('Ctrl Pts',(1.75137405313962,-1.,-0.392375812294307));
#31777=CARTESIAN_POINT('Ctrl Pts',(1.75137405313962,1.,-0.392375812294307));
#31778=CARTESIAN_POINT('Ctrl Pts',(1.7697556004756,-1.,-0.39634619612042));
#31779=CARTESIAN_POINT('Ctrl Pts',(1.7697556004756,1.,-0.39634619612042));
#31780=CARTESIAN_POINT('Ctrl Pts',(1.78598826347533,-1.,-0.399919403783081));
#31781=CARTESIAN_POINT('Ctrl Pts',(1.78598826347533,1.,-0.399919403783081));
#31782=CARTESIAN_POINT('Ctrl Pts',(1.80012077176221,-1.,-0.403107976170441));
#31783=CARTESIAN_POINT('Ctrl Pts',(1.80012077176221,1.,-0.403107976170441));
#31784=CARTESIAN_POINT('Ctrl Pts',(1.81223801813988,-1.,-0.405933518411838));
#31785=CARTESIAN_POINT('Ctrl Pts',(1.81223801813988,1.,-0.405933518411838));
#31786=CARTESIAN_POINT('Ctrl Pts',(1.8224702267854,-1.,-0.408428948108534));
#31787=CARTESIAN_POINT('Ctrl Pts',(1.8224702267854,1.,-0.408428948108534));
#31788=CARTESIAN_POINT('Ctrl Pts',(1.83100408895216,-1.,-0.410641256301675));
#31789=CARTESIAN_POINT('Ctrl Pts',(1.83100408895216,1.,-0.410641256301675));
#31790=CARTESIAN_POINT('Ctrl Pts',(1.83808953475839,-1.,-0.412633125322162));
#31791=CARTESIAN_POINT('Ctrl Pts',(1.83808953475839,1.,-0.412633125322162));
#31792=CARTESIAN_POINT('Ctrl Pts',(1.8440575707371,-1.,-0.41448743825434));
#31793=CARTESIAN_POINT('Ctrl Pts',(1.8440575707371,1.,-0.41448743825434));
#31794=CARTESIAN_POINT('Ctrl Pts',(1.84929312929882,-1.,-0.416300022038864));
#31795=CARTESIAN_POINT('Ctrl Pts',(1.84929312929882,1.,-0.416300022038864));
#31796=CARTESIAN_POINT('Ctrl Pts',(1.85417632856234,-1.,-0.418164129143534));
#31797=CARTESIAN_POINT('Ctrl Pts',(1.85417632856234,1.,-0.418164129143534));
#31798=CARTESIAN_POINT('Ctrl Pts',(1.85903281096686,-1.,-0.42015728797562));
#31799=CARTESIAN_POINT('Ctrl Pts',(1.85903281096686,1.,-0.42015728797562));
#31800=CARTESIAN_POINT('Ctrl Pts',(1.86408083334028,-1.,-0.422327307418275));
#31801=CARTESIAN_POINT('Ctrl Pts',(1.86408083334028,1.,-0.422327307418275));
#31802=CARTESIAN_POINT('Ctrl Pts',(1.86937803944323,-1.,-0.424678177291359));
#31803=CARTESIAN_POINT('Ctrl Pts',(1.86937803944323,1.,-0.424678177291359));
#31804=CARTESIAN_POINT('Ctrl Pts',(1.87486989291484,-1.,-0.427183828519102));
#31805=CARTESIAN_POINT('Ctrl Pts',(1.87486989291484,1.,-0.427183828519102));
#31806=CARTESIAN_POINT('Ctrl Pts',(1.88044229001832,-1.,-0.429803062482345));
#31807=CARTESIAN_POINT('Ctrl Pts',(1.88044229001832,1.,-0.429803062482345));
#31808=CARTESIAN_POINT('Ctrl Pts',(1.88596913666793,-1.,-0.432493038548748));
#31809=CARTESIAN_POINT('Ctrl Pts',(1.88596913666793,1.,-0.432493038548748));
#31810=CARTESIAN_POINT('Ctrl Pts',(1.89136993975504,-1.,-0.435225660963383));
#31811=CARTESIAN_POINT('Ctrl Pts',(1.89136993975504,1.,-0.435225660963383));
#31812=CARTESIAN_POINT('Ctrl Pts',(1.89663648956466,-1.,-0.437995003948244));
#31813=CARTESIAN_POINT('Ctrl Pts',(1.89663648956466,1.,-0.437995003948244));
#31814=CARTESIAN_POINT('Ctrl Pts',(1.90180124389086,-1.,-0.440807833704038));
#31815=CARTESIAN_POINT('Ctrl Pts',(1.90180124389086,1.,-0.440807833704038));
#31816=CARTESIAN_POINT('Ctrl Pts',(1.90691756144898,-1.,-0.443677556849151));
#31817=CARTESIAN_POINT('Ctrl Pts',(1.90691756144898,1.,-0.443677556849151));
#31818=CARTESIAN_POINT('Ctrl Pts',(1.9120369998112,-1.,-0.446617343485711));
#31819=CARTESIAN_POINT('Ctrl Pts',(1.9120369998112,1.,-0.446617343485711));
#31820=CARTESIAN_POINT('Ctrl Pts',(1.91718342555755,-1.,-0.449632260106662));
#31821=CARTESIAN_POINT('Ctrl Pts',(1.91718342555755,1.,-0.449632260106662));
#31822=CARTESIAN_POINT('Ctrl Pts',(1.92235380648502,-1.,-0.452719478359433));
#31823=CARTESIAN_POINT('Ctrl Pts',(1.92235380648502,1.,-0.452719478359433));
#31824=CARTESIAN_POINT('Ctrl Pts',(1.92753067150476,-1.,-0.455872005174371));
#31825=CARTESIAN_POINT('Ctrl Pts',(1.92753067150476,1.,-0.455872005174371));
#31826=CARTESIAN_POINT('Ctrl Pts',(1.93269066517934,-1.,-0.459081234547926));
#31827=CARTESIAN_POINT('Ctrl Pts',(1.93269066517934,1.,-0.459081234547926));
#31828=CARTESIAN_POINT('Ctrl Pts',(1.93781486640821,-1.,-0.462340031009057));
#31829=CARTESIAN_POINT('Ctrl Pts',(1.93781486640821,1.,-0.462340031009057));
#31830=CARTESIAN_POINT('Ctrl Pts',(1.9428979419619,-1.,-0.46564546202603));
#31831=CARTESIAN_POINT('Ctrl Pts',(1.9428979419619,1.,-0.46564546202603));
#31832=CARTESIAN_POINT('Ctrl Pts',(1.94794381136514,-1.,-0.468997482913135));
#31833=CARTESIAN_POINT('Ctrl Pts',(1.94794381136514,1.,-0.468997482913135));
#31834=CARTESIAN_POINT('Ctrl Pts',(1.95296148278133,-1.,-0.472397672264072));
#31835=CARTESIAN_POINT('Ctrl Pts',(1.95296148278133,1.,-0.472397672264072));
#31836=CARTESIAN_POINT('Ctrl Pts',(1.95796111148177,-1.,-0.475848034683176));
#31837=CARTESIAN_POINT('Ctrl Pts',(1.95796111148177,1.,-0.475848034683176));
#31838=CARTESIAN_POINT('Ctrl Pts',(1.96294933055943,-1.,-0.479349583074855));
#31839=CARTESIAN_POINT('Ctrl Pts',(1.96294933055943,1.,-0.479349583074855));
#31840=CARTESIAN_POINT('Ctrl Pts',(1.96792703422362,-1.,-0.482901662120691));
#31841=CARTESIAN_POINT('Ctrl Pts',(1.96792703422362,1.,-0.482901662120691));
#31842=CARTESIAN_POINT('Ctrl Pts',(1.97289186263272,-1.,-0.486502692907659));
#31843=CARTESIAN_POINT('Ctrl Pts',(1.97289186263272,1.,-0.486502692907659));
#31844=CARTESIAN_POINT('Ctrl Pts',(1.97783973019229,-1.,-0.490150627860953));
#31845=CARTESIAN_POINT('Ctrl Pts',(1.97783973019229,1.,-0.490150627860953));
#31846=CARTESIAN_POINT('Ctrl Pts',(1.98276658761821,-1.,-0.493843476541495));
#31847=CARTESIAN_POINT('Ctrl Pts',(1.98276658761821,1.,-0.493843476541495));
#31848=CARTESIAN_POINT('Ctrl Pts',(1.98767044752932,-1.,-0.497579909545574));
#31849=CARTESIAN_POINT('Ctrl Pts',(1.98767044752932,1.,-0.497579909545574));
#31850=CARTESIAN_POINT('Ctrl Pts',(1.99255149126155,-1.,-0.501359287727146));
#31851=CARTESIAN_POINT('Ctrl Pts',(1.99255149126155,1.,-0.501359287727146));
#31852=CARTESIAN_POINT('Ctrl Pts',(1.99741107463572,-1.,-0.505181361323026));
#31853=CARTESIAN_POINT('Ctrl Pts',(1.99741107463572,1.,-0.505181361323026));
#31854=CARTESIAN_POINT('Ctrl Pts',(2.00225107134734,-1.,-0.509046069886157));
#31855=CARTESIAN_POINT('Ctrl Pts',(2.00225107134734,1.,-0.509046069886157));
#31856=CARTESIAN_POINT('Ctrl Pts',(2.00707309946949,-1.,-0.512953306961793));
#31857=CARTESIAN_POINT('Ctrl Pts',(2.00707309946949,1.,-0.512953306961793));
#31858=CARTESIAN_POINT('Ctrl Pts',(2.01187773939242,-1.,-0.516902681728687));
#31859=CARTESIAN_POINT('Ctrl Pts',(2.01187773939242,1.,-0.516902681728687));
#31860=CARTESIAN_POINT('Ctrl Pts',(2.01666477917286,-1.,-0.520893590399371));
#31861=CARTESIAN_POINT('Ctrl Pts',(2.01666477917286,1.,-0.520893590399371));
#31862=CARTESIAN_POINT('Ctrl Pts',(2.02143356304698,-1.,-0.524925318333476));
#31863=CARTESIAN_POINT('Ctrl Pts',(2.02143356304698,1.,-0.524925318333476));
#31864=CARTESIAN_POINT('Ctrl Pts',(2.0261832908329,-1.,-0.528997127241914));
#31865=CARTESIAN_POINT('Ctrl Pts',(2.0261832908329,1.,-0.528997127241914));
#31866=CARTESIAN_POINT('Ctrl Pts',(2.03091336214426,-1.,-0.533108355132977));
#31867=CARTESIAN_POINT('Ctrl Pts',(2.03091336214426,1.,-0.533108355132977));
#31868=CARTESIAN_POINT('Ctrl Pts',(2.03562362954037,-1.,-0.537258489833262));
#31869=CARTESIAN_POINT('Ctrl Pts',(2.03562362954037,1.,-0.537258489833262));
#31870=CARTESIAN_POINT('Ctrl Pts',(2.04031422690527,-1.,-0.541447120615659));
#31871=CARTESIAN_POINT('Ctrl Pts',(2.04031422690527,1.,-0.541447120615659));
#31872=CARTESIAN_POINT('Ctrl Pts',(2.04498544714588,-1.,-0.54567390381743));
#31873=CARTESIAN_POINT('Ctrl Pts',(2.04498544714588,1.,-0.54567390381743));
#31874=CARTESIAN_POINT('Ctrl Pts',(2.04963761077958,-1.,-0.549938525150295));
#31875=CARTESIAN_POINT('Ctrl Pts',(2.04963761077958,1.,-0.549938525150295));
#31876=CARTESIAN_POINT('Ctrl Pts',(2.05427091604413,-1.,-0.554240657463906));
#31877=CARTESIAN_POINT('Ctrl Pts',(2.05427091604413,1.,-0.554240657463906));
#31878=CARTESIAN_POINT('Ctrl Pts',(2.05888537756462,-1.,-0.558579940185152));
#31879=CARTESIAN_POINT('Ctrl Pts',(2.05888537756462,1.,-0.558579940185152));
#31880=CARTESIAN_POINT('Ctrl Pts',(2.06348090160589,-1.,-0.562955993082262));
#31881=CARTESIAN_POINT('Ctrl Pts',(2.06348090160589,1.,-0.562955993082262));
#31882=CARTESIAN_POINT('Ctrl Pts',(2.06805732997334,-1.,-0.567368421181087));
#31883=CARTESIAN_POINT('Ctrl Pts',(2.06805732997334,1.,-0.567368421181087));
#31884=CARTESIAN_POINT('Ctrl Pts',(2.07261449292824,-1.,-0.571816823242603));
#31885=CARTESIAN_POINT('Ctrl Pts',(2.07261449292824,1.,-0.571816823242603));
#31886=CARTESIAN_POINT('Ctrl Pts',(2.07715226767559,-1.,-0.576300797416845));
#31887=CARTESIAN_POINT('Ctrl Pts',(2.07715226767559,1.,-0.576300797416845));
#31888=CARTESIAN_POINT('Ctrl Pts',(2.08167059018418,-1.,-0.580819952108064));
#31889=CARTESIAN_POINT('Ctrl Pts',(2.08167059018418,1.,-0.580819952108064));
#31890=CARTESIAN_POINT('Ctrl Pts',(2.08616943727951,-1.,-0.585373918991617));
#31891=CARTESIAN_POINT('Ctrl Pts',(2.08616943727951,1.,-0.585373918991617));
#31892=CARTESIAN_POINT('Ctrl Pts',(2.09064881812129,-1.,-0.589962365403406));
#31893=CARTESIAN_POINT('Ctrl Pts',(2.09064881812129,1.,-0.589962365403406));
#31894=CARTESIAN_POINT('Ctrl Pts',(2.0951087622027,-1.,-0.594585006052162));
#31895=CARTESIAN_POINT('Ctrl Pts',(2.0951087622027,1.,-0.594585006052162));
#31896=CARTESIAN_POINT('Ctrl Pts',(2.0995493086477,-1.,-0.599241616420534));
#31897=CARTESIAN_POINT('Ctrl Pts',(2.0995493086477,1.,-0.599241616420534));
#31898=CARTESIAN_POINT('Ctrl Pts',(2.10397049886949,-1.,-0.60393203073603));
#31899=CARTESIAN_POINT('Ctrl Pts',(2.10397049886949,1.,-0.60393203073603));
#31900=CARTESIAN_POINT('Ctrl Pts',(2.1074919961518,-1.,-0.607711315454876));
#31901=CARTESIAN_POINT('Ctrl Pts',(2.1074919961518,1.,-0.607711315454876));
#31902=CARTESIAN_POINT('Ctrl Pts',(2.11012443807238,-1.,-0.610560911689899));
#31903=CARTESIAN_POINT('Ctrl Pts',(2.11012443807238,1.,-0.610560911689899));
#31904=CARTESIAN_POINT('Ctrl Pts',(2.11187554259986,-1.,-0.6124673655618));
#31905=CARTESIAN_POINT('Ctrl Pts',(2.11187554259986,1.,-0.6124673655618));
#31906=CARTESIAN_POINT('Ctrl Pts',(2.11275013067528,-1.,-0.61342227326009));
#31907=CARTESIAN_POINT('Ctrl Pts',(2.11275013067528,1.,-0.61342227326009));
#31908=CARTESIAN_POINT('',(1.7075470150345,1.,-0.383122945602004));
#31909=CARTESIAN_POINT('Ctrl Pts',(1.7075470150345,1.,-0.383122945602004));
#31910=CARTESIAN_POINT('Ctrl Pts',(1.71231062891958,1.,-0.384119047315542));
#31911=CARTESIAN_POINT('Ctrl Pts',(1.72162022246158,1.,-0.38607079032701));
#31912=CARTESIAN_POINT('Ctrl Pts',(1.7349317097561,1.,-0.388877023509192));
#31913=CARTESIAN_POINT('Ctrl Pts',(1.75137405313962,1.,-0.392375812294307));
#31914=CARTESIAN_POINT('Ctrl Pts',(1.7697556004756,1.,-0.39634619612042));
#31915=CARTESIAN_POINT('Ctrl Pts',(1.78598826347533,1.,-0.399919403783081));
#31916=CARTESIAN_POINT('Ctrl Pts',(1.80012077176221,1.,-0.403107976170441));
#31917=CARTESIAN_POINT('Ctrl Pts',(1.81223801813988,1.,-0.405933518411838));
#31918=CARTESIAN_POINT('Ctrl Pts',(1.8224702267854,1.,-0.408428948108534));
#31919=CARTESIAN_POINT('Ctrl Pts',(1.83100408895216,1.,-0.410641256301675));
#31920=CARTESIAN_POINT('Ctrl Pts',(1.83808953475839,1.,-0.412633125322162));
#31921=CARTESIAN_POINT('Ctrl Pts',(1.8440575707371,1.,-0.41448743825434));
#31922=CARTESIAN_POINT('Ctrl Pts',(1.84929312929882,1.,-0.416300022038864));
#31923=CARTESIAN_POINT('Ctrl Pts',(1.85417632856234,1.,-0.418164129143534));
#31924=CARTESIAN_POINT('Ctrl Pts',(1.85903281096686,1.,-0.42015728797562));
#31925=CARTESIAN_POINT('Ctrl Pts',(1.86408083334028,1.,-0.422327307418275));
#31926=CARTESIAN_POINT('Ctrl Pts',(1.86937803944323,1.,-0.424678177291359));
#31927=CARTESIAN_POINT('Ctrl Pts',(1.87486989291484,1.,-0.427183828519102));
#31928=CARTESIAN_POINT('Ctrl Pts',(1.88044229001832,1.,-0.429803062482345));
#31929=CARTESIAN_POINT('Ctrl Pts',(1.88596913666793,1.,-0.432493038548748));
#31930=CARTESIAN_POINT('Ctrl Pts',(1.89136993975504,1.,-0.435225660963383));
#31931=CARTESIAN_POINT('Ctrl Pts',(1.89663648956466,1.,-0.437995003948244));
#31932=CARTESIAN_POINT('Ctrl Pts',(1.90180124389086,1.,-0.440807833704038));
#31933=CARTESIAN_POINT('Ctrl Pts',(1.90691756144898,1.,-0.443677556849151));
#31934=CARTESIAN_POINT('Ctrl Pts',(1.9120369998112,1.,-0.446617343485711));
#31935=CARTESIAN_POINT('Ctrl Pts',(1.91718342555755,1.,-0.449632260106662));
#31936=CARTESIAN_POINT('Ctrl Pts',(1.92235380648502,1.,-0.452719478359433));
#31937=CARTESIAN_POINT('Ctrl Pts',(1.92753067150476,1.,-0.455872005174371));
#31938=CARTESIAN_POINT('Ctrl Pts',(1.93269066517934,1.,-0.459081234547926));
#31939=CARTESIAN_POINT('Ctrl Pts',(1.93781486640821,1.,-0.462340031009057));
#31940=CARTESIAN_POINT('Ctrl Pts',(1.9428979419619,1.,-0.46564546202603));
#31941=CARTESIAN_POINT('Ctrl Pts',(1.94794381136514,1.,-0.468997482913135));
#31942=CARTESIAN_POINT('Ctrl Pts',(1.95296148278133,1.,-0.472397672264072));
#31943=CARTESIAN_POINT('Ctrl Pts',(1.95796111148177,1.,-0.475848034683176));
#31944=CARTESIAN_POINT('Ctrl Pts',(1.96294933055943,1.,-0.479349583074855));
#31945=CARTESIAN_POINT('Ctrl Pts',(1.96792703422362,1.,-0.482901662120691));
#31946=CARTESIAN_POINT('Ctrl Pts',(1.97289186263272,1.,-0.486502692907659));
#31947=CARTESIAN_POINT('Ctrl Pts',(1.97783973019229,1.,-0.490150627860953));
#31948=CARTESIAN_POINT('Ctrl Pts',(1.98276658761821,1.,-0.493843476541495));
#31949=CARTESIAN_POINT('Ctrl Pts',(1.98767044752932,1.,-0.497579909545574));
#31950=CARTESIAN_POINT('Ctrl Pts',(1.99255149126155,1.,-0.501359287727146));
#31951=CARTESIAN_POINT('Ctrl Pts',(1.99741107463572,1.,-0.505181361323026));
#31952=CARTESIAN_POINT('Ctrl Pts',(2.00225107134734,1.,-0.509046069886157));
#31953=CARTESIAN_POINT('Ctrl Pts',(2.00707309946949,1.,-0.512953306961793));
#31954=CARTESIAN_POINT('Ctrl Pts',(2.01187773939242,1.,-0.516902681728687));
#31955=CARTESIAN_POINT('Ctrl Pts',(2.01666477917286,1.,-0.520893590399371));
#31956=CARTESIAN_POINT('Ctrl Pts',(2.02143356304698,1.,-0.524925318333476));
#31957=CARTESIAN_POINT('Ctrl Pts',(2.0261832908329,1.,-0.528997127241914));
#31958=CARTESIAN_POINT('Ctrl Pts',(2.03091336214426,1.,-0.533108355132977));
#31959=CARTESIAN_POINT('Ctrl Pts',(2.03562362954037,1.,-0.537258489833262));
#31960=CARTESIAN_POINT('Ctrl Pts',(2.04031422690527,1.,-0.541447120615659));
#31961=CARTESIAN_POINT('Ctrl Pts',(2.04498544714588,1.,-0.54567390381743));
#31962=CARTESIAN_POINT('Ctrl Pts',(2.04963761077958,1.,-0.549938525150295));
#31963=CARTESIAN_POINT('Ctrl Pts',(2.05427091604413,1.,-0.554240657463906));
#31964=CARTESIAN_POINT('Ctrl Pts',(2.05888537756462,1.,-0.558579940185152));
#31965=CARTESIAN_POINT('Ctrl Pts',(2.06348090160589,1.,-0.562955993082262));
#31966=CARTESIAN_POINT('Ctrl Pts',(2.06805732997334,1.,-0.567368421181087));
#31967=CARTESIAN_POINT('Ctrl Pts',(2.07261449292824,1.,-0.571816823242603));
#31968=CARTESIAN_POINT('Ctrl Pts',(2.07715226767559,1.,-0.576300797416845));
#31969=CARTESIAN_POINT('Ctrl Pts',(2.08167059018418,1.,-0.580819952108064));
#31970=CARTESIAN_POINT('Ctrl Pts',(2.08616943727951,1.,-0.585373918991617));
#31971=CARTESIAN_POINT('Ctrl Pts',(2.09064881812129,1.,-0.589962365403406));
#31972=CARTESIAN_POINT('Ctrl Pts',(2.0951087622027,1.,-0.594585006052162));
#31973=CARTESIAN_POINT('Ctrl Pts',(2.0995493086477,1.,-0.599241616420534));
#31974=CARTESIAN_POINT('Ctrl Pts',(2.10397049886949,1.,-0.60393203073603));
#31975=CARTESIAN_POINT('Ctrl Pts',(2.1074919961518,1.,-0.607711315454876));
#31976=CARTESIAN_POINT('Ctrl Pts',(2.11012443807238,1.,-0.610560911689899));
#31977=CARTESIAN_POINT('Ctrl Pts',(2.11187554259986,1.,-0.6124673655618));
#31978=CARTESIAN_POINT('Ctrl Pts',(2.11275013067528,1.,-0.61342227326009));
#31979=CARTESIAN_POINT('',(1.7075470150345,0.,-0.383122945602001));
#31980=CARTESIAN_POINT('Origin',(0.,0.,0.));
#31981=CARTESIAN_POINT('',(1.74236521665491,1.,-0.163289472382896));
#31982=CARTESIAN_POINT('Origin',(0.,1.,0.));
#31983=CARTESIAN_POINT('',(1.74236521665491,0.,-0.163289472382896));
#31984=CARTESIAN_POINT('Ctrl Pts',(2.19890268624765,-1.,-0.0694764450219582));
#31985=CARTESIAN_POINT('Ctrl Pts',(2.19890268624765,1.,-0.0694764450219582));
#31986=CARTESIAN_POINT('Ctrl Pts',(2.19777582085423,-1.,-0.0701143536325491));
#31987=CARTESIAN_POINT('Ctrl Pts',(2.19777582085423,1.,-0.0701143536325491));
#31988=CARTESIAN_POINT('Ctrl Pts',(2.19552129484002,-1.,-0.0713863779526155));
#31989=CARTESIAN_POINT('Ctrl Pts',(2.19552129484002,1.,-0.0713863779526155));
#31990=CARTESIAN_POINT('Ctrl Pts',(2.19213712013662,-1.,-0.0732830357306726));
#31991=CARTESIAN_POINT('Ctrl Pts',(2.19213712013662,1.,-0.0732830357306726));
#31992=CARTESIAN_POINT('Ctrl Pts',(2.1876201139953,-1.,-0.0757891465836149));
#31993=CARTESIAN_POINT('Ctrl Pts',(2.1876201139953,1.,-0.0757891465836149));
#31994=CARTESIAN_POINT('Ctrl Pts',(2.18196589448887,-1.,-0.0788837727685244));
#31995=CARTESIAN_POINT('Ctrl Pts',(2.18196589448887,1.,-0.0788837727685244));
#31996=CARTESIAN_POINT('Ctrl Pts',(2.176303712113,-1.,-0.0819402680872767));
#31997=CARTESIAN_POINT('Ctrl Pts',(2.176303712113,1.,-0.0819402680872767));
#31998=CARTESIAN_POINT('Ctrl Pts',(2.17063357870952,-1.,-0.0849584620835374));
#31999=CARTESIAN_POINT('Ctrl Pts',(2.17063357870952,1.,-0.0849584620835374));
#32000=CARTESIAN_POINT('Ctrl Pts',(2.16495552645014,-1.,-0.0879381291386924));
#32001=CARTESIAN_POINT('Ctrl Pts',(2.16495552645014,1.,-0.0879381291386924));
#32002=CARTESIAN_POINT('Ctrl Pts',(2.15926961544516,-1.,-0.0908789888107267));
#32003=CARTESIAN_POINT('Ctrl Pts',(2.15926961544516,1.,-0.0908789888107267));
#32004=CARTESIAN_POINT('Ctrl Pts',(2.1535759397817,-1.,-0.0937807218867645));
#32005=CARTESIAN_POINT('Ctrl Pts',(2.1535759397817,1.,-0.0937807218867645));
#32006=CARTESIAN_POINT('Ctrl Pts',(2.14787463531795,-1.,-0.096642985230546));
#32007=CARTESIAN_POINT('Ctrl Pts',(2.14787463531795,1.,-0.096642985230546));
#32008=CARTESIAN_POINT('Ctrl Pts',(2.14216588396025,-1.,-0.0994654261990917));
#32009=CARTESIAN_POINT('Ctrl Pts',(2.14216588396025,1.,-0.0994654261990917));
#32010=CARTESIAN_POINT('Ctrl Pts',(2.13644992667165,-1.,-0.102247700556101));
#32011=CARTESIAN_POINT('Ctrl Pts',(2.13644992667165,1.,-0.102247700556101));
#32012=CARTESIAN_POINT('Ctrl Pts',(2.13072704887293,-1.,-0.10498947915274));
#32013=CARTESIAN_POINT('Ctrl Pts',(2.13072704887293,1.,-0.10498947915274));
#32014=CARTESIAN_POINT('Ctrl Pts',(2.12499752307,-1.,-0.10769043523109));
#32015=CARTESIAN_POINT('Ctrl Pts',(2.12499752307,1.,-0.10769043523109));
#32016=CARTESIAN_POINT('Ctrl Pts',(2.11926155590865,-1.,-0.110350236135025));
#32017=CARTESIAN_POINT('Ctrl Pts',(2.11926155590865,1.,-0.110350236135025));
#32018=CARTESIAN_POINT('Ctrl Pts',(2.11351924490306,-1.,-0.112968534419737));
#32019=CARTESIAN_POINT('Ctrl Pts',(2.11351924490306,1.,-0.112968534419737));
#32020=CARTESIAN_POINT('Ctrl Pts',(2.10777050261309,-1.,-0.115544957687927));
#32021=CARTESIAN_POINT('Ctrl Pts',(2.10777050261309,1.,-0.115544957687927));
#32022=CARTESIAN_POINT('Ctrl Pts',(2.102015121329,-1.,-0.118079107988356));
#32023=CARTESIAN_POINT('Ctrl Pts',(2.102015121329,1.,-0.118079107988356));
#32024=CARTESIAN_POINT('Ctrl Pts',(2.0962529286773,-1.,-0.120570567965122));
#32025=CARTESIAN_POINT('Ctrl Pts',(2.0962529286773,1.,-0.120570567965122));
#32026=CARTESIAN_POINT('Ctrl Pts',(2.09048392424825,-1.,-0.123018905621083));
#32027=CARTESIAN_POINT('Ctrl Pts',(2.09048392424825,1.,-0.123018905621083));
#32028=CARTESIAN_POINT('Ctrl Pts',(2.08470840653643,-1.,-0.125423679412062));
#32029=CARTESIAN_POINT('Ctrl Pts',(2.08470840653643,1.,-0.125423679412062));
#32030=CARTESIAN_POINT('Ctrl Pts',(2.07892715110987,-1.,-0.12778444527612));
#32031=CARTESIAN_POINT('Ctrl Pts',(2.07892715110987,1.,-0.12778444527612));
#32032=CARTESIAN_POINT('Ctrl Pts',(2.07314114713063,-1.,-0.130100748328404));
#32033=CARTESIAN_POINT('Ctrl Pts',(2.07314114713063,1.,-0.130100748328404));
#32034=CARTESIAN_POINT('Ctrl Pts',(2.06735123910326,-1.,-0.132372111547711));
#32035=CARTESIAN_POINT('Ctrl Pts',(2.06735123910326,1.,-0.132372111547711));
#32036=CARTESIAN_POINT('Ctrl Pts',(2.06155781517842,-1.,-0.134598026192106));
#32037=CARTESIAN_POINT('Ctrl Pts',(2.06155781517842,1.,-0.134598026192106));
#32038=CARTESIAN_POINT('Ctrl Pts',(2.05576044414264,-1.,-0.136777941218044));
#32039=CARTESIAN_POINT('Ctrl Pts',(2.05576044414264,1.,-0.136777941218044));
#32040=CARTESIAN_POINT('Ctrl Pts',(2.04995762001328,-1.,-0.138911255368966));
#32041=CARTESIAN_POINT('Ctrl Pts',(2.04995762001328,1.,-0.138911255368966));
#32042=CARTESIAN_POINT('Ctrl Pts',(2.04414757947916,-1.,-0.140997332152546));
#32043=CARTESIAN_POINT('Ctrl Pts',(2.04414757947916,1.,-0.140997332152546));
#32044=CARTESIAN_POINT('Ctrl Pts',(2.03832911025912,-1.,-0.143035515058209));
#32045=CARTESIAN_POINT('Ctrl Pts',(2.03832911025912,1.,-0.143035515058209));
#32046=CARTESIAN_POINT('Ctrl Pts',(2.03250223739942,-1.,-0.145025140186058));
#32047=CARTESIAN_POINT('Ctrl Pts',(2.03250223739942,1.,-0.145025140186058));
#32048=CARTESIAN_POINT('Ctrl Pts',(2.02666926182017,-1.,-0.146965557332583));
#32049=CARTESIAN_POINT('Ctrl Pts',(2.02666926182017,1.,-0.146965557332583));
#32050=CARTESIAN_POINT('Ctrl Pts',(2.02083464969894,-1.,-0.148856124775337));
#32051=CARTESIAN_POINT('Ctrl Pts',(2.02083464969894,1.,-0.148856124775337));
#32052=CARTESIAN_POINT('Ctrl Pts',(2.01500291940238,-1.,-0.150696157673078));
#32053=CARTESIAN_POINT('Ctrl Pts',(2.01500291940238,1.,-0.150696157673078));
#32054=CARTESIAN_POINT('Ctrl Pts',(2.00917680318424,-1.,-0.15248488362145));
#32055=CARTESIAN_POINT('Ctrl Pts',(2.00917680318424,1.,-0.15248488362145));
#32056=CARTESIAN_POINT('Ctrl Pts',(2.00335565310543,-1.,-0.154221403049722));
#32057=CARTESIAN_POINT('Ctrl Pts',(2.00335565310543,1.,-0.154221403049722));
#32058=CARTESIAN_POINT('Ctrl Pts',(1.99753284771497,-1.,-0.155904629548784));
#32059=CARTESIAN_POINT('Ctrl Pts',(1.99753284771497,1.,-0.155904629548784));
#32060=CARTESIAN_POINT('Ctrl Pts',(1.99169810931908,-1.,-0.157533331459227));
#32061=CARTESIAN_POINT('Ctrl Pts',(1.99169810931908,1.,-0.157533331459227));
#32062=CARTESIAN_POINT('Ctrl Pts',(1.98584238283292,-1.,-0.159106226437299));
#32063=CARTESIAN_POINT('Ctrl Pts',(1.98584238283292,1.,-0.159106226437299));
#32064=CARTESIAN_POINT('Ctrl Pts',(1.97996195437559,-1.,-0.160622060784611));
#32065=CARTESIAN_POINT('Ctrl Pts',(1.97996195437559,1.,-0.160622060784611));
#32066=CARTESIAN_POINT('Ctrl Pts',(1.97406280235188,-1.,-0.162079693556289));
#32067=CARTESIAN_POINT('Ctrl Pts',(1.97406280235188,1.,-0.162079693556289));
#32068=CARTESIAN_POINT('Ctrl Pts',(1.96816512677967,-1.,-0.163478185457734));
#32069=CARTESIAN_POINT('Ctrl Pts',(1.96816512677967,1.,-0.163478185457734));
#32070=CARTESIAN_POINT('Ctrl Pts',(1.96229379940136,-1.,-0.164816568920269));
#32071=CARTESIAN_POINT('Ctrl Pts',(1.96229379940136,1.,-0.164816568920269));
#32072=CARTESIAN_POINT('Ctrl Pts',(1.9564675971873,-1.,-0.166093592002813));
#32073=CARTESIAN_POINT('Ctrl Pts',(1.9564675971873,1.,-0.166093592002813));
#32074=CARTESIAN_POINT('Ctrl Pts',(1.95069027794294,-1.,-0.167307501784476));
#32075=CARTESIAN_POINT('Ctrl Pts',(1.95069027794294,1.,-0.167307501784476));
#32076=CARTESIAN_POINT('Ctrl Pts',(1.94493757756931,-1.,-0.168455741607556));
#32077=CARTESIAN_POINT('Ctrl Pts',(1.94493757756931,1.,-0.168455741607556));
#32078=CARTESIAN_POINT('Ctrl Pts',(1.93915639211581,-1.,-0.169534904817491));
#32079=CARTESIAN_POINT('Ctrl Pts',(1.93915639211581,1.,-0.169534904817491));
#32080=CARTESIAN_POINT('Ctrl Pts',(1.93329183155539,-1.,-0.170541253116202));
#32081=CARTESIAN_POINT('Ctrl Pts',(1.93329183155539,1.,-0.170541253116202));
#32082=CARTESIAN_POINT('Ctrl Pts',(1.92731093582036,-1.,-0.171471191532988));
#32083=CARTESIAN_POINT('Ctrl Pts',(1.92731093582036,1.,-0.171471191532988));
#32084=CARTESIAN_POINT('Ctrl Pts',(1.9212233439798,-1.,-0.172321621259514));
#32085=CARTESIAN_POINT('Ctrl Pts',(1.9212233439798,1.,-0.172321621259514));
#32086=CARTESIAN_POINT('Ctrl Pts',(1.91511429159527,-1.,-0.173090695383496));
#32087=CARTESIAN_POINT('Ctrl Pts',(1.91511429159527,1.,-0.173090695383496));
#32088=CARTESIAN_POINT('Ctrl Pts',(1.90911693975267,-1.,-0.173776635257817));
#32089=CARTESIAN_POINT('Ctrl Pts',(1.90911693975267,1.,-0.173776635257817));
#32090=CARTESIAN_POINT('Ctrl Pts',(1.90335253862834,-1.,-0.174375518661085));
#32091=CARTESIAN_POINT('Ctrl Pts',(1.90335253862834,1.,-0.174375518661085));
#32092=CARTESIAN_POINT('Ctrl Pts',(1.89788101117132,-1.,-0.174879405091263));
#32093=CARTESIAN_POINT('Ctrl Pts',(1.89788101117132,1.,-0.174879405091263));
#32094=CARTESIAN_POINT('Ctrl Pts',(1.892646301985,-1.,-0.175274276190844));
#32095=CARTESIAN_POINT('Ctrl Pts',(1.892646301985,1.,-0.175274276190844));
#32096=CARTESIAN_POINT('Ctrl Pts',(1.88742606273259,-1.,-0.175538155840648));
#32097=CARTESIAN_POINT('Ctrl Pts',(1.88742606273259,1.,-0.175538155840648));
#32098=CARTESIAN_POINT('Ctrl Pts',(1.88188663145367,-1.,-0.175644148889699));
#32099=CARTESIAN_POINT('Ctrl Pts',(1.88188663145367,1.,-0.175644148889699));
#32100=CARTESIAN_POINT('Ctrl Pts',(1.87563767773588,-1.,-0.175563480746485));
#32101=CARTESIAN_POINT('Ctrl Pts',(1.87563767773588,1.,-0.175563480746485));
#32102=CARTESIAN_POINT('Ctrl Pts',(1.86828349694799,-1.,-0.175268337590758));
#32103=CARTESIAN_POINT('Ctrl Pts',(1.86828349694799,1.,-0.175268337590758));
#32104=CARTESIAN_POINT('Ctrl Pts',(1.85948367088837,-1.,-0.17473525927603));
#32105=CARTESIAN_POINT('Ctrl Pts',(1.85948367088837,1.,-0.17473525927603));
#32106=CARTESIAN_POINT('Ctrl Pts',(1.8489811319852,-1.,-0.173946627587732));
#32107=CARTESIAN_POINT('Ctrl Pts',(1.8489811319852,1.,-0.173946627587732));
#32108=CARTESIAN_POINT('Ctrl Pts',(1.83658380527692,-1.,-0.1728894428919));
#32109=CARTESIAN_POINT('Ctrl Pts',(1.83658380527692,1.,-0.1728894428919));
#32110=CARTESIAN_POINT('Ctrl Pts',(1.82215766811545,-1.,-0.171554770204119));
#32111=CARTESIAN_POINT('Ctrl Pts',(1.82215766811545,1.,-0.171554770204119));
#32112=CARTESIAN_POINT('Ctrl Pts',(1.80561530629706,-1.,-0.169936923904608));
#32113=CARTESIAN_POINT('Ctrl Pts',(1.80561530629706,1.,-0.169936923904608));
#32114=CARTESIAN_POINT('Ctrl Pts',(1.7869064998507,-1.,-0.168032772805197));
#32115=CARTESIAN_POINT('Ctrl Pts',(1.7869064998507,1.,-0.168032772805197));
#32116=CARTESIAN_POINT('Ctrl Pts',(1.77018771684844,-1.,-0.1662793551464));
#32117=CARTESIAN_POINT('Ctrl Pts',(1.77018771684844,1.,-0.1662793551464));
#32118=CARTESIAN_POINT('Ctrl Pts',(1.75666056638427,-1.,-0.164834765707159));
#32119=CARTESIAN_POINT('Ctrl Pts',(1.75666056638427,1.,-0.164834765707159));
#32120=CARTESIAN_POINT('Ctrl Pts',(1.7472034950333,-1.,-0.163814161002002));
#32121=CARTESIAN_POINT('Ctrl Pts',(1.7472034950333,1.,-0.163814161002002));
#32122=CARTESIAN_POINT('Ctrl Pts',(1.74236521665491,-1.,-0.163289472382896));
#32123=CARTESIAN_POINT('Ctrl Pts',(1.74236521665491,1.,-0.163289472382896));
#32124=CARTESIAN_POINT('',(2.19890268624765,1.,-0.0694764450219582));
#32125=CARTESIAN_POINT('Ctrl Pts',(2.19890268624765,1.,-0.0694764450219582));
#32126=CARTESIAN_POINT('Ctrl Pts',(2.19777582085423,1.,-0.0701143536325491));
#32127=CARTESIAN_POINT('Ctrl Pts',(2.19552129484002,1.,-0.0713863779526155));
#32128=CARTESIAN_POINT('Ctrl Pts',(2.19213712013662,1.,-0.0732830357306726));
#32129=CARTESIAN_POINT('Ctrl Pts',(2.1876201139953,1.,-0.0757891465836149));
#32130=CARTESIAN_POINT('Ctrl Pts',(2.18196589448887,1.,-0.0788837727685244));
#32131=CARTESIAN_POINT('Ctrl Pts',(2.176303712113,1.,-0.0819402680872767));
#32132=CARTESIAN_POINT('Ctrl Pts',(2.17063357870952,1.,-0.0849584620835374));
#32133=CARTESIAN_POINT('Ctrl Pts',(2.16495552645014,1.,-0.0879381291386924));
#32134=CARTESIAN_POINT('Ctrl Pts',(2.15926961544516,1.,-0.0908789888107267));
#32135=CARTESIAN_POINT('Ctrl Pts',(2.1535759397817,1.,-0.0937807218867645));
#32136=CARTESIAN_POINT('Ctrl Pts',(2.14787463531795,1.,-0.096642985230546));
#32137=CARTESIAN_POINT('Ctrl Pts',(2.14216588396025,1.,-0.0994654261990917));
#32138=CARTESIAN_POINT('Ctrl Pts',(2.13644992667165,1.,-0.102247700556101));
#32139=CARTESIAN_POINT('Ctrl Pts',(2.13072704887293,1.,-0.10498947915274));
#32140=CARTESIAN_POINT('Ctrl Pts',(2.12499752307,1.,-0.10769043523109));
#32141=CARTESIAN_POINT('Ctrl Pts',(2.11926155590865,1.,-0.110350236135025));
#32142=CARTESIAN_POINT('Ctrl Pts',(2.11351924490306,1.,-0.112968534419737));
#32143=CARTESIAN_POINT('Ctrl Pts',(2.10777050261309,1.,-0.115544957687927));
#32144=CARTESIAN_POINT('Ctrl Pts',(2.102015121329,1.,-0.118079107988356));
#32145=CARTESIAN_POINT('Ctrl Pts',(2.0962529286773,1.,-0.120570567965122));
#32146=CARTESIAN_POINT('Ctrl Pts',(2.09048392424825,1.,-0.123018905621083));
#32147=CARTESIAN_POINT('Ctrl Pts',(2.08470840653643,1.,-0.125423679412062));
#32148=CARTESIAN_POINT('Ctrl Pts',(2.07892715110987,1.,-0.12778444527612));
#32149=CARTESIAN_POINT('Ctrl Pts',(2.07314114713063,1.,-0.130100748328404));
#32150=CARTESIAN_POINT('Ctrl Pts',(2.06735123910326,1.,-0.132372111547711));
#32151=CARTESIAN_POINT('Ctrl Pts',(2.06155781517842,1.,-0.134598026192106));
#32152=CARTESIAN_POINT('Ctrl Pts',(2.05576044414264,1.,-0.136777941218044));
#32153=CARTESIAN_POINT('Ctrl Pts',(2.04995762001328,1.,-0.138911255368966));
#32154=CARTESIAN_POINT('Ctrl Pts',(2.04414757947916,1.,-0.140997332152546));
#32155=CARTESIAN_POINT('Ctrl Pts',(2.03832911025912,1.,-0.143035515058209));
#32156=CARTESIAN_POINT('Ctrl Pts',(2.03250223739942,1.,-0.145025140186058));
#32157=CARTESIAN_POINT('Ctrl Pts',(2.02666926182017,1.,-0.146965557332583));
#32158=CARTESIAN_POINT('Ctrl Pts',(2.02083464969894,1.,-0.148856124775337));
#32159=CARTESIAN_POINT('Ctrl Pts',(2.01500291940238,1.,-0.150696157673078));
#32160=CARTESIAN_POINT('Ctrl Pts',(2.00917680318424,1.,-0.15248488362145));
#32161=CARTESIAN_POINT('Ctrl Pts',(2.00335565310543,1.,-0.154221403049722));
#32162=CARTESIAN_POINT('Ctrl Pts',(1.99753284771497,1.,-0.155904629548784));
#32163=CARTESIAN_POINT('Ctrl Pts',(1.99169810931908,1.,-0.157533331459227));
#32164=CARTESIAN_POINT('Ctrl Pts',(1.98584238283292,1.,-0.159106226437299));
#32165=CARTESIAN_POINT('Ctrl Pts',(1.97996195437559,1.,-0.160622060784611));
#32166=CARTESIAN_POINT('Ctrl Pts',(1.97406280235188,1.,-0.162079693556289));
#32167=CARTESIAN_POINT('Ctrl Pts',(1.96816512677967,1.,-0.163478185457734));
#32168=CARTESIAN_POINT('Ctrl Pts',(1.96229379940136,1.,-0.164816568920269));
#32169=CARTESIAN_POINT('Ctrl Pts',(1.9564675971873,1.,-0.166093592002813));
#32170=CARTESIAN_POINT('Ctrl Pts',(1.95069027794294,1.,-0.167307501784476));
#32171=CARTESIAN_POINT('Ctrl Pts',(1.94493757756931,1.,-0.168455741607556));
#32172=CARTESIAN_POINT('Ctrl Pts',(1.93915639211581,1.,-0.169534904817491));
#32173=CARTESIAN_POINT('Ctrl Pts',(1.93329183155539,1.,-0.170541253116202));
#32174=CARTESIAN_POINT('Ctrl Pts',(1.92731093582036,1.,-0.171471191532988));
#32175=CARTESIAN_POINT('Ctrl Pts',(1.9212233439798,1.,-0.172321621259514));
#32176=CARTESIAN_POINT('Ctrl Pts',(1.91511429159527,1.,-0.173090695383496));
#32177=CARTESIAN_POINT('Ctrl Pts',(1.90911693975267,1.,-0.173776635257817));
#32178=CARTESIAN_POINT('Ctrl Pts',(1.90335253862834,1.,-0.174375518661085));
#32179=CARTESIAN_POINT('Ctrl Pts',(1.89788101117132,1.,-0.174879405091263));
#32180=CARTESIAN_POINT('Ctrl Pts',(1.892646301985,1.,-0.175274276190844));
#32181=CARTESIAN_POINT('Ctrl Pts',(1.88742606273259,1.,-0.175538155840648));
#32182=CARTESIAN_POINT('Ctrl Pts',(1.88188663145367,1.,-0.175644148889699));
#32183=CARTESIAN_POINT('Ctrl Pts',(1.87563767773588,1.,-0.175563480746485));
#32184=CARTESIAN_POINT('Ctrl Pts',(1.86828349694799,1.,-0.175268337590758));
#32185=CARTESIAN_POINT('Ctrl Pts',(1.85948367088837,1.,-0.17473525927603));
#32186=CARTESIAN_POINT('Ctrl Pts',(1.8489811319852,1.,-0.173946627587732));
#32187=CARTESIAN_POINT('Ctrl Pts',(1.83658380527692,1.,-0.1728894428919));
#32188=CARTESIAN_POINT('Ctrl Pts',(1.82215766811545,1.,-0.171554770204119));
#32189=CARTESIAN_POINT('Ctrl Pts',(1.80561530629706,1.,-0.169936923904608));
#32190=CARTESIAN_POINT('Ctrl Pts',(1.7869064998507,1.,-0.168032772805197));
#32191=CARTESIAN_POINT('Ctrl Pts',(1.77018771684844,1.,-0.1662793551464));
#32192=CARTESIAN_POINT('Ctrl Pts',(1.75666056638427,1.,-0.164834765707159));
#32193=CARTESIAN_POINT('Ctrl Pts',(1.7472034950333,1.,-0.163814161002002));
#32194=CARTESIAN_POINT('Ctrl Pts',(1.74236521665491,1.,-0.163289472382896));
#32195=CARTESIAN_POINT('',(2.19890268624765,0.,-0.0694764450219582));
#32196=CARTESIAN_POINT('Origin',(2.19890268624765,0.,0.0694764450219582));
#32197=CARTESIAN_POINT('',(2.19890268624765,1.,0.0694764450219582));
#32198=CARTESIAN_POINT('',(2.19890268624765,1.,-0.0694764450219582));
#32199=CARTESIAN_POINT('',(2.19890268624765,0.,0.0694764450219582));
#32200=CARTESIAN_POINT('Ctrl Pts',(1.74236521665491,-1.,0.163289472382896));
#32201=CARTESIAN_POINT('Ctrl Pts',(1.74236521665491,1.,0.163289472382896));
#32202=CARTESIAN_POINT('Ctrl Pts',(1.74720349503904,-1.,0.163814161002474));
#32203=CARTESIAN_POINT('Ctrl Pts',(1.74720349503904,1.,0.163814161002474));
#32204=CARTESIAN_POINT('Ctrl Pts',(1.75666056640041,-1.,0.164834765708484));
#32205=CARTESIAN_POINT('Ctrl Pts',(1.75666056640041,1.,0.164834765708484));
#32206=CARTESIAN_POINT('Ctrl Pts',(1.77018771687692,-1.,0.166279355148738));
#32207=CARTESIAN_POINT('Ctrl Pts',(1.77018771687692,1.,0.166279355148738));
#32208=CARTESIAN_POINT('Ctrl Pts',(1.78690649988931,-1.,0.16803277280837));
#32209=CARTESIAN_POINT('Ctrl Pts',(1.78690649988931,1.,0.16803277280837));
#32210=CARTESIAN_POINT('Ctrl Pts',(1.80561530633924,-1.,0.169936923908078));
#32211=CARTESIAN_POINT('Ctrl Pts',(1.80561530633924,1.,0.169936923908078));
#32212=CARTESIAN_POINT('Ctrl Pts',(1.82215766815414,-1.,0.171554770207306));
#32213=CARTESIAN_POINT('Ctrl Pts',(1.82215766815414,1.,0.171554770207306));
#32214=CARTESIAN_POINT('Ctrl Pts',(1.83658380530747,-1.,0.17288944289442));
#32215=CARTESIAN_POINT('Ctrl Pts',(1.83658380530747,1.,0.17288944289442));
#32216=CARTESIAN_POINT('Ctrl Pts',(1.84898113200543,-1.,0.173946627589401));
#32217=CARTESIAN_POINT('Ctrl Pts',(1.84898113200543,1.,0.173946627589401));
#32218=CARTESIAN_POINT('Ctrl Pts',(1.85948367089838,-1.,0.174735259276856));
#32219=CARTESIAN_POINT('Ctrl Pts',(1.85948367089838,1.,0.174735259276856));
#32220=CARTESIAN_POINT('Ctrl Pts',(1.86828349694972,-1.,0.1752683375909));
#32221=CARTESIAN_POINT('Ctrl Pts',(1.86828349694972,1.,0.1752683375909));
#32222=CARTESIAN_POINT('Ctrl Pts',(1.87563767773249,-1.,0.175563480746205));
#32223=CARTESIAN_POINT('Ctrl Pts',(1.87563767773249,1.,0.175563480746205));
#32224=CARTESIAN_POINT('Ctrl Pts',(1.88188663144846,-1.,0.175644148889271));
#32225=CARTESIAN_POINT('Ctrl Pts',(1.88188663144846,1.,0.175644148889271));
#32226=CARTESIAN_POINT('Ctrl Pts',(1.88742606272818,-1.,0.175538155840286));
#32227=CARTESIAN_POINT('Ctrl Pts',(1.88742606272818,1.,0.175538155840286));
#32228=CARTESIAN_POINT('Ctrl Pts',(1.89264630198279,-1.,0.175274276190664));
#32229=CARTESIAN_POINT('Ctrl Pts',(1.89264630198279,1.,0.175274276190664));
#32230=CARTESIAN_POINT('Ctrl Pts',(1.89788101117148,-1.,0.174879405091277));
#32231=CARTESIAN_POINT('Ctrl Pts',(1.89788101117148,1.,0.174879405091277));
#32232=CARTESIAN_POINT('Ctrl Pts',(1.90335253863003,-1.,0.174375518661222));
#32233=CARTESIAN_POINT('Ctrl Pts',(1.90335253863003,1.,0.174375518661222));
#32234=CARTESIAN_POINT('Ctrl Pts',(1.90911693975475,-1.,0.173776635257983));
#32235=CARTESIAN_POINT('Ctrl Pts',(1.90911693975475,1.,0.173776635257983));
#32236=CARTESIAN_POINT('Ctrl Pts',(1.91511429159681,-1.,0.173090695383619));
#32237=CARTESIAN_POINT('Ctrl Pts',(1.91511429159681,1.,0.173090695383619));
#32238=CARTESIAN_POINT('Ctrl Pts',(1.92122334398034,-1.,0.172321621259556));
#32239=CARTESIAN_POINT('Ctrl Pts',(1.92122334398034,1.,0.172321621259556));
#32240=CARTESIAN_POINT('Ctrl Pts',(1.92731093582,-1.,0.17147119153296));
#32241=CARTESIAN_POINT('Ctrl Pts',(1.92731093582,1.,0.17147119153296));
#32242=CARTESIAN_POINT('Ctrl Pts',(1.93329183155455,-1.,0.170541253116136));
#32243=CARTESIAN_POINT('Ctrl Pts',(1.93329183155455,1.,0.170541253116136));
#32244=CARTESIAN_POINT('Ctrl Pts',(1.93915639211497,-1.,0.169534904817425));
#32245=CARTESIAN_POINT('Ctrl Pts',(1.93915639211497,1.,0.169534904817425));
#32246=CARTESIAN_POINT('Ctrl Pts',(1.94493757756879,-1.,0.168455741607515));
#32247=CARTESIAN_POINT('Ctrl Pts',(1.94493757756879,1.,0.168455741607515));
#32248=CARTESIAN_POINT('Ctrl Pts',(1.95069027794286,-1.,0.167307501784469));
#32249=CARTESIAN_POINT('Ctrl Pts',(1.95069027794286,1.,0.167307501784469));
#32250=CARTESIAN_POINT('Ctrl Pts',(1.95646759718755,-1.,0.166093592002832));
#32251=CARTESIAN_POINT('Ctrl Pts',(1.95646759718755,1.,0.166093592002832));
#32252=CARTESIAN_POINT('Ctrl Pts',(1.96229379940174,-1.,0.1648165689203));
#32253=CARTESIAN_POINT('Ctrl Pts',(1.96229379940174,1.,0.1648165689203));
#32254=CARTESIAN_POINT('Ctrl Pts',(1.96816512678,-1.,0.16347818545776));
#32255=CARTESIAN_POINT('Ctrl Pts',(1.96816512678,1.,0.16347818545776));
#32256=CARTESIAN_POINT('Ctrl Pts',(1.97406280235204,-1.,0.162079693556302));
#32257=CARTESIAN_POINT('Ctrl Pts',(1.97406280235204,1.,0.162079693556302));
#32258=CARTESIAN_POINT('Ctrl Pts',(1.97996195437557,-1.,0.16062206078461));
#32259=CARTESIAN_POINT('Ctrl Pts',(1.97996195437557,1.,0.16062206078461));
#32260=CARTESIAN_POINT('Ctrl Pts',(1.98584238283279,-1.,0.159106226437288));
#32261=CARTESIAN_POINT('Ctrl Pts',(1.98584238283279,1.,0.159106226437288));
#32262=CARTESIAN_POINT('Ctrl Pts',(1.99169810931893,-1.,0.157533331459215));
#32263=CARTESIAN_POINT('Ctrl Pts',(1.99169810931893,1.,0.157533331459215));
#32264=CARTESIAN_POINT('Ctrl Pts',(1.99753284771487,-1.,0.155904629548774));
#32265=CARTESIAN_POINT('Ctrl Pts',(1.99753284771487,1.,0.155904629548774));
#32266=CARTESIAN_POINT('Ctrl Pts',(2.00335565310539,-1.,0.154221403049719));
#32267=CARTESIAN_POINT('Ctrl Pts',(2.00335565310539,1.,0.154221403049719));
#32268=CARTESIAN_POINT('Ctrl Pts',(2.00917680318426,-1.,0.152484883621452));
#32269=CARTESIAN_POINT('Ctrl Pts',(2.00917680318426,1.,0.152484883621452));
#32270=CARTESIAN_POINT('Ctrl Pts',(2.01500291940243,-1.,0.150696157673084));
#32271=CARTESIAN_POINT('Ctrl Pts',(2.01500291940243,1.,0.150696157673084));
#32272=CARTESIAN_POINT('Ctrl Pts',(2.02083464969897,-1.,0.148856124775342));
#32273=CARTESIAN_POINT('Ctrl Pts',(2.02083464969897,1.,0.148856124775342));
#32274=CARTESIAN_POINT('Ctrl Pts',(2.02666926182017,-1.,0.146965557332586));
#32275=CARTESIAN_POINT('Ctrl Pts',(2.02666926182017,1.,0.146965557332586));
#32276=CARTESIAN_POINT('Ctrl Pts',(2.03250223739941,-1.,0.145025140186058));
#32277=CARTESIAN_POINT('Ctrl Pts',(2.03250223739941,1.,0.145025140186058));
#32278=CARTESIAN_POINT('Ctrl Pts',(2.03832911025913,-1.,0.143035515058208));
#32279=CARTESIAN_POINT('Ctrl Pts',(2.03832911025913,1.,0.143035515058208));
#32280=CARTESIAN_POINT('Ctrl Pts',(2.04414757947919,-1.,0.140997332152545));
#32281=CARTESIAN_POINT('Ctrl Pts',(2.04414757947919,1.,0.140997332152545));
#32282=CARTESIAN_POINT('Ctrl Pts',(2.04995762001333,-1.,0.138911255368966));
#32283=CARTESIAN_POINT('Ctrl Pts',(2.04995762001333,1.,0.138911255368966));
#32284=CARTESIAN_POINT('Ctrl Pts',(2.0557604441427,-1.,0.136777941218044));
#32285=CARTESIAN_POINT('Ctrl Pts',(2.0557604441427,1.,0.136777941218044));
#32286=CARTESIAN_POINT('Ctrl Pts',(2.06155781517844,-1.,0.134598026192107));
#32287=CARTESIAN_POINT('Ctrl Pts',(2.06155781517844,1.,0.134598026192107));
#32288=CARTESIAN_POINT('Ctrl Pts',(2.06735123910319,-1.,0.132372111547709));
#32289=CARTESIAN_POINT('Ctrl Pts',(2.06735123910319,1.,0.132372111547709));
#32290=CARTESIAN_POINT('Ctrl Pts',(2.07314114713047,-1.,0.1301007483284));
#32291=CARTESIAN_POINT('Ctrl Pts',(2.07314114713047,1.,0.1301007483284));
#32292=CARTESIAN_POINT('Ctrl Pts',(2.07892715110967,-1.,0.127784445276116));
#32293=CARTESIAN_POINT('Ctrl Pts',(2.07892715110967,1.,0.127784445276116));
#32294=CARTESIAN_POINT('Ctrl Pts',(2.08470840653628,-1.,0.125423679412058));
#32295=CARTESIAN_POINT('Ctrl Pts',(2.08470840653628,1.,0.125423679412058));
#32296=CARTESIAN_POINT('Ctrl Pts',(2.09048392424826,-1.,0.123018905621083));
#32297=CARTESIAN_POINT('Ctrl Pts',(2.09048392424826,1.,0.123018905621083));
#32298=CARTESIAN_POINT('Ctrl Pts',(2.09625292867756,-1.,0.120570567965129));
#32299=CARTESIAN_POINT('Ctrl Pts',(2.09625292867756,1.,0.120570567965129));
#32300=CARTESIAN_POINT('Ctrl Pts',(2.10201512132945,-1.,0.118079107988368));
#32301=CARTESIAN_POINT('Ctrl Pts',(2.10201512132945,1.,0.118079107988368));
#32302=CARTESIAN_POINT('Ctrl Pts',(2.10777050261359,-1.,0.11554495768794));
#32303=CARTESIAN_POINT('Ctrl Pts',(2.10777050261359,1.,0.11554495768794));
#32304=CARTESIAN_POINT('Ctrl Pts',(2.11351924490335,-1.,0.112968534419746));
#32305=CARTESIAN_POINT('Ctrl Pts',(2.11351924490335,1.,0.112968534419746));
#32306=CARTESIAN_POINT('Ctrl Pts',(2.11926155590849,-1.,0.11035023613502));
#32307=CARTESIAN_POINT('Ctrl Pts',(2.11926155590849,1.,0.11035023613502));
#32308=CARTESIAN_POINT('Ctrl Pts',(2.12499752306927,-1.,0.107690435231068));
#32309=CARTESIAN_POINT('Ctrl Pts',(2.12499752306927,1.,0.107690435231068));
#32310=CARTESIAN_POINT('Ctrl Pts',(2.1307270488718,-1.,0.104989479152703));
#32311=CARTESIAN_POINT('Ctrl Pts',(2.1307270488718,1.,0.104989479152703));
#32312=CARTESIAN_POINT('Ctrl Pts',(2.13644992667052,-1.,0.102247700556063));
#32313=CARTESIAN_POINT('Ctrl Pts',(2.13644992667052,1.,0.102247700556063));
#32314=CARTESIAN_POINT('Ctrl Pts',(2.14216588395974,-1.,0.0994654261990741));
#32315=CARTESIAN_POINT('Ctrl Pts',(2.14216588395974,1.,0.0994654261990741));
#32316=CARTESIAN_POINT('Ctrl Pts',(2.14787463531864,-1.,0.0966429852305688));
#32317=CARTESIAN_POINT('Ctrl Pts',(2.14787463531864,1.,0.0966429852305688));
#32318=CARTESIAN_POINT('Ctrl Pts',(2.15357593978377,-1.,0.0937807218868344));
#32319=CARTESIAN_POINT('Ctrl Pts',(2.15357593978377,1.,0.0937807218868344));
#32320=CARTESIAN_POINT('Ctrl Pts',(2.15926961544808,-1.,0.0908789888108265));
#32321=CARTESIAN_POINT('Ctrl Pts',(2.15926961544808,1.,0.0908789888108265));
#32322=CARTESIAN_POINT('Ctrl Pts',(2.16495552645275,-1.,0.0879381291387821));
#32323=CARTESIAN_POINT('Ctrl Pts',(2.16495552645275,1.,0.0879381291387821));
#32324=CARTESIAN_POINT('Ctrl Pts',(2.17063357871031,-1.,0.0849584620835642));
#32325=CARTESIAN_POINT('Ctrl Pts',(2.17063357871031,1.,0.0849584620835642));
#32326=CARTESIAN_POINT('Ctrl Pts',(2.1763037121106,-1.,0.0819402680871938));
#32327=CARTESIAN_POINT('Ctrl Pts',(2.1763037121106,1.,0.0819402680871938));
#32328=CARTESIAN_POINT('Ctrl Pts',(2.18196589448304,-1.,0.0788837727683226));
#32329=CARTESIAN_POINT('Ctrl Pts',(2.18196589448304,1.,0.0788837727683226));
#32330=CARTESIAN_POINT('Ctrl Pts',(2.1876201139874,-1.,0.075789146583341));
#32331=CARTESIAN_POINT('Ctrl Pts',(2.1876201139874,1.,0.075789146583341));
#32332=CARTESIAN_POINT('Ctrl Pts',(2.19213712012956,-1.,0.0732830357304275));
#32333=CARTESIAN_POINT('Ctrl Pts',(2.19213712012956,1.,0.0732830357304275));
#32334=CARTESIAN_POINT('Ctrl Pts',(2.19552129483562,-1.,0.0713863779524626));
#32335=CARTESIAN_POINT('Ctrl Pts',(2.19552129483562,1.,0.0713863779524626));
#32336=CARTESIAN_POINT('Ctrl Pts',(2.19777582085261,-1.,0.0701143536324925));
#32337=CARTESIAN_POINT('Ctrl Pts',(2.19777582085261,1.,0.0701143536324925));
#32338=CARTESIAN_POINT('Ctrl Pts',(2.19890268624765,-1.,0.0694764450219582));
#32339=CARTESIAN_POINT('Ctrl Pts',(2.19890268624765,1.,0.0694764450219582));
#32340=CARTESIAN_POINT('',(1.74236521665491,1.,0.163289472382896));
#32341=CARTESIAN_POINT('Ctrl Pts',(1.74236521665491,1.,0.163289472382896));
#32342=CARTESIAN_POINT('Ctrl Pts',(1.74720349503904,1.,0.163814161002474));
#32343=CARTESIAN_POINT('Ctrl Pts',(1.75666056640041,1.,0.164834765708484));
#32344=CARTESIAN_POINT('Ctrl Pts',(1.77018771687692,1.,0.166279355148738));
#32345=CARTESIAN_POINT('Ctrl Pts',(1.78690649988931,1.,0.16803277280837));
#32346=CARTESIAN_POINT('Ctrl Pts',(1.80561530633924,1.,0.169936923908078));
#32347=CARTESIAN_POINT('Ctrl Pts',(1.82215766815414,1.,0.171554770207306));
#32348=CARTESIAN_POINT('Ctrl Pts',(1.83658380530747,1.,0.17288944289442));
#32349=CARTESIAN_POINT('Ctrl Pts',(1.84898113200543,1.,0.173946627589401));
#32350=CARTESIAN_POINT('Ctrl Pts',(1.85948367089838,1.,0.174735259276856));
#32351=CARTESIAN_POINT('Ctrl Pts',(1.86828349694972,1.,0.1752683375909));
#32352=CARTESIAN_POINT('Ctrl Pts',(1.87563767773249,1.,0.175563480746205));
#32353=CARTESIAN_POINT('Ctrl Pts',(1.88188663144846,1.,0.175644148889271));
#32354=CARTESIAN_POINT('Ctrl Pts',(1.88742606272818,1.,0.175538155840286));
#32355=CARTESIAN_POINT('Ctrl Pts',(1.89264630198279,1.,0.175274276190664));
#32356=CARTESIAN_POINT('Ctrl Pts',(1.89788101117148,1.,0.174879405091277));
#32357=CARTESIAN_POINT('Ctrl Pts',(1.90335253863003,1.,0.174375518661222));
#32358=CARTESIAN_POINT('Ctrl Pts',(1.90911693975475,1.,0.173776635257983));
#32359=CARTESIAN_POINT('Ctrl Pts',(1.91511429159681,1.,0.173090695383619));
#32360=CARTESIAN_POINT('Ctrl Pts',(1.92122334398034,1.,0.172321621259556));
#32361=CARTESIAN_POINT('Ctrl Pts',(1.92731093582,1.,0.17147119153296));
#32362=CARTESIAN_POINT('Ctrl Pts',(1.93329183155455,1.,0.170541253116136));
#32363=CARTESIAN_POINT('Ctrl Pts',(1.93915639211497,1.,0.169534904817425));
#32364=CARTESIAN_POINT('Ctrl Pts',(1.94493757756879,1.,0.168455741607515));
#32365=CARTESIAN_POINT('Ctrl Pts',(1.95069027794286,1.,0.167307501784469));
#32366=CARTESIAN_POINT('Ctrl Pts',(1.95646759718755,1.,0.166093592002832));
#32367=CARTESIAN_POINT('Ctrl Pts',(1.96229379940174,1.,0.1648165689203));
#32368=CARTESIAN_POINT('Ctrl Pts',(1.96816512678,1.,0.16347818545776));
#32369=CARTESIAN_POINT('Ctrl Pts',(1.97406280235204,1.,0.162079693556302));
#32370=CARTESIAN_POINT('Ctrl Pts',(1.97996195437557,1.,0.16062206078461));
#32371=CARTESIAN_POINT('Ctrl Pts',(1.98584238283279,1.,0.159106226437288));
#32372=CARTESIAN_POINT('Ctrl Pts',(1.99169810931893,1.,0.157533331459215));
#32373=CARTESIAN_POINT('Ctrl Pts',(1.99753284771487,1.,0.155904629548774));
#32374=CARTESIAN_POINT('Ctrl Pts',(2.00335565310539,1.,0.154221403049719));
#32375=CARTESIAN_POINT('Ctrl Pts',(2.00917680318426,1.,0.152484883621452));
#32376=CARTESIAN_POINT('Ctrl Pts',(2.01500291940243,1.,0.150696157673084));
#32377=CARTESIAN_POINT('Ctrl Pts',(2.02083464969897,1.,0.148856124775342));
#32378=CARTESIAN_POINT('Ctrl Pts',(2.02666926182017,1.,0.146965557332586));
#32379=CARTESIAN_POINT('Ctrl Pts',(2.03250223739941,1.,0.145025140186058));
#32380=CARTESIAN_POINT('Ctrl Pts',(2.03832911025913,1.,0.143035515058208));
#32381=CARTESIAN_POINT('Ctrl Pts',(2.04414757947919,1.,0.140997332152545));
#32382=CARTESIAN_POINT('Ctrl Pts',(2.04995762001333,1.,0.138911255368966));
#32383=CARTESIAN_POINT('Ctrl Pts',(2.0557604441427,1.,0.136777941218044));
#32384=CARTESIAN_POINT('Ctrl Pts',(2.06155781517844,1.,0.134598026192107));
#32385=CARTESIAN_POINT('Ctrl Pts',(2.06735123910319,1.,0.132372111547709));
#32386=CARTESIAN_POINT('Ctrl Pts',(2.07314114713047,1.,0.1301007483284));
#32387=CARTESIAN_POINT('Ctrl Pts',(2.07892715110967,1.,0.127784445276116));
#32388=CARTESIAN_POINT('Ctrl Pts',(2.08470840653628,1.,0.125423679412058));
#32389=CARTESIAN_POINT('Ctrl Pts',(2.09048392424826,1.,0.123018905621083));
#32390=CARTESIAN_POINT('Ctrl Pts',(2.09625292867756,1.,0.120570567965129));
#32391=CARTESIAN_POINT('Ctrl Pts',(2.10201512132945,1.,0.118079107988368));
#32392=CARTESIAN_POINT('Ctrl Pts',(2.10777050261359,1.,0.11554495768794));
#32393=CARTESIAN_POINT('Ctrl Pts',(2.11351924490335,1.,0.112968534419746));
#32394=CARTESIAN_POINT('Ctrl Pts',(2.11926155590849,1.,0.11035023613502));
#32395=CARTESIAN_POINT('Ctrl Pts',(2.12499752306927,1.,0.107690435231068));
#32396=CARTESIAN_POINT('Ctrl Pts',(2.1307270488718,1.,0.104989479152703));
#32397=CARTESIAN_POINT('Ctrl Pts',(2.13644992667052,1.,0.102247700556063));
#32398=CARTESIAN_POINT('Ctrl Pts',(2.14216588395974,1.,0.0994654261990741));
#32399=CARTESIAN_POINT('Ctrl Pts',(2.14787463531864,1.,0.0966429852305688));
#32400=CARTESIAN_POINT('Ctrl Pts',(2.15357593978377,1.,0.0937807218868344));
#32401=CARTESIAN_POINT('Ctrl Pts',(2.15926961544808,1.,0.0908789888108265));
#32402=CARTESIAN_POINT('Ctrl Pts',(2.16495552645275,1.,0.0879381291387821));
#32403=CARTESIAN_POINT('Ctrl Pts',(2.17063357871031,1.,0.0849584620835642));
#32404=CARTESIAN_POINT('Ctrl Pts',(2.1763037121106,1.,0.0819402680871938));
#32405=CARTESIAN_POINT('Ctrl Pts',(2.18196589448304,1.,0.0788837727683226));
#32406=CARTESIAN_POINT('Ctrl Pts',(2.1876201139874,1.,0.075789146583341));
#32407=CARTESIAN_POINT('Ctrl Pts',(2.19213712012956,1.,0.0732830357304275));
#32408=CARTESIAN_POINT('Ctrl Pts',(2.19552129483562,1.,0.0713863779524626));
#32409=CARTESIAN_POINT('Ctrl Pts',(2.19777582085261,1.,0.0701143536324925));
#32410=CARTESIAN_POINT('Ctrl Pts',(2.19890268624765,1.,0.0694764450219582));
#32411=CARTESIAN_POINT('',(1.74236521665491,0.,0.163289472382896));
#32412=CARTESIAN_POINT('Origin',(0.,1.,0.));
#32413=CARTESIAN_POINT('Origin',(0.,1.,0.));
#32414=CARTESIAN_POINT('Origin',(0.,0.,0.));
#32696=UNCERTAINTY_MEASURE_WITH_UNIT(LENGTH_MEASURE(0.001),#32752,
'DISTANCE_ACCURACY_VALUE',
'Maximum model space distance between geometric entities at asserted c
onnectivities');
#32702=UNCERTAINTY_MEASURE_WITH_UNIT(LENGTH_MEASURE(0.001),#32752,
'DISTANCE_ACCURACY_VALUE',
'Maximum model space distance between geometric entities at asserted c
onnectivities');
#32745=(
GEOMETRIC_REPRESENTATION_CONTEXT(3)
GLOBAL_UNCERTAINTY_ASSIGNED_CONTEXT((#32696))
GLOBAL_UNIT_ASSIGNED_CONTEXT((#32752,#32754,#32755))
REPRESENTATION_CONTEXT('','3D')
);
#32751=(
GEOMETRIC_REPRESENTATION_CONTEXT(3)
GLOBAL_UNCERTAINTY_ASSIGNED_CONTEXT((#32702))
GLOBAL_UNIT_ASSIGNED_CONTEXT((#32752,#32754,#32755))
REPRESENTATION_CONTEXT('','3D')
);
#32752=(
LENGTH_UNIT()
NAMED_UNIT(*)
SI_UNIT(.CENTI.,.METRE.)
);
#32754=(
NAMED_UNIT(*)
PLANE_ANGLE_UNIT()
SI_UNIT($,.RADIAN.)
);
#32755=(
NAMED_UNIT(*)
SI_UNIT($,.STERADIAN.)
SOLID_ANGLE_UNIT()
);
#32798=SHAPE_DEFINITION_REPRESENTATION(#32855,#32971);
#32855=PRODUCT_DEFINITION_SHAPE('',$,#33020);
#32971=SHAPE_REPRESENTATION('',(#13923),#32745);
#32977=PRODUCT_DEFINITION_CONTEXT('part definition',#33123,'design');
#33020=PRODUCT_DEFINITION('Spur Gear - Module 2, 20 Teeth, 12 mm Bore',
'Spur Gear - Module 2, 20 Teeth, 12 mm Bore',#33068,#32977);
#33068=PRODUCT_DEFINITION_FORMATION('',$,#33167);
#33123=APPLICATION_CONTEXT(
'Core Data for Automotive Mechanical Design Process');
#33124=PRODUCT_CONTEXT('part definition',#33123,'mechanical');
#33167=PRODUCT('Spur Gear - Module 2, 20 Teeth, 12 mm Bore',
'Spur Gear - Module 2, 20 Teeth, 12 mm Bore',
'Spur Gear - Module 2, 20 Teeth, 12 mm Bore',(#33124));
#33250=COLOUR_RGB('Off White',0.89,0.88,0.83);
#33251=FILL_AREA_STYLE_COLOUR('',#33250);
#33252=FILL_AREA_STYLE('',(#33251));
#33253=SURFACE_STYLE_FILL_AREA(#33252);
#33254=SURFACE_SIDE_STYLE('',(#33253));
#33255=SURFACE_STYLE_USAGE(.BOTH.,#33254);
#33256=PRESENTATION_STYLE_ASSIGNMENT((#33255));
ENDSEC;
END-ISO-10303-21;
